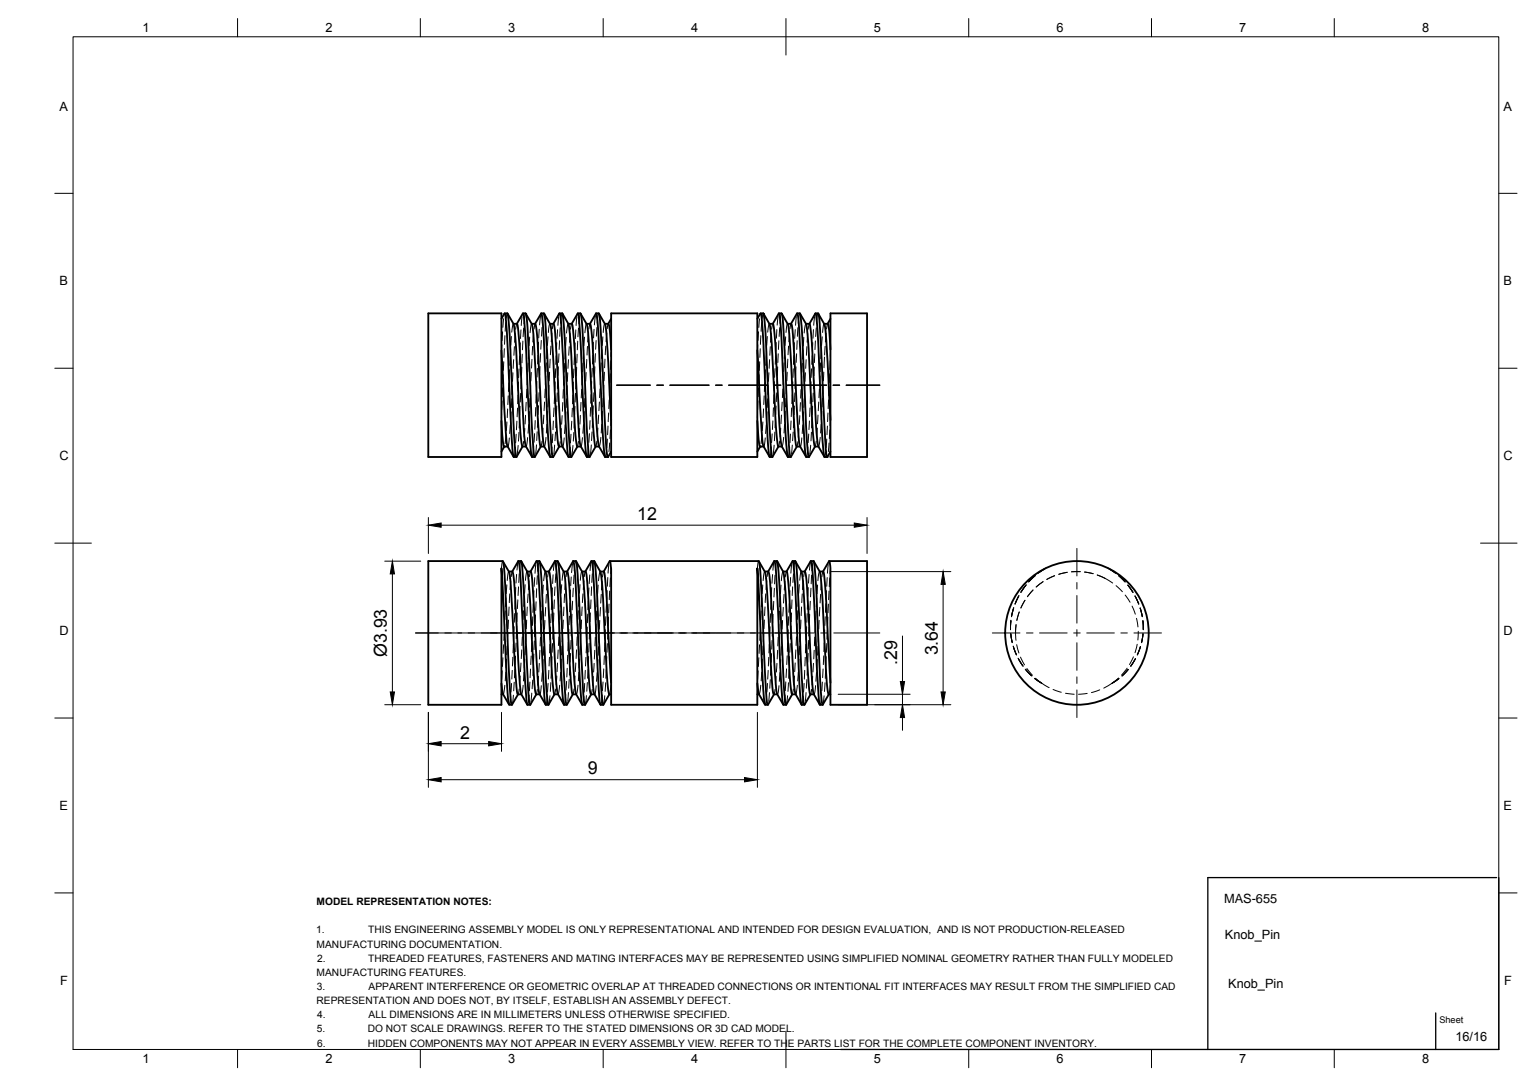
ISO-10303-21;
HEADER;
FILE_DESCRIPTION((''),'2;1');
FILE_NAME('Knob_Pin.step','2026-10-09T11:34:15-07:00',(''),(''),'','','');
FILE_SCHEMA (('AUTOMOTIVE_DESIGN { 1 0 10303 214 3 1 1 }'));
ENDSEC;
DATA;
#10=MECHANICAL_DESIGN_GEOMETRIC_PRESENTATION_REPRESENTATION('',(#648),#117170);
#606=SHAPE_REPRESENTATION_RELATIONSHIP('SRR','None',#117261,#627) ;
#627=ADVANCED_BREP_SHAPE_REPRESENTATION('',(#669),#117169) ;
#648=STYLED_ITEM('',(#117355),#669) ;
#669=MANIFOLD_SOLID_BREP('Body1',#49077) ;
#770=FACE_BOUND('',#17019,.T.) ;
#771=FACE_BOUND('',#17020,.T.) ;
#772=FACE_BOUND('',#17021,.T.) ;
#1697=B_SPLINE_CURVE_WITH_KNOTS('',3,(#109203,#109204,#109205,#109206,#109207,
#109208,#109209,#109210,#109211,#109212,#109213,#109214,#109215,#109216,
#109217,#109218,#109219,#109220,#109221,#109222,#109223,#109224,#109225,
#109226,#109227,#109228,#109229,#109230,#109231,#109232,#109233,#109234,
#109235,#109236,#109237,#109238,#109239,#109240,#109241,#109242,#109243,
#109244,#109245,#109246,#109247,#109248,#109249,#109250,#109251,#109252,
#109253,#109254,#109255,#109256,#109257,#109258,#109259,#109260,#109261,
#109262,#109263,#109264,#109265,#109266,#109267,#109268,#109269,#109270,
#109271,#109272,#109273,#109274,#109275,#109276,#109277,#109278,#109279,
#109280,#109281,#109282),.UNSPECIFIED.,.F.,.F.,(4,2,2,2,2,2,2,2,2,2,2,2,
2,2,2,2,2,2,2,2,2,2,2,2,2,2,2,2,2,2,2,2,2,2,2,2,2,2,2,4),(-0.552593410761711,
-0.5520841033493,-0.543414800045841,-0.530981645331462,-0.515682120379995,
-0.489011851192856,-0.475791475211459,-0.469800228676837,-0.464823585052418,
-0.456758200675436,-0.446117862199597,-0.412190397885134,-0.396445377902817,
-0.387356530724998,-0.378534621106888,-0.364686037892163,-0.330083411853553,
-0.312869588553632,-0.306676202327231,-0.301718040883505,-0.293987276238174,
-0.28400901338443,-0.255540175710082,-0.235962621045616,-0.226122570338451,
-0.217486499647387,-0.205608163506685,-0.191376706596845,-0.162958816002947,
-0.149015686282994,-0.143020064395438,-0.137940493423511,-0.129517498871141,
-0.118194060456811,-0.0767579974893125,-0.0659012890372971,-0.0573052858902992,
-0.0467033580009995,-0.0196389999660062,-0.00261625130652141),
 .UNSPECIFIED.) ;
#1698=B_SPLINE_CURVE_WITH_KNOTS('',3,(#109285,#109286,#109287,#109288,#109289,
#109290,#109291,#109292,#109293,#109294,#109295,#109296,#109297,#109298,
#109299,#109300,#109301,#109302,#109303,#109304,#109305,#109306,#109307,
#109308,#109309,#109310,#109311,#109312,#109313,#109314,#109315,#109316,
#109317,#109318,#109319,#109320,#109321,#109322,#109323,#109324,#109325,
#109326,#109327,#109328,#109329,#109330,#109331,#109332),.UNSPECIFIED.,
 .F.,.F.,(4,2,2,2,2,2,2,2,2,2,2,2,2,2,2,2,2,2,2,2,2,2,2,4),(-1.74388914172831,
-1.74010158624316,-1.73533493491195,-1.69713014187374,-1.68355997429145,
-1.67194962285965,-1.66271393068178,-1.65106169492588,-1.61630518110585,
-1.58993773929061,-1.58306967342475,-1.57816077380394,-1.57132637085491,
-1.54363126039316,-1.51548297073149,-1.50527675750718,-1.49695811956463,
-1.48648723066268,-1.44858943711612,-1.42603340225277,-1.41932565863014,
-1.41457975898413,-1.40826951094876,-1.40009241220142),.UNSPECIFIED.) ;
#1699=B_SPLINE_CURVE_WITH_KNOTS('',3,(#109337,#109338,#109339,#109340,#109341,
#109342,#109343,#109344,#109345,#109346,#109347,#109348,#109349,#109350,
#109351,#109352,#109353,#109354,#109355,#109356,#109357,#109358,#109359,
#109360,#109361,#109362,#109363,#109364,#109365,#109366,#109367,#109368,
#109369,#109370,#109371,#109372,#109373,#109374,#109375,#109376,#109377,
#109378,#109379,#109380,#109381,#109382,#109383,#109384,#109385,#109386,
#109387,#109388,#109389,#109390,#109391,#109392,#109393,#109394,#109395,
#109396,#109397,#109398,#109399,#109400,#109401,#109402,#109403,#109404,
#109405,#109406,#109407,#109408,#109409,#109410,#109411,#109412,#109413,
#109414,#109415,#109416,#109417,#109418,#109419,#109420,#109421,#109422,
#109423,#109424,#109425,#109426,#109427,#109428,#109429,#109430,#109431,
#109432,#109433,#109434,#109435,#109436,#109437,#109438,#109439,#109440,
#109441,#109442,#109443,#109444,#109445,#109446,#109447,#109448,#109449,
#109450,#109451,#109452,#109453,#109454,#109455,#109456,#109457,#109458,
#109459,#109460,#109461,#109462,#109463,#109464,#109465,#109466,#109467,
#109468,#109469,#109470,#109471,#109472,#109473,#109474,#109475,#109476),
 .UNSPECIFIED.,.F.,.F.,(4,2,2,2,2,2,2,2,2,2,2,2,2,2,2,2,2,2,2,2,2,2,2,2,
2,2,2,2,2,2,2,2,2,2,2,2,2,2,2,2,2,2,2,2,2,2,2,2,2,2,2,2,2,2,2,2,2,2,2,2,
2,2,2,2,2,2,2,2,2,4),(-1.60819476001236,-1.60157151108133,-1.57374993060186,
-1.54333520918712,-1.5330944628995,-1.52455732114626,-1.51368106490473,
-1.48363670371605,-1.45716775914122,-1.45034362080875,-1.44544941240374,
-1.43858684897259,-1.40293109993587,-1.38660840131381,-1.37365915712381,
-1.36493247672918,-1.35557163070149,-1.33795142758038,-1.30177252657126,
-1.29363751094972,-1.28694201653805,-1.28204551297269,-1.27504505146196,
-1.24750286398903,-1.21793991752278,-1.20732165243159,-1.1987959811487,
-1.18816616116487,-1.1535726711856,-1.1305629468268,-1.12379029329879,-1.11889461776859,
-1.11197522743769,-1.08352620940999,-1.05355243311613,-1.04333196199694,
-1.03479173415174,-1.02388438639545,-0.996280762100526,-0.97622121148834,
-0.964282134908163,-0.958700667916607,-0.953524190525165,-0.944167265791223,
-0.930858282226715,-0.891097096141751,-0.88060265191729,-0.872078959293447,
-0.861328341297288,-0.836209324457884,-0.803362711467678,-0.796962241119135,
-0.792056336516214,-0.784839695546787,-0.775791460713609,-0.753103628892537,
-0.728807187779854,-0.717955013186807,-0.709422378254332,-0.699000038493792,
-0.687312334031512,-0.663447018063261,-0.64163726390635,-0.634488912403423,
-0.629581096095425,-0.622988562285989,-0.615033268711227,-0.580749247858517,
-0.561627829423672,-0.552593410761711),.UNSPECIFIED.) ;
#1700=B_SPLINE_CURVE_WITH_KNOTS('',3,(#109477,#109478,#109479,#109480,#109481,
#109482,#109483,#109484,#109485,#109486,#109487,#109488,#109489,#109490,
#109491,#109492,#109493,#109494,#109495,#109496,#109497,#109498,#109499,
#109500,#109501,#109502,#109503,#109504,#109505,#109506,#109507,#109508,
#109509,#109510,#109511,#109512,#109513,#109514,#109515,#109516,#109517,
#109518,#109519,#109520,#109521,#109522,#109523,#109524,#109525,#109526,
#109527,#109528,#109529,#109530,#109531,#109532,#109533,#109534,#109535,
#109536,#109537,#109538,#109539,#109540,#109541,#109542,#109543,#109544,
#109545,#109546,#109547,#109548,#109549,#109550,#109551,#109552,#109553,
#109554,#109555,#109556,#109557,#109558,#109559,#109560,#109561,#109562,
#109563,#109564,#109565,#109566,#109567,#109568,#109569,#109570,#109571,
#109572,#109573,#109574,#109575,#109576,#109577,#109578,#109579,#109580,
#109581,#109582,#109583,#109584,#109585,#109586,#109587,#109588,#109589,
#109590,#109591,#109592,#109593,#109594,#109595,#109596,#109597,#109598,
#109599,#109600,#109601,#109602,#109603,#109604,#109605,#109606,#109607,
#109608,#109609,#109610,#109611,#109612,#109613,#109614,#109615,#109616,
#109617,#109618,#109619,#109620),.UNSPECIFIED.,.F.,.F.,(4,2,2,2,2,2,2,2,
2,2,2,2,2,2,2,2,2,2,2,2,2,2,2,2,2,2,2,2,2,2,2,2,2,2,2,2,2,2,2,2,2,2,2,2,
2,2,2,2,2,2,2,2,2,2,2,2,2,2,2,2,2,2,2,2,2,2,2,2,2,2,2,4),(-1.40009241220142,
-1.39027892404271,-1.35652120621099,-1.3427890502387,-1.33390838723088,
-1.3246360693791,-1.30797596827838,-1.27140299931499,-1.26322847705518,
-1.25649865986203,-1.25154939614112,-1.24437689145958,-1.22365219794817,
-1.19905991057942,-1.18720625527165,-1.17667403901707,-1.16811126913231,
-1.15728955781264,-1.12451282687639,-1.09983755963236,-1.09322146021638,
-1.08831885826578,-1.08120958853904,-1.05752347272841,-1.03479351117752,
-1.02336848189861,-1.01311471325315,-1.00462167080781,-0.993887863487606,
-0.96170664133996,-0.936256142399075,-0.929732827025822,-0.924842413978316,
-0.917692992839221,-0.896900816749588,-0.872386852319312,-0.856044560452436,
-0.846845625567806,-0.838022804779289,-0.824388691598358,-0.790916712807407,
-0.772827844029858,-0.766460546761273,-0.761546789185446,-0.754262465407307,
-0.745092618908703,-0.721724376077324,-0.698241216394806,-0.687447507649216,
-0.678919154709546,-0.668453448578193,-0.640197040220508,-0.610392150786397,
-0.603605311475741,-0.598712180190372,-0.59181667254431,-0.58333495261135,
-0.563541826914644,-0.535576624556928,-0.524668307552705,-0.51613376685688,
-0.505929580557802,-0.476712978209925,-0.447172033827767,-0.440359701789513,
-0.435467268922646,-0.428599990352192,-0.406330629551592,-0.370984619119945,
-0.36043799547759,-0.351912666138791,-0.344447890118419),.UNSPECIFIED.) ;
#1701=B_SPLINE_CURVE_WITH_KNOTS('',3,(#109626,#109627,#109628,#109629,#109630,
#109631,#109632,#109633),.UNSPECIFIED.,.F.,.F.,(4,1,1,1,1,4),(21.9911559852233,
22.8773584072887,23.8489981895043,24.8206379717199,25.7922777539356,26.2282428538859),
 .UNSPECIFIED.) ;
#1702=B_SPLINE_CURVE_WITH_KNOTS('',3,(#109634,#109635,#109636,#109637,#109638,
#109639,#109640,#109641,#109642,#109643,#109644,#109645,#109646,#109647,
#109648,#109649,#109650,#109651,#109652,#109653,#109654,#109655,#109656,
#109657,#109658,#109659,#109660,#109661,#109662,#109663,#109664,#109665,
#109666,#109667,#109668,#109669,#109670,#109671,#109672,#109673,#109674,
#109675,#109676,#109677,#109678,#109679,#109680,#109681,#109682,#109683,
#109684,#109685,#109686,#109687),.UNSPECIFIED.,.F.,.F.,(4,2,2,2,2,2,2,2,
2,2,2,2,2,2,2,2,2,2,2,2,2,2,2,2,2,2,4),(-1.95189018697911,-1.94523075986396,
-1.93976018216148,-1.9350625880257,-1.92813522823441,-1.9002619203118,-1.86981700938258,
-1.8595676021692,-1.85103118055753,-1.8401664646119,-1.81373957993934,-1.79279860037804,
-1.78408227826745,-1.77705321706049,-1.77215613141574,-1.76560901647882,
-1.72998813070304,-1.71337217751185,-1.70027829875411,-1.69153273295096,
-1.68221230721063,-1.66491104766538,-1.62833238402752,-1.62016088599395,
-1.61344422315257,-1.60854836482265,-1.60819476001236),.UNSPECIFIED.) ;
#1703=B_SPLINE_CURVE_WITH_KNOTS('',3,(#109689,#109690,#109691,#109692,#109693,
#109694,#109695,#109696,#109697,#109698,#109699,#109700,#109701,#109702,
#109703,#109704,#109705,#109706,#109707,#109708,#109709,#109710,#109711,
#109712,#109713,#109714,#109715,#109716,#109717,#109718,#109719,#109720,
#109721,#109722,#109723,#109724,#109725,#109726,#109727,#109728,#109729,
#109730,#109731,#109732,#109733,#109734),.UNSPECIFIED.,.F.,.F.,(4,2,2,2,
2,2,2,2,2,2,2,2,2,2,2,2,2,2,2,2,2,2,4),(-0.344447890118419,-0.341211553818979,
-0.316491587765998,-0.284698969180093,-0.277510677721432,-0.272606774376936,
-0.266068464621561,-0.240741588803494,-0.208560897771362,-0.197819047043028,
-0.189289309551728,-0.178943542594523,-0.150329573893438,-0.120559673202142,
-0.113770569004943,-0.108877003813415,-0.101982213749196,-0.0784204016516493,
-0.0446107495584237,-0.0340010178915369,-0.0254774882305537,-0.0173105615643668,
-0.000450519194125924),.UNSPECIFIED.) ;
#1704=B_SPLINE_CURVE_WITH_KNOTS('',3,(#109735,#109736,#109737,#109738,#109739,
#109740,#109741,#109742,#109743),.UNSPECIFIED.,.F.,.F.,(4,1,1,1,1,1,4),
(21.9911530646648,22.3032518321267,23.2748916143424,24.246531396558,25.2181711787737,
26.1898109609893,26.2282189766792),.UNSPECIFIED.) ;
#1705=B_SPLINE_CURVE_WITH_KNOTS('',3,(#109749,#109750,#109751,#109752,#109753,
#109754,#109755,#109756,#109757,#109758,#109759,#109760,#109761,#109762,
#109763,#109764,#109765,#109766,#109767,#109768,#109769,#109770,#109771,
#109772,#109773,#109774,#109775,#109776,#109777,#109778,#109779,#109780,
#109781,#109782,#109783,#109784,#109785,#109786,#109787,#109788,#109789,
#109790,#109791,#109792,#109793,#109794,#109795,#109796,#109797,#109798,
#109799,#109800,#109801,#109802,#109803,#109804,#109805,#109806,#109807,
#109808,#109809,#109810,#109811,#109812,#109813,#109814,#109815,#109816,
#109817,#109818,#109819,#109820,#109821,#109822,#109823,#109824,#109825,
#109826,#109827,#109828,#109829,#109830,#109831,#109832,#109833,#109834,
#109835,#109836,#109837,#109838,#109839,#109840,#109841,#109842,#109843,
#109844,#109845,#109846,#109847,#109848,#109849,#109850,#109851,#109852,
#109853,#109854,#109855,#109856,#109857,#109858,#109859,#109860,#109861,
#109862,#109863,#109864,#109865,#109866),.UNSPECIFIED.,.F.,.F.,(4,3,3,3,
3,3,3,3,3,3,3,3,3,3,3,3,3,3,3,3,3,3,3,3,3,3,3,3,3,3,3,3,3,3,3,3,3,3,3,4),
(28.2743338823081,28.3918577636548,28.5096435278108,28.6278521981456,28.7071971005825,
28.8171687217528,28.9269585080325,29.0366468286716,29.1462735481556,29.255878446213,
29.3655761414453,29.4753179582527,29.5852551857474,29.6788368827982,29.7887989434638,
29.8985795120685,30.0082588307296,30.1178767771779,30.2274731446426,30.337162748593,
30.4468967050156,30.5568265477835,30.6504766650138,30.7603623692327,30.8700661842359,
30.9796685717358,31.0892095506955,31.1987290554581,31.3083425744435,31.4180007690804,
31.527856329468,31.6221164472294,31.733214795593,31.8431380171637,31.9529572746322,
32.0627121966772,32.1747599560424,32.2845548564219,32.39772904528,32.5109032341381),
 .UNSPECIFIED.) ;
#1706=B_SPLINE_CURVE_WITH_KNOTS('',3,(#109867,#109868,#109869,#109870,#109871,
#109872),.UNSPECIFIED.,.F.,.F.,(4,1,1,4),(26.2282428538859,26.7639175361512,
27.7355573183669,28.2743338823081),.UNSPECIFIED.) ;
#1707=B_SPLINE_CURVE_WITH_KNOTS('',3,(#109874,#109875,#109876,#109877,#109878,
#109879),.UNSPECIFIED.,.F.,.F.,(4,1,1,4),(26.2282189766792,27.161450743205,
28.1330905254206,28.2743338823081),.UNSPECIFIED.) ;
#1708=B_SPLINE_CURVE_WITH_KNOTS('',3,(#109880,#109881,#109882,#109883,#109884,
#109885,#109886,#109887,#109888,#109889,#109890,#109891,#109892,#109893,
#109894,#109895,#109896,#109897,#109898,#109899,#109900,#109901,#109902,
#109903,#109904,#109905,#109906,#109907,#109908,#109909,#109910,#109911,
#109912,#109913,#109914,#109915,#109916,#109917,#109918,#109919,#109920,
#109921,#109922,#109923,#109924,#109925,#109926,#109927,#109928,#109929,
#109930,#109931,#109932,#109933,#109934,#109935,#109936,#109937,#109938,
#109939,#109940,#109941,#109942,#109943,#109944,#109945,#109946,#109947,
#109948,#109949,#109950,#109951,#109952,#109953,#109954,#109955,#109956,
#109957,#109958,#109959,#109960,#109961,#109962,#109963,#109964,#109965,
#109966,#109967,#109968,#109969,#109970,#109971,#109972,#109973,#109974,
#109975,#109976,#109977,#109978,#109979),.UNSPECIFIED.,.F.,.F.,(4,2,2,2,
2,2,2,2,2,2,2,2,2,2,2,2,2,2,2,2,2,2,2,2,2,2,2,2,2,2,2,2,2,2,2,2,2,2,2,2,
2,2,2,2,2,2,2,2,2,4),(0.712378143918981,0.712379954064215,0.72117831390082,
0.734657145018622,0.752068558527762,0.785373251131307,0.792345568546191,
0.79723963207803,0.803953757521709,0.812122008433253,0.848675628910262,
0.866001748507462,0.875321640069418,0.884058766219068,0.89712011860944,
0.913671889982011,0.949516073360798,0.956030042968438,0.960925950122258,
0.967985280014148,0.976755452934728,0.997970755917627,1.02406159262653,
1.03490881969519,1.0434433464097,1.05370359091221,1.08319754493553,1.11210683471402,
1.11898020632238,1.12387379656926,1.13068482421711,1.13901971639607,1.15811611731338,
1.18714628278811,1.19805288514865,1.20658974636888,1.21680178599216,1.24639735813157,
1.27537558519748,1.28224247880753,1.28713538887,1.2939502869039,1.30229203079242,
1.32142061052155,1.35040203680972,1.36130945627684,1.36984608699719,1.38005675842585,
1.4095946811458,1.42435463577266),.UNSPECIFIED.) ;
#1709=B_SPLINE_CURVE_WITH_KNOTS('',3,(#109985,#109986,#109987,#109988,#109989,
#109990,#109991,#109992,#109993,#109994,#109995,#109996,#109997,#109998,
#109999,#110000,#110001,#110002,#110003,#110004,#110005,#110006,#110007,
#110008,#110009,#110010,#110011,#110012,#110013,#110014,#110015,#110016,
#110017,#110018,#110019,#110020,#110021,#110022,#110023,#110024,#110025,
#110026,#110027,#110028,#110029,#110030,#110031,#110032,#110033,#110034,
#110035,#110036,#110037,#110038,#110039,#110040,#110041,#110042,#110043,
#110044,#110045,#110046,#110047,#110048,#110049,#110050,#110051,#110052,
#110053,#110054,#110055,#110056,#110057,#110058,#110059,#110060,#110061,
#110062,#110063,#110064,#110065,#110066,#110067,#110068,#110069,#110070,
#110071,#110072,#110073,#110074,#110075,#110076,#110077,#110078),
 .UNSPECIFIED.,.F.,.F.,(4,3,3,3,3,3,3,3,3,3,3,3,3,3,3,3,3,3,3,3,3,3,3,3,
3,3,3,3,3,3,3,4),(10.3764047342417,10.4900645190595,10.5981563505387,10.7061539904157,
10.8140997864379,10.9220360039885,11.0300742467267,11.1381720731464,11.2464519829849,
11.2856830127838,11.3954831058327,11.5060464833154,11.6155542565773,11.7249978887657,
11.8344175025737,11.9458106583537,12.0553714468275,12.1676807862607,12.2799901256938,
12.3895641603662,12.5001557951459,12.6094282845871,12.7186338508099,12.8278130186388,
12.93943407363,13.0487513389406,13.1615242887721,13.2742972386037,13.3839155036222,
13.4933854860546,13.6027340815615,13.6618521794004),.UNSPECIFIED.) ;
#1710=B_SPLINE_CURVE_WITH_KNOTS('',3,(#110081,#110082,#110083,#110084,#110085,
#110086,#110087,#110088,#110089,#110090,#110091,#110092,#110093,#110094,
#110095,#110096,#110097,#110098,#110099,#110100,#110101,#110102,#110103,
#110104,#110105,#110106,#110107,#110108,#110109,#110110,#110111,#110112,
#110113,#110114,#110115,#110116,#110117,#110118,#110119,#110120,#110121,
#110122,#110123,#110124,#110125,#110126,#110127,#110128,#110129,#110130,
#110131,#110132,#110133,#110134,#110135,#110136,#110137,#110138,#110139,
#110140),.UNSPECIFIED.,.F.,.F.,(4,2,2,2,2,2,2,2,2,2,2,2,2,2,2,2,2,2,2,2,
2,2,2,2,2,2,2,2,2,4),(-6.33424724009888,-6.3305869177302,-6.32541614156915,
-6.30776597142003,-6.28525261227357,-6.27314356015186,-6.2633690855282,
-6.25704102834557,-6.25075796634079,-6.24130885212152,-6.2018848898745,
-6.17573635588415,-6.17042441658865,-6.16711907831754,-6.16370428441967,
-6.15775527423043,-6.13753220062291,-6.11997163190395,-6.09800360015442,
-6.09050748347225,-6.08506535512531,-6.07923638089268,-6.06962378328271,
-6.02913105778434,-6.01429072948881,-6.00777656269078,-6.00256469572425,
-5.99938374041717,-5.99604989891884,-5.99053971230419),.UNSPECIFIED.) ;
#1711=B_SPLINE_CURVE_WITH_KNOTS('',3,(#110146,#110147,#110148,#110149,#110150,
#110151,#110152,#110153,#110154,#110155,#110156,#110157,#110158,#110159,
#110160,#110161,#110162,#110163,#110164,#110165,#110166,#110167,#110168,
#110169,#110170,#110171,#110172,#110173,#110174,#110175,#110176,#110177,
#110178,#110179,#110180,#110181,#110182,#110183,#110184,#110185,#110186,
#110187,#110188,#110189,#110190,#110191,#110192,#110193,#110194,#110195,
#110196,#110197,#110198,#110199,#110200,#110201,#110202,#110203,#110204,
#110205,#110206,#110207,#110208,#110209,#110210,#110211,#110212,#110213,
#110214,#110215,#110216,#110217,#110218,#110219,#110220,#110221,#110222,
#110223,#110224,#110225,#110226,#110227,#110228,#110229,#110230,#110231,
#110232,#110233,#110234,#110235,#110236,#110237,#110238,#110239,#110240,
#110241,#110242,#110243,#110244,#110245,#110246,#110247,#110248,#110249,
#110250,#110251,#110252,#110253,#110254,#110255,#110256,#110257),
 .UNSPECIFIED.,.F.,.F.,(4,2,2,2,2,2,2,2,2,2,2,2,2,2,2,2,2,2,2,2,2,2,2,2,
2,2,2,2,2,2,2,2,2,2,2,2,2,2,2,2,2,2,2,2,2,2,2,2,2,2,2,2,2,2,2,4),(-0.712477051017104,
-0.692802655493847,-0.683772920129568,-0.677945641814678,-0.672243058678314,
-0.663900351001329,-0.630604780701155,-0.603779896817934,-0.597758211996828,
-0.594319329048754,-0.59103022263903,-0.585743272187226,-0.560611083704649,
-0.525331213931128,-0.51649143220176,-0.510699465027105,-0.504968120500479,
-0.49646209662495,-0.469169926483107,-0.436335484292804,-0.430512931507663,
-0.427114820016612,-0.42379348225532,-0.418345458607985,-0.411507449451325,
-0.39559713149191,-0.357518717259878,-0.349022553353028,-0.343864348052536,
-0.338176905527992,-0.329923428023697,-0.30068061415273,-0.268790936312498,
-0.2632130787766,-0.25986516831537,-0.256495374779357,-0.250812807680856,
-0.227712274654564,-0.190747755479028,-0.182106619482357,-0.176350235475083,
-0.170583038913043,-0.161882552302035,-0.13811727285328,-0.102004110348754,
-0.0962660030206231,-0.0928851028491788,-0.0895501348445353,-0.0840301566912476,
-0.0606491320262799,-0.0405891786089123,-0.0211129520942058,-0.0137273297259265,
-0.00825233034605935,-0.00423882998995977,-0.000487560506064013),
 .UNSPECIFIED.) ;
#1712=B_SPLINE_CURVE_WITH_KNOTS('',3,(#110258,#110259,#110260,#110261,#110262,
#110263,#110264,#110265,#110266,#110267,#110268,#110269,#110270,#110271,
#110272,#110273,#110274,#110275,#110276,#110277,#110278,#110279,#110280,
#110281,#110282,#110283,#110284,#110285,#110286,#110287,#110288,#110289,
#110290,#110291,#110292,#110293,#110294,#110295,#110296,#110297,#110298,
#110299,#110300,#110301,#110302,#110303,#110304,#110305,#110306,#110307,
#110308,#110309,#110310,#110311,#110312,#110313,#110314,#110315),
 .UNSPECIFIED.,.F.,.F.,(4,3,3,3,3,3,3,3,3,3,3,3,3,3,3,3,3,3,3,4),(13.6618521794004,
13.7711169148501,13.88037702439,13.9897475868547,14.0991785591997,14.2088043877141,
14.2686043515136,14.3782655527654,14.4888462917227,14.5982089574048,14.7075055716608,
14.8167765076852,14.9283102468698,15.0377199986809,15.1503157315523,15.2629114644236,
15.3810391917761,15.4988692888196,15.6162446022961,15.7079632675443),
 .UNSPECIFIED.) ;
#1713=B_SPLINE_CURVE_WITH_KNOTS('',3,(#110316,#110317,#110318,#110319,#110320,
#110321,#110322,#110323,#110324,#110325,#110326,#110327,#110328,#110329,
#110330,#110331,#110332,#110333,#110334,#110335,#110336,#110337,#110338,
#110339,#110340,#110341,#110342,#110343,#110344,#110345,#110346,#110347,
#110348,#110349,#110350,#110351,#110352,#110353,#110354,#110355,#110356,
#110357,#110358,#110359,#110360,#110361,#110362,#110363,#110364,#110365,
#110366,#110367,#110368,#110369,#110370,#110371,#110372,#110373,#110374,
#110375,#110376,#110377,#110378,#110379,#110380,#110381,#110382,#110383,
#110384,#110385,#110386,#110387,#110388,#110389,#110390,#110391,#110392,
#110393,#110394,#110395,#110396,#110397,#110398,#110399,#110400,#110401,
#110402,#110403,#110404,#110405,#110406,#110407,#110408,#110409,#110410,
#110411,#110412,#110413,#110414,#110415,#110416,#110417,#110418,#110419,
#110420,#110421,#110422,#110423,#110424,#110425,#110426,#110427,#110428,
#110429,#110430,#110431,#110432,#110433,#110434,#110435,#110436,#110437,
#110438,#110439,#110440,#110441,#110442,#110443,#110444,#110445,#110446,
#110447,#110448,#110449,#110450,#110451,#110452,#110453,#110454,#110455,
#110456,#110457,#110458,#110459,#110460,#110461,#110462,#110463,#110464,
#110465,#110466,#110467,#110468,#110469,#110470,#110471,#110472,#110473,
#110474,#110475),.UNSPECIFIED.,.F.,.F.,(4,2,2,2,2,2,2,2,2,2,2,2,2,2,2,2,
2,2,2,2,2,2,2,2,2,2,2,2,2,2,2,2,2,2,2,2,2,2,2,2,2,2,2,2,2,2,2,2,2,2,2,2,
2,2,2,2,2,2,2,2,2,2,2,2,2,2,2,2,2,2,2,2,2,2,2,2,2,2,2,4),(-5.99053971230419,
-5.99047461915376,-5.95863408749524,-5.92969933625071,-5.92114681247369,
-5.915382578984,-5.90955220244452,-5.90062838830993,-5.87701819018997,-5.85236394846719,
-5.84376533328685,-5.8373135536108,-5.83375945007048,-5.83052134715155,
-5.82542463673811,-5.80505229717849,-5.77693764917991,-5.76556984118265,
-5.75625855327928,-5.75035861651557,-5.7447229240835,-5.73656342255167,
-5.69603857832968,-5.68123878905728,-5.67467388255143,-5.66938441896224,
-5.6660855631516,-5.66265149068689,-5.65661618350724,-5.62976488185456,
-5.59655621591346,-5.58823493236518,-5.58255620616837,-5.57744225437469,
-5.56910919109571,-5.52835464098746,-5.51380877876097,-5.50732381078696,
-5.50209177678022,-5.49882403274683,-5.49538334870154,-5.48934624246608,
-5.46251397712469,-5.42923993509709,-5.4209137181702,-5.41521229709611,
-5.41006365996861,-5.40163487145359,-5.36317618148174,-5.34096910239947,
-5.33541870518404,-5.33207440806664,-5.32869619298517,-5.32297321551596,
-5.29245413663171,-5.26226599070794,-5.2539712036158,-5.24827681786533,
-5.24243800882422,-5.23334744843942,-5.20142115753318,-5.17348278738021,
-5.16816968985747,-5.16487583020783,-5.16144680644824,-5.15546548539489,
-5.12795602433186,-5.0955345838297,-5.08709883194831,-5.0813835504828,-5.07558361949721,
-5.06668208643157,-5.03201451159366,-5.00644599200698,-5.00112565663733,
-4.99783192271362,-4.99440511132734,-4.98843793496379,-4.95371727216649,
-4.9350521817335),.UNSPECIFIED.) ;
#1714=B_SPLINE_CURVE_WITH_KNOTS('',3,(#110480,#110481,#110482,#110483,#110484,
#110485,#110486,#110487,#110488,#110489,#110490,#110491,#110492,#110493,
#110494,#110495,#110496,#110497,#110498,#110499,#110500,#110501,#110502,
#110503,#110504,#110505,#110506,#110507,#110508,#110509,#110510,#110511,
#110512,#110513,#110514,#110515,#110516,#110517,#110518,#110519,#110520,
#110521,#110522,#110523,#110524,#110525,#110526,#110527,#110528,#110529,
#110530,#110531,#110532,#110533,#110534,#110535,#110536,#110537,#110538,
#110539,#110540,#110541,#110542,#110543,#110544,#110545,#110546,#110547,
#110548,#110549,#110550,#110551,#110552,#110553,#110554,#110555,#110556,
#110557,#110558,#110559,#110560,#110561,#110562,#110563,#110564,#110565,
#110566,#110567,#110568,#110569,#110570,#110571,#110572,#110573,#110574,
#110575,#110576,#110577,#110578,#110579,#110580,#110581,#110582,#110583,
#110584,#110585,#110586,#110587,#110588,#110589,#110590,#110591,#110592,
#110593,#110594,#110595,#110596,#110597,#110598,#110599,#110600,#110601,
#110602,#110603,#110604,#110605,#110606,#110607,#110608,#110609,#110610,
#110611,#110612,#110613,#110614,#110615,#110616,#110617,#110618,#110619,
#110620,#110621,#110622,#110623,#110624,#110625,#110626,#110627,#110628,
#110629,#110630,#110631,#110632,#110633,#110634,#110635,#110636,#110637,
#110638,#110639,#110640,#110641,#110642,#110643),.UNSPECIFIED.,.F.,.F.,
(4,2,2,2,2,2,2,2,2,2,2,2,2,2,2,2,2,2,2,2,2,2,2,2,2,2,2,2,2,2,2,2,2,2,2,
2,2,2,2,2,2,2,2,2,2,2,2,2,2,2,2,2,2,2,2,2,2,2,2,2,2,2,2,2,2,2,2,2,2,2,2,
2,2,2,2,2,2,2,2,2,2,4),(-1.76818356378078,-1.76666210863979,-1.76335874747055,
-1.75993953124951,-1.75401304730633,-1.7261788047067,-1.69407326476353,
-1.68558675228945,-1.67985926096194,-1.67406390562458,-1.66520393482846,
-1.63010226962174,-1.60561277861248,-1.59990800700045,-1.59653437101539,
-1.5931919816856,-1.58763889989772,-1.55556687777865,-1.52720892284277,
-1.5186289076951,-1.5128845673421,-1.50710766903938,-1.49834858149115,-1.46232917555678,
-1.43790919774604,-1.43254040047344,-1.42923527159702,-1.42581814563762,
-1.41990211094776,-1.39200096337258,-1.37007954259637,-1.36001416862498,
-1.35150084664892,-1.34576835606398,-1.33997808174755,-1.33114681658688,
-1.29576757956943,-1.27111086695335,-1.2656091204,-1.26227714970592,-1.2588918091262,
-1.25313088766896,-1.22300159181825,-1.19232624188739,-1.1840951061917,
-1.17841204248402,-1.17325077710014,-1.16473296027604,-1.12680166285061,
-1.11081344178922,-1.10395627554512,-1.09849739707728,-1.09517412141265,
-1.09177887023573,-1.08596972878113,-1.05647958053428,-1.02710225847862,
-1.01799436632724,-1.0121526839847,-1.0064613458708,-0.998182189048535,
-0.968373423054622,-0.937279229744221,-0.931613068231424,-0.928247271935606,
-0.924897021545374,-0.919306345738125,-0.912225740972987,-0.89530601260113,
-0.859324571674764,-0.850563538847296,-0.844786048445886,-0.839041581798305,
-0.830462374491692,-0.802250305773277,-0.76995397365888,-0.764423281997596,
-0.761085322112715,-0.75770626514405,-0.751976387823087,-0.72590084049544,
-0.712477051017104),.UNSPECIFIED.) ;
#1715=B_SPLINE_CURVE_WITH_KNOTS('',3,(#110644,#110645,#110646,#110647,#110648,
#110649,#110650,#110651,#110652,#110653,#110654,#110655,#110656,#110657,
#110658,#110659,#110660,#110661,#110662,#110663,#110664,#110665,#110666,
#110667,#110668,#110669,#110670,#110671,#110672,#110673,#110674,#110675,
#110676,#110677,#110678,#110679,#110680,#110681,#110682,#110683,#110684,
#110685,#110686,#110687,#110688,#110689,#110690,#110691,#110692,#110693,
#110694,#110695,#110696,#110697,#110698,#110699,#110700,#110701,#110702,
#110703,#110704,#110705,#110706,#110707,#110708,#110709,#110710,#110711,
#110712,#110713,#110714,#110715,#110716,#110717,#110718,#110719,#110720,
#110721,#110722,#110723,#110724,#110725,#110726,#110727,#110728,#110729,
#110730,#110731,#110732,#110733,#110734,#110735,#110736,#110737,#110738,
#110739,#110740,#110741,#110742,#110743,#110744,#110745,#110746,#110747,
#110748,#110749,#110750,#110751,#110752,#110753,#110754,#110755,#110756,
#110757,#110758,#110759,#110760,#110761,#110762,#110763,#110764,#110765,
#110766,#110767,#110768,#110769,#110770,#110771,#110772,#110773,#110774,
#110775,#110776,#110777,#110778,#110779,#110780,#110781,#110782,#110783,
#110784,#110785,#110786,#110787,#110788,#110789,#110790,#110791,#110792,
#110793,#110794,#110795,#110796,#110797,#110798,#110799,#110800,#110801,
#110802,#110803,#110804,#110805,#110806,#110807,#110808,#110809),
 .UNSPECIFIED.,.F.,.F.,(4,2,2,2,2,2,2,2,2,2,2,2,2,2,2,2,2,2,2,2,2,2,2,2,
2,2,2,2,2,2,2,2,2,2,2,2,2,2,2,2,2,2,2,2,2,2,2,2,2,2,2,2,2,2,2,2,2,2,2,2,
2,2,2,2,2,2,2,2,2,2,2,2,2,2,2,2,2,2,2,2,2,2,4),(-4.9350521817335,-4.92924063431001,
-4.92044239877843,-4.91465940528696,-4.90892351641425,-4.90038456224455,
-4.86264847290703,-4.84658277607218,-4.8397074909766,-4.83423827443184,
-4.83091341750573,-4.82752198218248,-4.82172782759203,-4.79203898950566,
-4.77112106687337,-4.76130259504078,-4.75294376002215,-4.74724004938001,
-4.74141951950012,-4.73241737215319,-4.69892832381971,-4.6728214363707,
-4.66728213436687,-4.66394329293773,-4.66056834654829,-4.65485352521452,
-4.62426640486569,-4.59411722047284,-4.58582595290027,-4.58013430875787,
-4.57429882728677,-4.56521504374047,-4.53318283650538,-4.50616750618709,
-4.50042352036627,-4.49704259355698,-4.49411219504707,-4.48902115662041,
-4.46748769556528,-4.44020461262813,-4.42900107160256,-4.41979655965162,
-4.41393804178965,-4.40832682243432,-4.40017938091833,-4.35965849168015,
-4.34482640449425,-4.3382611866649,-4.33297664176318,-4.32968873335359,
-4.32625095373141,-4.32023086486532,-4.29342481673317,-4.26015236585617,
-4.25181104174667,-4.24611029313889,-4.24028564120251,-4.23126189696331,
-4.19807637418412,-4.17162792408406,-4.16613041753203,-4.16280001841052,
-4.15941534758802,-4.15365421993062,-4.12354614187762,-4.09338197576611,
-4.08491495060093,-4.0791920594429,-4.07339477872434,-4.06451836754818,
-4.02959475019793,-4.00439138334853,-3.99899340105477,-3.99568309549955,
-3.99227477190073,-3.98639863391994,-3.95113205383628,-3.92694774181241,
-3.91819047658281,-3.91241514624073,-3.90667266451009,-3.89809625365554,
-3.87952612660362),.UNSPECIFIED.) ;
#1716=B_SPLINE_CURVE_WITH_KNOTS('',3,(#110815,#110816,#110817,#110818,#110819,
#110820,#110821,#110822,#110823,#110824,#110825,#110826,#110827,#110828,
#110829,#110830,#110831,#110832,#110833,#110834,#110835,#110836,#110837,
#110838,#110839,#110840,#110841,#110842,#110843,#110844,#110845,#110846,
#110847,#110848,#110849,#110850,#110851,#110852,#110853,#110854,#110855,
#110856,#110857,#110858,#110859,#110860,#110861,#110862,#110863,#110864,
#110865,#110866,#110867,#110868,#110869,#110870,#110871,#110872,#110873,
#110874,#110875,#110876,#110877,#110878,#110879,#110880,#110881,#110882,
#110883,#110884,#110885,#110886,#110887,#110888,#110889,#110890,#110891,
#110892,#110893,#110894,#110895,#110896,#110897,#110898,#110899,#110900,
#110901,#110902,#110903,#110904,#110905,#110906,#110907,#110908,#110909,
#110910,#110911,#110912,#110913,#110914,#110915,#110916),.UNSPECIFIED.,
 .F.,.F.,(4,2,2,2,2,2,2,2,2,2,2,2,2,2,2,2,2,2,2,2,2,2,2,2,2,2,2,2,2,2,2,
2,2,2,2,2,2,2,2,2,2,2,2,2,2,2,2,2,2,2,4),(-0.712560310195096,-0.696927543742108,
-0.664393756377226,-0.658308473226922,-0.654856627884361,-0.65157642714292,
-0.646335858781874,-0.619824553094956,-0.586138170659426,-0.577149854410368,
-0.571330128691633,-0.565621274854638,-0.557243683240465,-0.52515271781851,
-0.496938482436241,-0.491060214402507,-0.487650558070128,-0.484338641962742,
-0.478937515505729,-0.453679571810099,-0.41884006969134,-0.409954338268172,
-0.404153524304069,-0.398428867282295,-0.389962470359715,-0.360362849023259,
-0.329508722091577,-0.3238157222087,-0.320444136084627,-0.317098690632935,
-0.311532565593602,-0.287426221779339,-0.251506631916206,-0.242737154611523,
-0.236957694377381,-0.231213934171252,-0.222641014264426,-0.194841718838807,
-0.16199081489796,-0.156522544681182,-0.153197069938858,-0.149803377221981,
-0.144003303274408,-0.124995580033334,-0.0846985680180007,-0.075785096394773,
-0.0699791943610914,-0.0642589396352745,-0.0558170987592085,-0.0233685145724937,
-0.000486898249177208),.UNSPECIFIED.) ;
#1717=B_SPLINE_CURVE_WITH_KNOTS('',3,(#110917,#110918,#110919,#110920,#110921,
#110922,#110923,#110924,#110925,#110926,#110927,#110928,#110929,#110930,
#110931,#110932,#110933,#110934,#110935,#110936,#110937,#110938,#110939,
#110940,#110941,#110942,#110943,#110944,#110945,#110946,#110947,#110948,
#110949,#110950,#110951,#110952,#110953,#110954,#110955,#110956,#110957,
#110958,#110959,#110960,#110961,#110962,#110963,#110964,#110965,#110966,
#110967,#110968,#110969,#110970,#110971,#110972,#110973,#110974),
 .UNSPECIFIED.,.F.,.F.,(4,2,2,2,2,2,2,2,2,2,2,2,2,2,2,2,2,2,2,2,2,2,2,2,
2,2,2,2,4),(-2.11192746243384,-2.10365836072938,-2.10032748721145,-2.09739905319525,
-2.09395618783264,-2.0879135511067,-2.0618322929545,-2.05345777211631,-2.02888579184874,
-2.0200732276697,-2.01428663417168,-2.00855143726169,-2.00002183872159,
-1.96218415944355,-1.94615428816371,-1.93928708674953,-1.93382235705294,
-1.93049802943554,-1.92710441440501,-1.92130264175917,-1.89170157783663,
-1.86141009373834,-1.85279580594553,-1.84704537799896,-1.84127518605679,
-1.83255223671774,-1.79622972800035,-1.77202226703003,-1.76818356378078),
 .UNSPECIFIED.) ;
#1718=B_SPLINE_CURVE_WITH_KNOTS('',3,(#110975,#110976,#110977,#110978,#110979,
#110980,#110981,#110982,#110983,#110984,#110985,#110986,#110987,#110988,
#110989,#110990,#110991,#110992,#110993,#110994,#110995,#110996,#110997,
#110998,#110999,#111000,#111001,#111002,#111003,#111004,#111005,#111006,
#111007,#111008,#111009,#111010,#111011,#111012,#111013,#111014,#111015,
#111016,#111017,#111018,#111019,#111020,#111021,#111022,#111023,#111024,
#111025,#111026,#111027,#111028,#111029,#111030,#111031,#111032,#111033,
#111034,#111035,#111036,#111037,#111038,#111039,#111040,#111041,#111042,
#111043,#111044,#111045,#111046,#111047,#111048,#111049,#111050,#111051,
#111052,#111053,#111054,#111055,#111056,#111057,#111058,#111059,#111060,
#111061,#111062,#111063,#111064,#111065,#111066,#111067,#111068,#111069,
#111070,#111071,#111072,#111073,#111074,#111075,#111076,#111077,#111078,
#111079,#111080,#111081,#111082,#111083,#111084,#111085,#111086,#111087,
#111088,#111089,#111090,#111091,#111092,#111093,#111094,#111095,#111096,
#111097,#111098,#111099,#111100,#111101,#111102,#111103,#111104,#111105,
#111106,#111107,#111108,#111109,#111110,#111111,#111112,#111113,#111114,
#111115,#111116,#111117,#111118,#111119,#111120,#111121,#111122,#111123,
#111124,#111125,#111126,#111127,#111128,#111129,#111130,#111131,#111132,
#111133,#111134,#111135,#111136,#111137,#111138,#111139,#111140),
 .UNSPECIFIED.,.F.,.F.,(4,2,2,2,2,2,2,2,2,2,2,2,2,2,2,2,2,2,2,2,2,2,2,2,
2,2,2,2,2,2,2,2,2,2,2,2,2,2,2,2,2,2,2,2,2,2,2,2,2,2,2,2,2,2,2,2,2,2,2,2,
2,2,2,2,2,2,2,2,2,2,2,2,2,2,2,2,2,2,2,2,2,2,4),(-3.87952612660362,-3.86062568452188,
-3.84442601515873,-3.83751797114886,-3.83202943311297,-3.82870086247565,
-3.82531413862114,-3.81954303164399,-3.78955091772268,-3.7592912808188,
-3.7508234548549,-3.7451004257672,-3.73930331754311,-3.73042781496521,-3.6954957738308,
-3.67029896598693,-3.66490124106473,-3.661590990245,-3.65818262332641,-3.65230620949632,
-3.62412515274316,-3.5920459744581,-3.58367034575224,-3.57796362120538,
-3.57214672886548,-3.56316448102137,-3.52941186474604,-3.50302060509746,
-3.49774346021087,-3.49445708491337,-3.49101745410518,-3.48498800924908,
-3.4581560142016,-3.42487758809319,-3.41655914447765,-3.41086247708157,
-3.40503275253428,-3.39598133942955,-3.37005366899035,-3.34641573350646,
-3.33797448860644,-3.33161560747389,-3.32810952227488,-3.32490391984474,
-3.319885547723,-3.30123149955326,-3.27984059566937,-3.26413966465563,-3.25247692687625,
-3.24615940815198,-3.24063956259222,-3.23357099957884,-3.21846630144393,
-3.18244798671489,-3.16773500197394,-3.16305806015763,-3.15987674157065,
-3.15621982427784,-3.14908667546599,-3.11755196697434,-3.09237116509003,
-3.08332238548082,-3.07749299246945,-3.07179562991928,-3.06347434404492,
-3.03018176236825,-3.0033288158175,-2.99730399144291,-2.99386520520512,
-2.99057789569833,-2.98529675938854,-2.95999947546801,-2.92493103033546,
-2.91607175218247,-2.91027740623184,-2.90455134575136,-2.89606802224394,
-2.88604934852181,-2.86432142289227,-2.83600264401299,-2.83013743101675,
-2.82673127717738,-2.82399026850942),.UNSPECIFIED.) ;
#1719=B_SPLINE_CURVE_WITH_KNOTS('',3,(#111145,#111146,#111147,#111148,#111149,
#111150,#111151,#111152,#111153,#111154,#111155,#111156,#111157,#111158,
#111159,#111160,#111161,#111162,#111163,#111164,#111165,#111166,#111167,
#111168,#111169,#111170,#111171,#111172,#111173,#111174,#111175,#111176,
#111177,#111178,#111179,#111180,#111181,#111182,#111183,#111184,#111185,
#111186,#111187,#111188,#111189,#111190,#111191,#111192,#111193,#111194,
#111195,#111196,#111197,#111198,#111199,#111200,#111201,#111202,#111203,
#111204,#111205,#111206,#111207,#111208,#111209,#111210,#111211,#111212,
#111213,#111214,#111215,#111216,#111217,#111218,#111219,#111220,#111221,
#111222,#111223,#111224,#111225,#111226,#111227,#111228,#111229,#111230,
#111231,#111232,#111233,#111234,#111235,#111236,#111237,#111238,#111239,
#111240,#111241,#111242,#111243,#111244,#111245,#111246,#111247,#111248,
#111249,#111250,#111251,#111252,#111253,#111254,#111255,#111256,#111257,
#111258,#111259,#111260,#111261,#111262,#111263,#111264,#111265,#111266,
#111267,#111268,#111269,#111270,#111271,#111272,#111273,#111274,#111275,
#111276,#111277,#111278,#111279,#111280,#111281,#111282,#111283,#111284,
#111285,#111286,#111287,#111288,#111289,#111290,#111291,#111292,#111293,
#111294,#111295,#111296,#111297,#111298,#111299,#111300,#111301,#111302,
#111303,#111304,#111305,#111306),.UNSPECIFIED.,.F.,.F.,(4,2,2,2,2,2,2,2,
2,2,2,2,2,2,2,2,2,2,2,2,2,2,2,2,2,2,2,2,2,2,2,2,2,2,2,2,2,2,2,2,2,2,2,2,
2,2,2,2,2,2,2,2,2,2,2,2,2,2,2,2,2,2,2,2,2,2,2,2,2,2,2,2,2,2,2,2,2,2,2,2,
4),(-1.76829897325153,-1.75460392163481,-1.74611762918806,-1.74038984818434,
-1.73459384330885,-1.72573211997339,-1.69063835242174,-1.66555260637465,
-1.66015783335173,-1.65684745379245,-1.65343685955817,-1.64755255118024,
-1.61942449203402,-1.58730905211199,-1.57892593974264,-1.57321674186153,
-1.56739935178262,-1.55842050573739,-1.52459629337172,-1.49855014186046,
-1.49312071830056,-1.48980351553656,-1.48640137667395,-1.48055862353011,
-1.44508483627295,-1.42100550335908,-1.41226161927158,-1.40648741653162,
-1.40074025349759,-1.39214525728931,-1.35479931095745,-1.33167692340998,
-1.32614191424939,-1.32280313343559,-1.31942525780903,-1.31370051849044,
-1.28319005419036,-1.25297473638803,-1.24467823110622,-1.23898392491907,
-1.2331463645208,-1.22406051627092,-1.19201073794918,-1.16500246036131,
-1.15925695802786,-1.15587482220384,-1.15253997060442,-1.14702422880595,
-1.11462133444451,-1.08535977678247,-1.07730603012133,-1.07165280267554,
-1.06575282050299,-1.0563353966255,-1.02697771227102,-0.998098672414146,
-0.992262514355829,-0.988861694626336,-0.985543012286294,-0.98010727071304,
-0.973289789452838,-0.957461674297307,-0.919211833316843,-0.9107404145102,
-0.905586573923107,-0.899895806731126,-0.891620532261262,-0.861899771527197,
-0.830682611318693,-0.825029788918696,-0.821666696298092,-0.81831367031811,
-0.812709721714768,-0.805606455171284,-0.788590340785238,-0.752797444912451,
-0.74401456566953,-0.738233003103442,-0.732492126687357,-0.723933250484363,
-0.712560310195096),.UNSPECIFIED.) ;
#1720=B_SPLINE_CURVE_WITH_KNOTS('',3,(#111307,#111308,#111309,#111310,#111311,
#111312,#111313,#111314,#111315,#111316,#111317,#111318,#111319,#111320,
#111321,#111322,#111323,#111324,#111325,#111326,#111327,#111328,#111329,
#111330,#111331,#111332,#111333,#111334,#111335,#111336,#111337,#111338,
#111339,#111340,#111341,#111342,#111343,#111344,#111345,#111346,#111347,
#111348,#111349,#111350,#111351,#111352,#111353,#111354,#111355,#111356,
#111357,#111358,#111359,#111360,#111361,#111362,#111363,#111364,#111365,
#111366,#111367,#111368,#111369,#111370,#111371,#111372,#111373,#111374,
#111375,#111376,#111377,#111378,#111379,#111380,#111381,#111382,#111383,
#111384,#111385,#111386,#111387,#111388,#111389,#111390,#111391,#111392,
#111393,#111394,#111395,#111396,#111397,#111398,#111399,#111400,#111401,
#111402,#111403,#111404,#111405,#111406,#111407,#111408,#111409,#111410,
#111411,#111412,#111413,#111414,#111415,#111416,#111417,#111418,#111419,
#111420,#111421,#111422,#111423,#111424,#111425,#111426,#111427,#111428,
#111429,#111430,#111431,#111432,#111433,#111434,#111435,#111436,#111437,
#111438,#111439,#111440,#111441,#111442,#111443,#111444,#111445,#111446,
#111447,#111448,#111449,#111450,#111451,#111452,#111453,#111454,#111455,
#111456,#111457,#111458,#111459,#111460,#111461,#111462,#111463,#111464,
#111465,#111466,#111467,#111468),.UNSPECIFIED.,.F.,.F.,(4,2,2,2,2,2,2,2,
2,2,2,2,2,2,2,2,2,2,2,2,2,2,2,2,2,2,2,2,2,2,2,2,2,2,2,2,2,2,2,2,2,2,2,2,
2,2,2,2,2,2,2,2,2,2,2,2,2,2,2,2,2,2,2,2,2,2,2,2,2,2,2,2,2,2,2,2,2,2,2,2,
4),(-2.82399026850942,-2.82341890687629,-2.81801132306273,-2.79253919112659,
-2.75799980550302,-2.74908808182721,-2.74328402892283,-2.73756618862353,
-2.72912918990773,-2.69797579532232,-2.66887982531938,-2.66305181517914,
-2.65965324196555,-2.65633440963625,-2.65089498863588,-2.64407077120943,
-2.62821305750453,-2.59003369288838,-2.58155457207929,-2.57640052065259,
-2.57071300498161,-2.56244987304937,-2.53296005495871,-2.50142691207352,
-2.4958106358921,-2.49245568167594,-2.48909648100377,-2.48345980855283,
-2.456974533545,-2.42415276243805,-2.41510756047844,-2.40927853774309,-2.40358016901041,
-2.39525485839727,-2.36196088688736,-2.33510849801988,-2.3290854951205,
-2.32564692129078,-2.32235904506188,-2.31707583991493,-2.31051361107425,
-2.29569318899404,-2.25516488421965,-2.24702024182607,-2.24140908540174,
-2.23554906495507,-2.2263388407737,-2.21512519677322,-2.18779871835891,
-2.16629308856763,-2.16120069777036,-2.15826981502894,-2.15488845048444,
-2.14914429800924,-2.14179899911136,-2.12372082221965,-2.08990279265047,
-2.08092730936326,-2.07511128899889,-2.06940285603707,-2.06101995164008,
-2.02889883164275,-2.00075263773878,-1.99486799858886,-1.99145772928818,
-1.98814835522146,-1.98275634484835,-1.95771002465056,-1.922592074612,-1.91373719119365,
-1.90794342607117,-1.90221626915163,-1.89372810144114,-1.86159458878002,
-1.83377362628468,-1.82784069540986,-1.82442048288859,-1.82111879767998,
-1.81576572041569,-1.79171101232918,-1.76831699902817),.UNSPECIFIED.) ;
#1721=B_SPLINE_CURVE_WITH_KNOTS('',3,(#111474,#111475,#111476,#111477,#111478,
#111479,#111480,#111481,#111482,#111483,#111484,#111485,#111486,#111487,
#111488,#111489,#111490,#111491,#111492,#111493,#111494,#111495,#111496,
#111497,#111498,#111499,#111500,#111501,#111502,#111503,#111504,#111505,
#111506,#111507,#111508,#111509,#111510,#111511,#111512,#111513,#111514,
#111515,#111516,#111517,#111518,#111519,#111520,#111521,#111522,#111523,
#111524,#111525,#111526,#111527,#111528,#111529,#111530,#111531,#111532,
#111533,#111534,#111535,#111536,#111537,#111538,#111539,#111540,#111541,
#111542,#111543,#111544,#111545,#111546,#111547,#111548,#111549,#111550,
#111551,#111552,#111553,#111554,#111555,#111556,#111557,#111558,#111559,
#111560,#111561,#111562,#111563,#111564,#111565,#111566,#111567,#111568,
#111569,#111570,#111571,#111572,#111573,#111574,#111575,#111576,#111577,
#111578,#111579,#111580,#111581,#111582,#111583,#111584,#111585,#111586,
#111587,#111588),.UNSPECIFIED.,.F.,.F.,(4,3,3,3,3,3,3,3,3,3,3,3,3,3,3,3,
3,3,3,3,3,3,3,3,3,3,3,3,3,3,3,3,3,3,3,3,3,3,4),(40.8407044969695,40.9778004485257,
41.1148964000819,41.2245591175802,41.3351396670066,41.4445029598726,41.5537998679094,
41.6630707648349,41.7746039518741,41.8840128460614,41.9966081795266,42.1092035129918,
42.2188516823835,42.3294340503233,42.4387834441433,42.5480667322124,42.6573243083354,
42.768870887727,42.8782673433037,42.9908889846027,43.1035106259017,43.2130813463413,
43.3236733954001,43.4329445134416,43.5421494364015,43.6513286879563,43.7629509506701,
43.8722700890464,43.985043913929,44.0978177388117,44.2076327245732,44.3172547150156,
44.4267684933025,44.536214279915,44.6456322030823,44.7551374325598,44.8646820423166,
44.9744233938719,45.0774317841423),.UNSPECIFIED.) ;
#1722=B_SPLINE_CURVE_WITH_KNOTS('',3,(#111589,#111590,#111591,#111592,#111593,
#111594,#111595,#111596,#111597,#111598,#111599,#111600,#111601,#111602,
#111603,#111604,#111605,#111606,#111607,#111608,#111609,#111610,#111611,
#111612,#111613,#111614,#111615,#111616,#111617,#111618,#111619,#111620,
#111621,#111622,#111623,#111624,#111625,#111626,#111627,#111628,#111629,
#111630,#111631,#111632,#111633,#111634,#111635,#111636,#111637,#111638,
#111639,#111640,#111641,#111642,#111643,#111644),.UNSPECIFIED.,.F.,.F.,
(4,2,2,2,2,2,2,2,2,2,2,2,2,2,2,2,2,2,2,2,2,2,2,2,2,2,2,4),(-2.11228412499268,
-2.09589069751274,-2.08616970041209,-2.08037589962005,-2.07463269380149,
-2.0688595433906,-2.06011197044276,-2.0235776218593,-2.0069774997407,-1.99997283546138,
-1.99442747362915,-1.99108766548718,-1.98771301743009,-1.98200388162584,
-1.95133971005555,-1.92190326785172,-1.91330335441766,-1.90755485784521,
-1.9017807039189,-1.8930396354663,-1.85687418159894,-1.83256461598671,-1.82719981502227,
-1.82389505434892,-1.82047618598876,-1.81455254885302,-1.78669711134918,
-1.76829897325153),.UNSPECIFIED.) ;
#1723=B_SPLINE_CURVE_WITH_KNOTS('',3,(#111645,#111646,#111647,#111648,#111649,
#111650,#111651,#111652,#111653,#111654,#111655,#111656,#111657,#111658,
#111659,#111660,#111661,#111662,#111663,#111664,#111665,#111666,#111667,
#111668,#111669,#111670,#111671,#111672,#111673,#111674,#111675,#111676,
#111677,#111678,#111679,#111680,#111681,#111682,#111683,#111684,#111685,
#111686,#111687,#111688,#111689,#111690,#111691,#111692,#111693,#111694,
#111695,#111696,#111697,#111698,#111699,#111700,#111701,#111702,#111703,
#111704,#111705,#111706,#111707,#111708,#111709,#111710,#111711,#111712,
#111713,#111714,#111715,#111716,#111717,#111718,#111719,#111720,#111721,
#111722,#111723,#111724,#111725,#111726,#111727,#111728,#111729,#111730,
#111731,#111732,#111733,#111734,#111735,#111736,#111737,#111738,#111739,
#111740,#111741,#111742,#111743,#111744,#111745,#111746,#111747,#111748,
#111749,#111750,#111751,#111752,#111753,#111754,#111755,#111756,#111757,
#111758,#111759,#111760,#111761,#111762,#111763,#111764,#111765,#111766,
#111767,#111768,#111769,#111770,#111771,#111772,#111773,#111774,#111775,
#111776,#111777,#111778,#111779,#111780,#111781,#111782,#111783,#111784,
#111785,#111786,#111787,#111788,#111789,#111790,#111791,#111792,#111793,
#111794,#111795,#111796,#111797,#111798,#111799,#111800,#111801,#111802,
#111803,#111804,#111805,#111806,#111807,#111808),.UNSPECIFIED.,.F.,.F.,
(4,2,2,2,2,2,2,2,2,2,2,2,2,2,2,2,2,2,2,2,2,2,2,2,2,2,2,2,2,2,2,2,2,2,2,
2,2,2,2,2,2,2,2,2,2,2,2,2,2,2,2,2,2,2,2,2,2,2,2,2,2,2,2,2,2,2,2,2,2,2,2,
2,2,2,2,2,2,2,2,2,2,4),(-1.76831699902817,-1.75518964805716,-1.7464939967529,
-1.74072931780407,-1.73497502618634,-1.72633662398727,-1.69475416514867,
-1.66661632486612,-1.66073017475442,-1.65731947814099,-1.65401004875575,
-1.64861855660536,-1.62359288966011,-1.58844479684806,-1.57959255588087,
-1.57379900488342,-1.56807094121945,-1.55957925089772,-1.52737702425792,
-1.49966150675423,-1.49370975209278,-1.49028556586819,-1.48698678312783,
-1.48164844322083,-1.45555171790032,-1.42160028807763,-1.41263445446714,
-1.40681995276556,-1.40110964628147,-1.39271766668299,-1.36054972024335,
-1.33248078779257,-1.32658507794482,-1.32317237433183,-1.31986434892612,
-1.3144804660512,-1.28966197107827,-1.25422061233062,-1.24539843861857,
-1.23961009702442,-1.23387658404469,-1.22535624893443,-1.19575074172621,
-1.16505376690443,-1.15934496571757,-1.15597044251782,-1.15262831875543,
-1.14707799948981,-1.12489509543687,-1.08629569001683,-1.07787376642098,
-1.07272788441997,-1.06702884083304,-1.05870563516865,-1.02540582083539,
-0.998547257588233,-0.992520046801463,-0.989080304812647,-0.985794181702154,
-0.980516494618136,-0.97396305824982,-0.959175820696547,-0.918536689606294,
-0.910405236709954,-0.904797500956223,-0.898936632101549,-0.889715679414612,
-0.878483193532081,-0.851054163825655,-0.829681793148376,-0.824590238282511,
-0.821659670394674,-0.818276870565965,-0.812530368884856,-0.805182019449805,
-0.787095435655023,-0.753274574776637,-0.744294657821547,-0.738475350004387,
-0.732763203677629,-0.724373493863662,-0.712529018801462),.UNSPECIFIED.) ;
#1724=B_SPLINE_CURVE_WITH_KNOTS('',3,(#111816,#111817,#111818,#111819,#111820,
#111821,#111822,#111823),.UNSPECIFIED.,.F.,.F.,(4,1,1,1,1,4),(-27.2059139020381,
-26.2342741198224,-25.2626343376068,-24.2909945553912,-23.3193547731755,
-22.9423101900986),.UNSPECIFIED.) ;
#1725=B_SPLINE_CURVE_WITH_KNOTS('',3,(#111825,#111826,#111827,#111828,#111829,
#111830,#111831,#111832,#111833,#111834,#111835,#111836,#111837,#111838,
#111839,#111840,#111841,#111842,#111843,#111844,#111845,#111846,#111847,
#111848,#111849,#111850,#111851,#111852,#111853,#111854,#111855,#111856,
#111857,#111858,#111859,#111860,#111861,#111862,#111863,#111864,#111865,
#111866,#111867,#111868,#111869,#111870,#111871,#111872,#111873,#111874,
#111875,#111876,#111877,#111878,#111879,#111880,#111881,#111882,#111883,
#111884,#111885,#111886,#111887,#111888,#111889,#111890,#111891,#111892,
#111893,#111894,#111895,#111896,#111897,#111898,#111899,#111900,#111901,
#111902,#111903,#111904,#111905,#111906,#111907,#111908,#111909,#111910,
#111911,#111912,#111913,#111914,#111915,#111916,#111917,#111918,#111919,
#111920,#111921,#111922,#111923,#111924,#111925,#111926,#111927,#111928,
#111929,#111930,#111931,#111932,#111933,#111934,#111935,#111936,#111937,
#111938,#111939,#111940,#111941,#111942,#111943,#111944,#111945,#111946,
#111947,#111948,#111949,#111950,#111951,#111952,#111953,#111954,#111955,
#111956,#111957,#111958,#111959,#111960,#111961,#111962,#111963,#111964,
#111965,#111966,#111967,#111968,#111969,#111970,#111971,#111972,#111973,
#111974,#111975,#111976,#111977,#111978,#111979,#111980,#111981,#111982,
#111983,#111984,#111985,#111986,#111987,#111988,#111989,#111990,#111991,
#111992,#111993,#111994,#111995,#111996,#111997,#111998,#111999,#112000,
#112001,#112002,#112003,#112004,#112005,#112006,#112007,#112008,#112009,
#112010,#112011,#112012,#112013,#112014,#112015,#112016,#112017),
 .UNSPECIFIED.,.F.,.F.,(4,3,3,3,3,3,3,3,3,3,3,3,3,3,3,3,3,3,3,3,3,3,3,3,
3,3,3,3,3,3,3,3,3,3,3,3,3,3,3,3,3,3,3,3,3,3,3,3,3,3,3,3,3,3,3,3,3,3,3,3,
3,3,3,3,4),(-22.9423049617331,-22.8359146756665,-22.7294985856963,-22.6229461677493,
-22.5163198701347,-22.4094937864604,-22.3477149909599,-22.241991690464,
-22.133752130249,-22.0282970330834,-21.9229015138189,-21.8175302025545,
-21.7071664541019,-21.6016731308017,-21.4961119262998,-21.3903887822451,
-21.3760752087442,-21.270344951488,-21.1621062608681,-21.0566434209101,
-20.95123988815,-20.8458603053796,-20.7355040856669,-20.6300019344483,-20.5244317166851,
-20.4186993582769,-20.4044354265286,-20.2987232088165,-20.1904822632535,
-20.0850383121632,-19.9796539285277,-19.8742937220325,-19.7639192026026,
-19.6584367694276,-19.5528863693,-19.4471738307262,-19.4327956443129,-19.327075538132,
-19.2188355786277,-19.1133834865874,-19.0079908919881,-18.9026224187124,
-18.7922557795586,-18.6867650370827,-18.581206320842,-18.4754855147286,
-18.4611558620973,-18.355436078419,-18.2471960786018,-18.1417442669779,
-18.0363519363068,-17.9309837099735,-17.8206168024505,-17.7151262611044,
-17.609567729898,-17.5038470846879,-17.4895160798816,-17.3853086147757,
-17.2812326981936,-17.1772506712568,-17.0733250028991,-16.9693644080451,
-16.8653929900671,-16.7612777660331,-16.6591196549165),.UNSPECIFIED.) ;
#1726=B_SPLINE_CURVE_WITH_KNOTS('',3,(#112019,#112020,#112021,#112022,#112023,
#112024,#112025,#112026,#112027,#112028,#112029,#112030,#112031,#112032,
#112033,#112034,#112035,#112036,#112037,#112038,#112039,#112040,#112041,
#112042,#112043,#112044,#112045,#112046,#112047,#112048,#112049,#112050,
#112051,#112052,#112053,#112054,#112055,#112056,#112057,#112058,#112059,
#112060,#112061,#112062,#112063,#112064,#112065,#112066,#112067,#112068,
#112069,#112070,#112071,#112072,#112073,#112074,#112075,#112076,#112077,
#112078,#112079,#112080,#112081,#112082,#112083,#112084,#112085,#112086,
#112087,#112088,#112089,#112090,#112091,#112092,#112093,#112094,#112095,
#112096,#112097,#112098,#112099,#112100,#112101,#112102,#112103,#112104,
#112105,#112106,#112107,#112108,#112109,#112110,#112111,#112112,#112113,
#112114,#112115,#112116,#112117,#112118,#112119,#112120,#112121,#112122,
#112123,#112124,#112125,#112126,#112127,#112128,#112129,#112130,#112131,
#112132,#112133,#112134,#112135,#112136,#112137,#112138,#112139,#112140,
#112141,#112142,#112143,#112144,#112145,#112146,#112147,#112148,#112149,
#112150,#112151,#112152,#112153,#112154,#112155,#112156,#112157,#112158,
#112159,#112160,#112161,#112162,#112163,#112164,#112165,#112166,#112167,
#112168,#112169,#112170,#112171,#112172,#112173,#112174,#112175,#112176,
#112177,#112178,#112179,#112180,#112181,#112182,#112183,#112184,#112185,
#112186,#112187,#112188,#112189,#112190,#112191,#112192,#112193,#112194,
#112195,#112196,#112197,#112198,#112199,#112200,#112201,#112202,#112203,
#112204,#112205,#112206,#112207,#112208,#112209,#112210,#112211),
 .UNSPECIFIED.,.F.,.F.,(4,3,3,3,3,3,3,3,3,3,3,3,3,3,3,3,3,3,3,3,3,3,3,3,
3,3,3,3,3,3,3,3,3,3,3,3,3,3,3,3,3,3,3,3,3,3,3,3,3,3,3,3,3,3,3,3,3,3,3,3,
3,3,3,3,4),(-16.6591196545535,-16.517876297666,-16.4121571817512,-16.3039170984636,
-16.1984659993176,-16.0930743956811,-15.98770690971,-15.8773393111451,-15.7718495350374,
-15.6662917769805,-15.5605719107464,-15.5462365154503,-15.4405175111735,
-15.3322774139311,-15.2268264264337,-15.1214349341175,-15.0160675589399,
-14.9056998525136,-14.8002101845372,-14.6946525335813,-14.5889327722318,
-14.5745967332347,-14.4688778255767,-14.360637716257,-14.2551868315348,
-14.1497954439831,-14.044428175381,-13.9340603692905,-13.8285708111944,
-13.7230132711611,-13.6172936214372,-13.602956951019,-13.4972380492425,
-13.3889979391876,-13.2835470569139,-13.1781556705346,-13.0727884018306,
-12.9624205935738,-12.856931032194,-12.7513734877815,-12.6456538321663,
-12.6313171688034,-12.5255981556858,-12.4173580595486,-12.3119070683704,
-12.2065155742917,-12.1011481992669,-11.9907804960971,-11.8852908330562,
-11.7797331886823,-11.6740134361877,-11.6596773865878,-11.5539582688639,
-11.4457181858024,-11.3402670859034,-11.2348754819066,-11.1295079959672,
-11.0191403980684,-10.9136506229712,-10.8080928662617,-10.7023730018402,
-10.6880376043721,-10.5637109854946,-10.4405584833869,-10.3759343476556),
 .UNSPECIFIED.) ;
#1727=B_SPLINE_CURVE_WITH_KNOTS('',3,(#112213,#112214,#112215,#112216,#112217,
#112218,#112219,#112220,#112221,#112222,#112223,#112224,#112225,#112226,
#112227,#112228,#112229,#112230,#112231,#112232,#112233,#112234,#112235,
#112236,#112237,#112238,#112239,#112240,#112241,#112242,#112243,#112244,
#112245,#112246,#112247,#112248,#112249,#112250,#112251,#112252,#112253,
#112254,#112255,#112256,#112257,#112258,#112259,#112260,#112261,#112262,
#112263,#112264,#112265,#112266,#112267,#112268,#112269,#112270,#112271,
#112272,#112273,#112274,#112275,#112276,#112277,#112278,#112279,#112280,
#112281,#112282,#112283,#112284,#112285,#112286,#112287,#112288,#112289,
#112290,#112291,#112292,#112293,#112294,#112295,#112296,#112297,#112298,
#112299,#112300,#112301,#112302,#112303,#112304,#112305,#112306,#112307,
#112308,#112309,#112310,#112311,#112312,#112313,#112314,#112315,#112316,
#112317,#112318,#112319,#112320,#112321,#112322,#112323,#112324,#112325,
#112326,#112327,#112328,#112329,#112330,#112331,#112332,#112333,#112334,
#112335,#112336,#112337,#112338,#112339,#112340,#112341,#112342,#112343,
#112344,#112345,#112346,#112347,#112348,#112349,#112350,#112351,#112352,
#112353,#112354,#112355,#112356,#112357,#112358,#112359,#112360,#112361,
#112362,#112363,#112364,#112365,#112366,#112367,#112368,#112369,#112370,
#112371,#112372,#112373,#112374,#112375,#112376,#112377,#112378,#112379,
#112380,#112381,#112382,#112383,#112384,#112385,#112386,#112387,#112388,
#112389,#112390,#112391,#112392,#112393,#112394,#112395,#112396,#112397,
#112398,#112399,#112400,#112401,#112402,#112403,#112404,#112405,#112406,
#112407,#112408),.UNSPECIFIED.,.F.,.F.,(4,3,3,3,3,3,3,3,3,3,3,3,3,3,3,3,
3,3,3,3,3,3,3,3,3,3,3,3,3,3,3,3,3,3,3,3,3,3,3,3,3,3,3,3,3,3,3,3,3,3,3,3,
3,3,3,3,3,3,3,3,3,3,3,3,3,4),(-10.375934347374,-10.270818228235,-10.1657261742581,
-10.0606224775472,-9.95540604281518,-9.8501222535424,-9.74466686480985,
-9.71639782215646,-9.61067792744562,-9.50243794150752,-9.39698608366202,
-9.2915937308619,-9.18622550645682,-9.07585863982782,-8.97036816048045,
-8.86480971195451,-8.75908917797183,-8.74475803994082,-8.63903798481663,
-8.5307980189302,-8.42534594814427,-8.31995336372064,-8.2145848895582,-8.10421823159994,
-7.99872746061479,-7.89316870635468,-7.78744784909512,-7.77311825772517,
-7.66740644868325,-7.55916545203653,-7.45372167107659,-7.34833736890122,
-7.24297715532693,-7.13260248537258,-7.02711982401829,-6.92156911959377,
-6.81585617164976,-6.80147847550953,-6.69574689772163,-6.58750837216816,
-6.48204498251401,-6.37664118662987,-6.27126162688296,-6.16090589348569,
-6.05540447971091,-5.94983524539449,-5.84410420992605,-5.82983869329388,
-5.72411630668951,-5.6158766322381,-5.51042191551005,-5.40502657837274,
-5.29965525121858,-5.18929116618349,-5.0837973325642,-4.97823544750672,
-4.87251138793772,-4.85819891107823,-4.75396818259709,-4.64987162623521,
-4.54587159887065,-4.44193058968034,-4.33797426762636,-4.23400853536007,
-4.12994521022668,-4.09274904045468),.UNSPECIFIED.) ;
#1728=B_SPLINE_CURVE_WITH_KNOTS('',3,(#112410,#112411,#112412,#112413,#112414,
#112415,#112416,#112417,#112418,#112419,#112420,#112421,#112422,#112423,
#112424,#112425,#112426,#112427,#112428,#112429,#112430,#112431,#112432,
#112433,#112434,#112435,#112436,#112437,#112438,#112439,#112440,#112441,
#112442,#112443,#112444,#112445,#112446,#112447,#112448,#112449,#112450,
#112451,#112452,#112453,#112454,#112455,#112456,#112457,#112458,#112459,
#112460,#112461,#112462,#112463,#112464,#112465,#112466,#112467,#112468,
#112469,#112470),.UNSPECIFIED.,.F.,.F.,(4,3,3,3,3,3,3,3,3,3,3,3,3,3,3,3,
3,3,3,3,4),(-4.09274904019429,-3.94994251714104,-3.88655912886259,-3.78069844242293,
-3.67247605545093,-3.5668839769559,-3.46135201338902,-3.35584502036394,
-3.24561360193469,-3.13998805631316,-3.03429594813686,-2.92844465404552,
-2.91491934664694,-2.80970101248105,-2.70571134479635,-2.60181252142057,
-2.49796692460674,-2.39176836178501,-2.28786550058172,-2.18051908695078,
-2.07317267331984),.UNSPECIFIED.) ;
#1729=B_SPLINE_CURVE_WITH_KNOTS('',3,(#112472,#112473,#112474,#112475),
 .UNSPECIFIED.,.F.,.F.,(4,4),(-0.0367203712850908,0.),.UNSPECIFIED.) ;
#1730=B_SPLINE_CURVE_WITH_KNOTS('',3,(#112479,#112480,#112481,#112482,#112483),
 .UNSPECIFIED.,.F.,.F.,(4,1,4),(0.,0.971639782215629,1.12201628671538),
 .UNSPECIFIED.) ;
#1731=B_SPLINE_CURVE_WITH_KNOTS('',3,(#112485,#112486,#112487,#112488,#112489,
#112490,#112491,#112492,#112493,#112494,#112495,#112496,#112497,#112498,
#112499,#112500,#112501,#112502,#112503,#112504,#112505,#112506,#112507,
#112508,#112509,#112510,#112511,#112512,#112513,#112514,#112515,#112516,
#112517,#112518,#112519,#112520,#112521,#112522,#112523,#112524,#112525,
#112526,#112527,#112528,#112529,#112530,#112531,#112532,#112533,#112534,
#112535,#112536,#112537,#112538,#112539,#112540,#112541,#112542,#112543,
#112544,#112545,#112546,#112547,#112548,#112549,#112550,#112551,#112552,
#112553,#112554,#112555,#112556,#112557,#112558,#112559,#112560,#112561,
#112562,#112563,#112564,#112565,#112566,#112567,#112568,#112569,#112570,
#112571,#112572,#112573,#112574,#112575,#112576,#112577,#112578,#112579,
#112580,#112581,#112582,#112583,#112584,#112585,#112586,#112587,#112588,
#112589,#112590,#112591,#112592,#112593,#112594,#112595,#112596,#112597,
#112598,#112599,#112600,#112601,#112602,#112603,#112604,#112605,#112606,
#112607,#112608,#112609,#112610,#112611,#112612,#112613,#112614,#112615,
#112616,#112617,#112618,#112619,#112620,#112621,#112622,#112623,#112624,
#112625,#112626,#112627,#112628,#112629,#112630,#112631,#112632,#112633,
#112634,#112635,#112636,#112637,#112638,#112639,#112640,#112641,#112642,
#112643,#112644,#112645,#112646,#112647,#112648,#112649,#112650,#112651,
#112652,#112653,#112654,#112655,#112656,#112657,#112658,#112659,#112660,
#112661,#112662,#112663,#112664,#112665,#112666,#112667,#112668,#112669,
#112670,#112671,#112672,#112673,#112674,#112675,#112676,#112677),
 .UNSPECIFIED.,.F.,.F.,(4,3,3,3,3,3,3,3,3,3,3,3,3,3,3,3,3,3,3,3,3,3,3,3,
3,3,3,3,3,3,3,3,3,3,3,3,3,3,3,3,3,3,3,3,3,3,3,3,3,3,3,3,3,3,3,3,3,3,3,3,
3,3,3,3,4),(1.12201628671538,1.22573351984078,1.32934711813555,1.4328950730314,
1.53641527935953,1.64001495378494,1.74365071550474,1.84746877012718,1.94327956443127,
2.0489757773739,2.15721872353302,2.2626385001509,2.36799578538946,2.47332604534675,
2.58372437067179,2.68917019510039,2.79468174011294,2.90035256690749,2.91491934664691,
3.02076955040777,3.12899324771462,3.23458096412644,3.34011084293479,3.44561802516486,
3.55585330108929,3.66148470545172,3.76718462728308,3.8730464282202,3.88655912886256,
3.9922114528047,4.10045988508888,4.20584197472517,4.31116394383356,4.41646128846482,
4.52689569411816,4.6323148743042,4.73780194400129,4.84345148339452,4.8581989110782,
4.96392221077202,5.07216177108725,5.17761686744958,5.28301238591223,5.38838369637743,
5.49874744560654,5.60424076812202,5.70980197184468,5.81552511513283,5.82983869329384,
5.93556895048034,6.04380764110898,6.14927048100083,6.254674013696,6.36005359640275,
6.47040981617943,6.575911967338,6.68148218504262,6.78721454339403,6.80147847550949,
6.90810451976517,7.01457261073179,7.12090179489442,7.22714857804156,7.3333604972507,
7.40520159389494),.UNSPECIFIED.) ;
#1732=B_SPLINE_CURVE_WITH_KNOTS('',3,(#112679,#112680,#112681,#112682,#112683,
#112684,#112685,#112686,#112687,#112688,#112689,#112690,#112691,#112692,
#112693,#112694,#112695,#112696,#112697,#112698,#112699,#112700,#112701,
#112702,#112703,#112704,#112705,#112706,#112707,#112708,#112709,#112710,
#112711,#112712,#112713,#112714,#112715,#112716,#112717,#112718,#112719,
#112720,#112721,#112722,#112723,#112724,#112725,#112726,#112727,#112728,
#112729,#112730,#112731,#112732,#112733,#112734,#112735,#112736,#112737,
#112738,#112739,#112740,#112741,#112742,#112743,#112744,#112745,#112746,
#112747,#112748,#112749,#112750,#112751,#112752,#112753,#112754,#112755,
#112756,#112757,#112758,#112759,#112760,#112761,#112762,#112763,#112764,
#112765,#112766,#112767,#112768,#112769,#112770,#112771,#112772,#112773,
#112774,#112775,#112776,#112777,#112778,#112779,#112780,#112781,#112782,
#112783,#112784,#112785,#112786,#112787,#112788,#112789,#112790,#112791,
#112792,#112793,#112794,#112795,#112796,#112797,#112798,#112799,#112800,
#112801,#112802,#112803,#112804,#112805,#112806,#112807,#112808,#112809,
#112810,#112811,#112812,#112813,#112814,#112815,#112816,#112817,#112818,
#112819,#112820,#112821,#112822,#112823,#112824,#112825,#112826,#112827,
#112828,#112829,#112830,#112831,#112832,#112833,#112834,#112835,#112836,
#112837,#112838,#112839,#112840,#112841,#112842,#112843,#112844,#112845,
#112846,#112847,#112848,#112849,#112850,#112851,#112852,#112853,#112854,
#112855,#112856,#112857,#112858,#112859,#112860,#112861,#112862,#112863,
#112864,#112865,#112866,#112867,#112868,#112869,#112870,#112871,#112872,
#112873,#112874),.UNSPECIFIED.,.F.,.F.,(4,3,3,3,3,3,3,3,3,3,3,3,3,3,3,3,
3,3,3,3,3,3,3,3,3,3,3,3,3,3,3,3,3,3,3,3,3,3,3,3,3,3,3,3,3,3,3,3,3,3,3,3,
3,3,3,3,3,3,3,3,3,3,3,3,3,4),(7.4052015942302,7.52274829518333,7.64076688448783,
7.75933378391934,7.77311825772513,7.87883836383028,7.98707832334409,8.0925304153057,
8.19792300982544,8.3032914830209,8.41365812225087,8.51914886464601,8.6247075808057,
8.73042838683844,8.74475803994077,8.85047782361075,8.95871782342896,9.06416963504312,
9.16956196570429,9.27493019202703,9.38529709955938,9.49078764089399,9.59634617208882,
9.7020668172867,9.71639782215641,9.82211609691572,9.93035628534776,10.0358065127374,
10.1411972357971,10.2465638338936,10.3569322765132,10.4624211569032,10.5679780173793,
10.6736969896783,10.6880376043721,10.7937567202753,10.9019968035643,11.0074479026982,
11.1128395063224,11.2182069922812,11.3285745908578,11.4340643669531,11.5396221249977,
11.6453419912194,11.6596773865877,11.7653963908656,11.8736364881078,11.9790874756063,
12.0844789679236,12.1898463431023,12.3002140495275,12.405703717505,12.511261368462,
12.6169811298125,12.6313171688033,12.7370360764623,12.8452761857819,12.9507270705053,
13.0561184580582,13.1614857266615,13.2718535327509,13.3773430908484,13.4829006308829,
13.5886202806081,13.602956951019,13.6883869010745),.UNSPECIFIED.) ;
#1733=B_SPLINE_CURVE_WITH_KNOTS('',3,(#112876,#112877,#112878,#112879,#112880,
#112881,#112882,#112883,#112884,#112885,#112886,#112887,#112888,#112889,
#112890,#112891,#112892,#112893,#112894,#112895,#112896,#112897,#112898,
#112899,#112900,#112901,#112902,#112903,#112904,#112905,#112906,#112907,
#112908,#112909,#112910,#112911,#112912,#112913,#112914,#112915,#112916,
#112917,#112918,#112919,#112920,#112921,#112922,#112923,#112924,#112925,
#112926,#112927,#112928,#112929,#112930,#112931,#112932,#112933,#112934,
#112935,#112936,#112937,#112938,#112939,#112940,#112941,#112942,#112943,
#112944,#112945,#112946,#112947,#112948,#112949,#112950,#112951,#112952,
#112953,#112954,#112955,#112956,#112957,#112958,#112959,#112960,#112961,
#112962,#112963,#112964,#112965,#112966,#112967,#112968,#112969,#112970,
#112971,#112972,#112973,#112974,#112975,#112976,#112977,#112978,#112979,
#112980,#112981,#112982,#112983,#112984,#112985,#112986,#112987,#112988,
#112989,#112990,#112991,#112992,#112993,#112994,#112995,#112996,#112997,
#112998,#112999,#113000,#113001,#113002,#113003,#113004,#113005,#113006,
#113007,#113008,#113009,#113010,#113011,#113012,#113013,#113014,#113015,
#113016,#113017,#113018,#113019,#113020,#113021,#113022,#113023,#113024,
#113025,#113026,#113027,#113028,#113029,#113030,#113031,#113032,#113033,
#113034,#113035,#113036,#113037,#113038,#113039,#113040,#113041,#113042,
#113043,#113044,#113045,#113046,#113047,#113048,#113049,#113050,#113051,
#113052,#113053,#113054,#113055,#113056,#113057,#113058,#113059,#113060,
#113061,#113062,#113063,#113064,#113065,#113066,#113067,#113068),
 .UNSPECIFIED.,.F.,.F.,(4,3,3,3,3,3,3,3,3,3,3,3,3,3,3,3,3,3,3,3,3,3,3,3,
3,3,3,3,3,3,3,3,3,3,3,3,3,3,3,3,3,3,3,3,3,3,3,3,3,3,3,3,3,3,3,3,3,3,3,3,
3,3,3,3,4),(13.6883869014638,13.7928966431387,13.8972545313542,14.0015295444517,
14.10575882162,14.2099794381379,14.3142930238784,14.4186584630941,14.5231928841024,
14.5745967332346,14.6803157463521,14.7885558424894,14.8940068336676,14.9993983277466,
15.1047657027714,15.2151334059411,15.3206230689822,15.4261807133564,15.5319004658512,
15.5462365154503,15.6519556331625,15.7601957162254,15.8656468161126,15.9710384200976,
16.0764059060253,16.1867735039355,16.292263279021,16.397821035719,16.5035409001291,
16.5178762976659,16.62359452377,16.7318347182839,16.8372849254186,16.9426756387808,
17.0480422377219,17.1584106982618,17.2638996058194,17.3694565025261,17.475175523565,
17.4895160798816,17.5952359745804,17.70347596052,17.8089278183545,17.9143201711438,
18.0196883955385,18.1300552621782,18.2355457415161,18.341104190033,18.4468247240073,
18.4611558620972,18.5668759171409,18.6751158830374,18.7805679537426,18.8859605380855,
18.9913290121675,19.1016956702039,19.2071864411105,19.3127451952932,19.4184660524764,
19.4327956443128,19.5414242479478,19.6498166849957,19.7580694756742,19.8661879885317,
19.9715722082541),.UNSPECIFIED.) ;
#1734=B_SPLINE_CURVE_WITH_KNOTS('',3,(#113070,#113071,#113072,#113073,#113074,
#113075,#113076,#113077,#113078,#113079,#113080,#113081,#113082,#113083,
#113084,#113085,#113086,#113087,#113088,#113089,#113090,#113091,#113092,
#113093,#113094,#113095,#113096,#113097,#113098,#113099,#113100,#113101,
#113102,#113103,#113104,#113105,#113106,#113107,#113108,#113109,#113110,
#113111,#113112,#113113,#113114,#113115,#113116,#113117,#113118,#113119,
#113120,#113121,#113122,#113123,#113124,#113125,#113126,#113127,#113128,
#113129,#113130,#113131,#113132,#113133,#113134,#113135,#113136,#113137,
#113138,#113139,#113140,#113141,#113142,#113143,#113144,#113145,#113146,
#113147,#113148,#113149,#113150,#113151,#113152,#113153,#113154,#113155,
#113156,#113157,#113158,#113159,#113160,#113161,#113162,#113163,#113164,
#113165,#113166,#113167,#113168,#113169,#113170,#113171,#113172,#113173,
#113174,#113175,#113176,#113177,#113178,#113179,#113180,#113181,#113182,
#113183,#113184,#113185,#113186,#113187,#113188,#113189,#113190,#113191,
#113192,#113193,#113194,#113195,#113196,#113197,#113198,#113199,#113200,
#113201,#113202,#113203,#113204,#113205,#113206,#113207,#113208,#113209,
#113210,#113211,#113212,#113213,#113214,#113215,#113216,#113217,#113218,
#113219,#113220,#113221,#113222,#113223,#113224,#113225,#113226),
 .UNSPECIFIED.,.F.,.F.,(4,3,3,3,3,3,3,3,3,3,3,3,3,3,3,3,3,3,3,3,3,3,3,3,
3,3,3,3,3,3,3,3,3,3,3,3,3,3,3,3,3,3,3,3,3,3,3,3,3,3,3,3,4),(19.9715722086605,
20.0845648631634,20.1977996632066,20.3114400836798,20.4044354265285,20.5101670042602,
20.6184055298206,20.7238689194144,20.8292727152366,20.9346522749201,21.0450080083761,
21.1505094220841,21.2560786563325,21.3618096917317,21.3760752087441,21.4817975945836,
21.5900372691306,21.6954919850707,21.8008873214135,21.9062586477675,22.0166227335656,
22.122116566379,22.2276784506292,22.3334025093939,22.3477149909598,22.4533639643363,
22.5616128154412,22.6669935098671,22.7723148103133,22.8776122117521,22.9880478521079,
23.0934689019899,23.1989584650854,23.3046113595733,23.3193547731754,23.4252154579137,
23.5334378450984,23.6390299220907,23.7445618842346,23.8500688759196,23.9603002957875,
24.0659258402978,24.1716179474442,24.2774692406294,24.2909945553911,24.396212889557,
24.5002025561162,24.6041013784337,24.7079469742604,24.8141455378748,24.9180483982882,
25.0253948135031,25.1327412287181),.UNSPECIFIED.) ;
#1735=B_SPLINE_CURVE_WITH_KNOTS('',3,(#113227,#113228,#113229,#113230),
 .UNSPECIFIED.,.F.,.F.,(4,4),(-0.0367209699986071,0.),.UNSPECIFIED.) ;
#1736=B_SPLINE_CURVE_WITH_KNOTS('',3,(#113235,#113236,#113237,#113238,#113239,
#113240,#113241,#113242),.UNSPECIFIED.,.F.,.F.,(4,1,1,1,1,4),(-39.7722845163973,
-38.7779774034875,-37.7836702905775,-36.7893631776676,-35.7950560647577,
-35.5086795309852),.UNSPECIFIED.) ;
#1737=B_SPLINE_CURVE_WITH_KNOTS('',3,(#113244,#113245,#113246,#113247,#113248,
#113249,#113250,#113251,#113252,#113253,#113254,#113255,#113256,#113257,
#113258,#113259,#113260,#113261,#113262,#113263,#113264,#113265,#113266,
#113267,#113268,#113269,#113270,#113271,#113272,#113273,#113274,#113275,
#113276,#113277,#113278,#113279,#113280,#113281,#113282,#113283,#113284,
#113285,#113286,#113287,#113288,#113289,#113290,#113291,#113292,#113293,
#113294,#113295,#113296,#113297,#113298,#113299,#113300,#113301,#113302,
#113303,#113304,#113305,#113306,#113307,#113308,#113309,#113310,#113311,
#113312,#113313,#113314,#113315,#113316,#113317,#113318,#113319,#113320,
#113321,#113322,#113323,#113324,#113325,#113326,#113327,#113328,#113329,
#113330,#113331,#113332,#113333,#113334,#113335,#113336,#113337,#113338,
#113339,#113340,#113341,#113342,#113343,#113344,#113345,#113346,#113347,
#113348,#113349,#113350,#113351,#113352,#113353,#113354,#113355,#113356,
#113357,#113358,#113359,#113360,#113361,#113362,#113363,#113364,#113365,
#113366,#113367,#113368,#113369,#113370,#113371,#113372,#113373,#113374,
#113375,#113376,#113377,#113378,#113379,#113380,#113381,#113382,#113383,
#113384,#113385,#113386,#113387,#113388,#113389,#113390,#113391,#113392,
#113393,#113394,#113395,#113396,#113397,#113398,#113399,#113400,#113401,
#113402,#113403,#113404,#113405,#113406,#113407,#113408,#113409,#113410,
#113411,#113412,#113413,#113414,#113415,#113416,#113417,#113418,#113419,
#113420,#113421,#113422,#113423,#113424,#113425,#113426,#113427,#113428,
#113429,#113430,#113431,#113432,#113433),.UNSPECIFIED.,.F.,.F.,(4,3,3,3,
3,3,3,3,3,3,3,3,3,3,3,3,3,3,3,3,3,3,3,3,3,3,3,3,3,3,3,3,3,3,3,3,3,3,3,3,
3,3,3,3,3,3,3,3,3,3,3,3,3,3,3,3,3,3,3,3,3,3,3,4),(-35.5086755760922,-35.4044022275757,
-35.3001748457792,-35.1959564275686,-35.0916365673699,-34.9872656491195,
-34.8827030128636,-34.8007489518477,-34.6953269562437,-34.590062699299,
-34.4849213620955,-34.3798454078011,-34.2747989300688,-34.1697460662361,
-34.0645822019727,-33.9593555008014,-33.8539493708266,-33.8064418389378,
-33.7010087123129,-33.5957328956943,-33.4905794204482,-33.3854909757382,
-33.280431674028,-33.1753656711069,-33.0701882799077,-32.9649478104766,
-32.859527683096,-32.8121347260278,-32.7067227907937,-32.6014685704431,
-32.4963371822769,-32.3912711160732,-32.2862344494186,-32.1811913035088,
-32.0760369477011,-31.9708196485666,-31.8654226574899,-31.8178276131179,
-31.7124073632301,-31.6071447184869,-31.5020047860233,-31.3969301063105,
-31.2918847704261,-31.1868329129934,-31.0816698418366,-30.9764438127394,
-30.8710381603998,-30.823520500208,-30.7180998986488,-30.6128368710002,
-30.5076965111687,-30.4026213766816,-30.2975755592732,-30.1925231941935,
-30.0873595792423,-29.9821329848799,-29.8767267400281,-29.8292133872981,
-29.7224635603256,-29.6158838669993,-29.5094623746583,-29.4031341758113,
-29.2968586465874,-29.2254902689127),.UNSPECIFIED.) ;
#1738=B_SPLINE_CURVE_WITH_KNOTS('',3,(#113435,#113436,#113437,#113438,#113439,
#113440,#113441,#113442,#113443,#113444,#113445,#113446,#113447,#113448,
#113449,#113450,#113451,#113452,#113453,#113454,#113455,#113456,#113457,
#113458,#113459,#113460,#113461,#113462,#113463,#113464,#113465,#113466,
#113467,#113468,#113469,#113470,#113471,#113472,#113473,#113474,#113475,
#113476,#113477,#113478,#113479,#113480,#113481,#113482,#113483,#113484,
#113485,#113486,#113487,#113488,#113489,#113490,#113491,#113492,#113493,
#113494,#113495,#113496,#113497,#113498,#113499,#113500,#113501,#113502,
#113503,#113504,#113505,#113506,#113507,#113508,#113509,#113510,#113511,
#113512,#113513,#113514,#113515,#113516,#113517,#113518,#113519,#113520,
#113521,#113522,#113523,#113524,#113525,#113526,#113527,#113528,#113529,
#113530,#113531,#113532,#113533,#113534,#113535,#113536,#113537,#113538,
#113539,#113540,#113541,#113542,#113543,#113544,#113545,#113546,#113547,
#113548,#113549,#113550,#113551,#113552,#113553,#113554,#113555,#113556,
#113557,#113558,#113559,#113560,#113561,#113562,#113563,#113564,#113565,
#113566,#113567,#113568,#113569,#113570,#113571,#113572,#113573,#113574,
#113575,#113576,#113577,#113578,#113579,#113580,#113581,#113582,#113583,
#113584,#113585,#113586,#113587,#113588,#113589,#113590,#113591,#113592,
#113593,#113594,#113595,#113596,#113597,#113598,#113599,#113600,#113601,
#113602,#113603,#113604,#113605,#113606,#113607,#113608,#113609,#113610,
#113611,#113612,#113613,#113614,#113615,#113616,#113617,#113618,#113619,
#113620,#113621,#113622,#113623,#113624),.UNSPECIFIED.,.F.,.F.,(4,3,3,3,
3,3,3,3,3,3,3,3,3,3,3,3,3,3,3,3,3,3,3,3,3,3,3,3,3,3,3,3,3,3,3,3,3,3,3,3,
3,3,3,3,3,3,3,3,3,3,3,3,3,3,3,3,3,3,3,3,3,3,3,4),(-29.2254902685167,-29.1088417077146,
-28.9917385973977,-28.8740574296362,-28.8349062743881,-28.7294867233392,
-28.6242247724242,-28.5190855227818,-28.4140115186036,-28.3089668498783,
-28.2039156501323,-28.0987532177186,-27.9935278174278,-27.8881227719779,
-27.8405991614782,-27.7351796522675,-27.6299177413909,-27.5247785289052,
-27.419704560066,-27.3146599248016,-27.2096087565756,-27.1044463525154,
-26.9992209788055,-26.8938159569209,-26.8462920485682,-26.7408727177183,
-26.6356109889847,-26.5304719633295,-26.4253981841197,-26.3203537409896,
-26.2153027671114,-26.1101405594126,-26.0049153834966,-25.8995105595505,
-25.8519849356583,-25.746565505444,-25.6413036758188,-25.5361645475202,
-25.4310906646418,-25.3260461169799,-25.2209950378678,-25.1158327245988,
-25.0106074427696,-24.9052025134882,-24.8576778227484,-24.7522584043583,
-24.6469965865146,-24.5418574698731,-24.436783598567,-24.331739062374,-24.2266879946087,
-24.1215256924225,-24.0163004215407,-23.9108955028829,-23.8633707098384,
-23.7590253019421,-23.6548572600467,-23.5507881656705,-23.4467805861788,
-23.34279717317,-23.238732933035,-23.1346302543012,-23.0303500238302,-22.9423049621638),
 .UNSPECIFIED.) ;
#1739=B_SPLINE_CURVE_WITH_KNOTS('',3,(#113626,#113627,#113628,#113629,#113630,
#113631,#113632,#113633,#113634,#113635,#113636,#113637,#113638,#113639,
#113640,#113641,#113642,#113643,#113644,#113645,#113646,#113647,#113648,
#113649,#113650,#113651,#113652,#113653,#113654,#113655,#113656,#113657,
#113658,#113659,#113660,#113661,#113662,#113663,#113664,#113665,#113666,
#113667,#113668,#113669,#113670,#113671,#113672,#113673,#113674,#113675,
#113676,#113677,#113678,#113679,#113680,#113681,#113682,#113683,#113684,
#113685,#113686,#113687,#113688,#113689,#113690,#113691,#113692,#113693,
#113694,#113695,#113696,#113697,#113698,#113699,#113700,#113701,#113702,
#113703,#113704,#113705,#113706,#113707,#113708,#113709,#113710,#113711,
#113712,#113713,#113714,#113715,#113716,#113717,#113718,#113719,#113720,
#113721,#113722,#113723,#113724,#113725,#113726,#113727,#113728,#113729,
#113730,#113731,#113732,#113733,#113734,#113735,#113736,#113737,#113738,
#113739,#113740,#113741,#113742,#113743,#113744,#113745,#113746,#113747,
#113748,#113749,#113750,#113751,#113752,#113753,#113754,#113755,#113756,
#113757,#113758,#113759,#113760,#113761,#113762,#113763,#113764,#113765,
#113766,#113767,#113768,#113769,#113770,#113771,#113772,#113773,#113774,
#113775,#113776,#113777,#113778,#113779,#113780,#113781,#113782,#113783,
#113784,#113785,#113786,#113787,#113788,#113789,#113790,#113791,#113792,
#113793,#113794,#113795,#113796,#113797,#113798,#113799,#113800,#113801,
#113802,#113803,#113804,#113805,#113806,#113807,#113808,#113809,#113810,
#113811,#113812,#113813,#113814,#113815),.UNSPECIFIED.,.F.,.F.,(4,3,3,3,
3,3,3,3,3,3,3,3,3,3,3,3,3,3,3,3,3,3,3,3,3,3,3,3,3,3,3,3,3,3,3,3,3,3,3,3,
3,3,3,3,3,3,3,3,3,3,3,3,3,3,3,3,3,3,3,3,3,3,3,4),(-22.9423049617331,-22.8690635969285,
-22.7636441836932,-22.6583823711868,-22.5532432601264,-22.4481693945498,
-22.3431248642258,-22.2380738024606,-22.1329115064317,-22.0276862418063,
-21.9222813294921,-21.8747564840186,-21.7693370725943,-21.6640752619096,
-21.5589361526772,-21.4538622889313,-21.3488177604379,-21.2437667005001,
-21.1386044062813,-21.0333791434584,-20.9279742329166,-20.8804493711086,
-20.7750299606903,-20.6697681510407,-20.5646290428816,-20.4595551802322,
-20.3545106528565,-20.2494595940563,-20.1442973009971,-20.0390720393482,
-19.93366712999,-19.8861422581987,-19.7807228478555,-19.6754610382638,-19.5703219301372,
-19.4652480675043,-19.3602035401295,-19.2551524813143,-19.1499901882165,
-19.0447649265154,-18.9393600170848,-18.8918351452888,-18.7864157337639,
-18.6811539230014,-18.5760148137255,-18.4709409499573,-18.3658964214628,
-18.2608453615451,-18.1556830673781,-18.0504578046253,-17.9450528941805,
-17.8975280323788,-17.7921086190912,-17.6868468065444,-17.5817076954615,
-17.4766338298734,-17.371589299549,-17.2665382377944,-17.1613759417928,
-17.056150677204,-16.9507457649406,-16.9032209194689,-16.7660415444305,
-16.6591196548236),.UNSPECIFIED.) ;
#1740=B_SPLINE_CURVE_WITH_KNOTS('',3,(#113817,#113818,#113819,#113820,#113821,
#113822,#113823,#113824,#113825,#113826,#113827,#113828,#113829,#113830,
#113831,#113832,#113833,#113834,#113835,#113836,#113837,#113838,#113839,
#113840,#113841,#113842,#113843,#113844,#113845,#113846,#113847,#113848,
#113849,#113850,#113851,#113852,#113853,#113854,#113855,#113856,#113857,
#113858,#113859,#113860,#113861,#113862,#113863,#113864,#113865,#113866,
#113867,#113868,#113869,#113870,#113871,#113872,#113873,#113874,#113875,
#113876,#113877,#113878,#113879,#113880,#113881,#113882,#113883,#113884,
#113885,#113886,#113887,#113888,#113889,#113890,#113891,#113892,#113893,
#113894,#113895,#113896,#113897,#113898,#113899,#113900,#113901,#113902,
#113903,#113904,#113905,#113906,#113907,#113908,#113909,#113910,#113911,
#113912,#113913,#113914,#113915,#113916,#113917,#113918,#113919,#113920,
#113921,#113922,#113923,#113924,#113925,#113926,#113927,#113928,#113929,
#113930,#113931,#113932,#113933,#113934,#113935,#113936,#113937,#113938,
#113939,#113940,#113941,#113942,#113943,#113944,#113945,#113946,#113947,
#113948,#113949,#113950,#113951,#113952,#113953,#113954,#113955,#113956,
#113957,#113958,#113959,#113960,#113961,#113962,#113963,#113964,#113965,
#113966,#113967,#113968,#113969,#113970,#113971,#113972,#113973,#113974,
#113975,#113976,#113977,#113978,#113979,#113980,#113981,#113982,#113983,
#113984,#113985,#113986,#113987,#113988,#113989,#113990,#113991,#113992,
#113993,#113994,#113995,#113996,#113997,#113998,#113999,#114000,#114001,
#114002,#114003,#114004,#114005,#114006,#114007,#114008,#114009),
 .UNSPECIFIED.,.F.,.F.,(4,3,3,3,3,3,3,3,3,3,3,3,3,3,3,3,3,3,3,3,3,3,3,3,
3,3,3,3,3,3,3,3,3,3,3,3,3,3,3,3,3,3,3,3,3,3,3,3,3,3,3,3,3,3,3,3,3,3,3,3,
3,3,3,3,4),(-16.6591196545535,-16.5552036813066,-16.4513560625145,-16.3475392568374,
-16.2437157711178,-16.1397837879908,-16.0357856707898,-15.9316178772595,
-15.908913806559,-15.8034943869351,-15.698232568139,-15.5930934509645,-15.4880195793859,
-15.3829750431806,-15.2779239756628,-15.1727616741133,-15.0675364040917,
-14.9621314866271,-14.914606693649,-14.8091872634756,-14.7039254338822,
-14.5987863056011,-14.4937124227317,-14.3886678750699,-14.2836167959496,
-14.178454482659,-14.0732292008009,-13.9678242714792,-13.9202995807391,
-13.8148802555112,-13.7096185311161,-13.6044795078905,-13.4994057299235,
-13.3943612868513,-13.2893103118467,-13.1841481012487,-13.0789229214155,
-12.9735180920354,-12.9259924678292,-12.8205729452315,-12.715311024023,
-12.6101718057521,-12.5050978339537,-12.4000531985516,-12.2950020330076,
-12.1898396358509,-12.0846142714686,-11.9792092625234,-11.9316853549192,
-11.8262658092296,-11.7210038624508,-11.6158646151245,-11.5107906121308,
-11.4057459434607,-11.3006947426411,-11.1955323074635,-11.0903069034382,
-10.9849018528082,-10.9373782420093,-10.8292878650851,-10.7159494856573,
-10.6082494155454,-10.5006633351676,-10.3931764397244,-10.375934347374),
 .UNSPECIFIED.) ;
#1741=B_SPLINE_CURVE_WITH_KNOTS('',3,(#114011,#114012,#114013,#114014,#114015,
#114016,#114017,#114018,#114019,#114020,#114021,#114022,#114023,#114024,
#114025,#114026,#114027,#114028,#114029,#114030,#114031,#114032,#114033,
#114034,#114035,#114036,#114037,#114038,#114039,#114040,#114041,#114042,
#114043,#114044,#114045,#114046,#114047,#114048,#114049,#114050,#114051,
#114052,#114053,#114054,#114055,#114056,#114057,#114058,#114059,#114060,
#114061,#114062,#114063,#114064,#114065,#114066,#114067,#114068,#114069,
#114070,#114071,#114072,#114073,#114074,#114075,#114076,#114077,#114078,
#114079,#114080,#114081,#114082,#114083,#114084,#114085,#114086,#114087,
#114088,#114089,#114090,#114091,#114092,#114093,#114094,#114095,#114096,
#114097,#114098,#114099,#114100,#114101,#114102,#114103,#114104,#114105,
#114106,#114107,#114108,#114109,#114110,#114111,#114112,#114113,#114114,
#114115,#114116,#114117,#114118,#114119,#114120,#114121,#114122,#114123,
#114124,#114125,#114126,#114127,#114128,#114129,#114130,#114131,#114132,
#114133,#114134,#114135,#114136,#114137,#114138,#114139,#114140,#114141,
#114142,#114143,#114144,#114145,#114146,#114147,#114148,#114149,#114150,
#114151,#114152,#114153,#114154,#114155,#114156,#114157,#114158,#114159,
#114160,#114161,#114162,#114163,#114164,#114165,#114166,#114167,#114168,
#114169,#114170,#114171,#114172,#114173,#114174,#114175,#114176,#114177,
#114178,#114179,#114180,#114181,#114182,#114183,#114184,#114185,#114186,
#114187,#114188,#114189,#114190,#114191,#114192,#114193,#114194,#114195,
#114196,#114197,#114198,#114199,#114200),.UNSPECIFIED.,.F.,.F.,(4,3,3,3,
3,3,3,3,3,3,3,3,3,3,3,3,3,3,3,3,3,3,3,3,3,3,3,3,3,3,3,3,3,3,3,3,3,3,3,3,
3,3,3,3,3,3,3,3,3,3,3,3,3,3,3,3,3,3,3,3,3,3,3,4),(-10.3759343470868,-10.2622932374969,
-10.1483592599546,-10.0339564107411,-9.94307112909935,-9.83765038685958,
-9.73238725063561,-9.62724683000794,-9.52217166442452,-9.41712584557071,
-9.31207350868044,-9.20690996627838,-9.10168346994019,-8.99627736106777,
-8.94876401618942,-8.84334386834391,-8.7380813023553,-8.63294141399026,
-8.52786675683356,-8.42282142199786,-8.31776954411901,-8.21260642033977,
-8.107380320142,-8.00197456917108,-7.95445690327949,-7.84904538178143,-7.74379148075398,
-7.63866027140058,-7.53359429667177,-7.42855763429612,-7.32351440552014,
-7.21835983638616,-7.1131422490107,-7.00774485805702,-6.96014979036955,
-6.85471520591697,-6.74943826420544,-6.64428415902488,-6.53919539218959,
-6.43413607566243,-6.329070365056,-6.22389372586801,-6.11865427247152,-6.01323555438736,
-5.96584267745961,-5.86042207933793,-5.75515890094995,-5.65001816767372,
-5.54494252227572,-5.43989605888921,-5.3348429150212,-5.2296783300615,-5.1244506551307,
-5.01904317436125,-4.97153556454968,-4.86758857729089,-4.76381948081389,
-4.66014914956136,-4.55653972806567,-4.45295345014138,-4.34929458304977,
-4.24559519972438,-4.14174369917986,-4.09274904066394),.UNSPECIFIED.) ;
#1742=B_SPLINE_CURVE_WITH_KNOTS('',3,(#114202,#114203,#114204,#114205,#114206,
#114207,#114208,#114209,#114210,#114211,#114212,#114213,#114214,#114215,
#114216,#114217,#114218,#114219,#114220,#114221,#114222,#114223,#114224,
#114225,#114226,#114227,#114228,#114229,#114230,#114231,#114232,#114233,
#114234,#114235,#114236,#114237,#114238,#114239,#114240,#114241,#114242,
#114243,#114244,#114245,#114246,#114247,#114248,#114249,#114250,#114251,
#114252,#114253,#114254,#114255,#114256,#114257,#114258,#114259,#114260,
#114261,#114262),.UNSPECIFIED.,.F.,.F.,(4,3,3,3,3,3,3,3,3,3,3,3,3,3,3,3,
3,3,3,3,4),(-4.09274904019429,-3.97722845163974,-3.87164849924216,-3.76622632436345,
-3.66092789460631,-3.55569545944398,-3.45049334973295,-3.34528594082316,
-3.23997021120549,-3.13459296743756,-3.02903986465691,-2.98292133872981,
-2.87879939642559,-2.77485099638648,-2.67099903247579,-2.56720584380832,
-2.46343385283584,-2.35957849417104,-2.25568164883975,-2.15160928322696,
-2.07317267331984),.UNSPECIFIED.) ;
#1743=B_SPLINE_CURVE_WITH_KNOTS('',3,(#114264,#114265,#114266,#114267),
 .UNSPECIFIED.,.F.,.F.,(4,4),(-0.0487081061340111,0.),.UNSPECIFIED.) ;
#1744=B_SPLINE_CURVE_WITH_KNOTS('',3,(#114271,#114272,#114273,#114274,#114275),
 .UNSPECIFIED.,.F.,.F.,(4,1,4),(0.,0.994307112909918,1.12201628671538),
 .UNSPECIFIED.) ;
#1745=B_SPLINE_CURVE_WITH_KNOTS('',3,(#114277,#114278,#114279,#114280,#114281,
#114282,#114283,#114284,#114285,#114286,#114287,#114288,#114289,#114290,
#114291,#114292,#114293,#114294,#114295,#114296,#114297,#114298,#114299,
#114300,#114301,#114302,#114303,#114304,#114305,#114306,#114307,#114308,
#114309,#114310,#114311,#114312,#114313,#114314,#114315,#114316,#114317,
#114318,#114319,#114320,#114321,#114322,#114323,#114324,#114325,#114326,
#114327,#114328,#114329,#114330,#114331,#114332,#114333,#114334,#114335,
#114336,#114337,#114338,#114339,#114340,#114341,#114342,#114343,#114344,
#114345,#114346,#114347,#114348,#114349,#114350,#114351,#114352,#114353,
#114354,#114355,#114356,#114357,#114358,#114359,#114360,#114361,#114362,
#114363,#114364,#114365,#114366,#114367,#114368,#114369,#114370,#114371,
#114372,#114373,#114374,#114375,#114376,#114377,#114378,#114379,#114380,
#114381,#114382,#114383,#114384,#114385,#114386,#114387,#114388,#114389,
#114390,#114391,#114392,#114393,#114394,#114395,#114396,#114397,#114398,
#114399,#114400,#114401,#114402,#114403,#114404,#114405,#114406,#114407,
#114408,#114409,#114410,#114411,#114412,#114413,#114414,#114415,#114416,
#114417,#114418,#114419,#114420,#114421,#114422,#114423,#114424,#114425,
#114426,#114427,#114428,#114429,#114430,#114431,#114432,#114433,#114434,
#114435,#114436,#114437,#114438,#114439,#114440,#114441,#114442,#114443,
#114444,#114445,#114446,#114447,#114448,#114449,#114450,#114451,#114452,
#114453,#114454,#114455,#114456,#114457,#114458,#114459,#114460,#114461,
#114462,#114463,#114464,#114465,#114466),.UNSPECIFIED.,.F.,.F.,(4,3,3,3,
3,3,3,3,3,3,3,3,3,3,3,3,3,3,3,3,3,3,3,3,3,3,3,3,3,3,3,3,3,3,3,3,3,3,3,3,
3,3,3,3,3,3,3,3,3,3,3,3,3,3,3,3,3,3,3,3,3,3,3,4),(1.12201628671538,1.23034102910344,
1.33358330420648,1.43674793062772,1.53987315811359,1.64299717167808,1.74622395060981,
1.84951097348011,1.95297061142083,1.98861422581985,2.09399892739112,2.19922262279794,
2.30431881533442,2.40934681168488,2.51434260972737,2.61934216073603,2.72444914077599,
2.82961683585291,2.93496134502189,2.98292133872979,3.08848800174328,3.19389992341939,
3.29919261601425,3.40442212311023,3.50962410932036,3.6148341977006,3.72015679699726,
3.82554331992505,3.93110928046911,3.97722845163972,4.08257777213716,4.18776850937299,
4.29283544498566,4.39783649479165,4.50280768124411,4.60778498265087,4.71287339380203,
4.81802459579896,4.92335594389848,4.97153556454966,5.07695755890264,5.18222181458872,
5.28736315052821,5.39243910355605,5.49748558002122,5.60253844258718,5.70770230559402,
5.81292900551239,5.91833513425313,5.96584267745959,6.07127580375949,6.176551620046,
6.28170509495031,6.38679353931261,6.49185284066994,6.59691884323355,6.70209623407033,
6.80733670313579,6.9127568301494,6.96014979036953,7.07372300911412,7.18702116753589,
7.2998880871726,7.40520159341374),.UNSPECIFIED.) ;
#1746=B_SPLINE_CURVE_WITH_KNOTS('',3,(#114468,#114469,#114470,#114471,#114472,
#114473,#114474,#114475,#114476,#114477,#114478,#114479,#114480,#114481,
#114482,#114483,#114484,#114485,#114486,#114487,#114488,#114489,#114490,
#114491,#114492,#114493,#114494,#114495,#114496,#114497,#114498,#114499,
#114500,#114501,#114502,#114503,#114504,#114505,#114506,#114507,#114508,
#114509,#114510,#114511,#114512,#114513,#114514,#114515,#114516,#114517,
#114518,#114519,#114520,#114521,#114522,#114523,#114524,#114525,#114526,
#114527,#114528,#114529,#114530,#114531,#114532,#114533,#114534,#114535,
#114536,#114537,#114538,#114539,#114540,#114541,#114542,#114543,#114544,
#114545,#114546,#114547,#114548,#114549,#114550,#114551,#114552,#114553,
#114554,#114555,#114556,#114557,#114558,#114559,#114560,#114561,#114562,
#114563,#114564,#114565,#114566,#114567,#114568,#114569,#114570,#114571,
#114572,#114573,#114574,#114575,#114576,#114577,#114578,#114579,#114580,
#114581,#114582,#114583,#114584,#114585,#114586,#114587,#114588,#114589,
#114590,#114591,#114592,#114593,#114594,#114595,#114596,#114597,#114598,
#114599,#114600,#114601,#114602,#114603,#114604,#114605,#114606,#114607,
#114608,#114609,#114610,#114611,#114612,#114613,#114614,#114615,#114616,
#114617,#114618,#114619,#114620,#114621,#114622,#114623,#114624,#114625,
#114626,#114627,#114628,#114629,#114630,#114631,#114632,#114633,#114634,
#114635,#114636,#114637,#114638,#114639,#114640,#114641,#114642,#114643,
#114644,#114645,#114646,#114647,#114648,#114649,#114650,#114651,#114652,
#114653,#114654,#114655,#114656,#114657),.UNSPECIFIED.,.F.,.F.,(4,3,3,3,
3,3,3,3,3,3,3,3,3,3,3,3,3,3,3,3,3,3,3,3,3,3,3,3,3,3,3,3,3,3,3,3,3,3,3,3,
3,3,3,3,3,3,3,3,3,3,3,3,3,3,3,3,3,3,3,3,3,3,3,4),(7.40520159389494,7.51310671647122,
7.62344426317328,7.73165200870718,7.84305445599332,7.95445690327946,8.05987715300651,
8.16513979758751,8.27027972988675,8.37535440943424,8.4803997451524,8.58545160241827,
8.69061467340867,8.79584070233938,8.90124635451427,8.94876401618939,9.05418461770193,
9.15944764530252,9.26458800508425,9.36966313952041,9.47470895687734,9.57976132190398,
9.68492493680147,9.79015153110949,9.89555777590651,9.94307112909933,10.0484897557137,
10.1537507688988,10.2588890658611,10.3639621086595,10.4690058088096,10.574056034282,
10.6792174905251,10.7844419121692,10.8898459853794,10.9373782420093,11.0427977930361,
11.1480597439288,11.2531989935486,11.3582729977041,11.4633176664064,11.5683688661293,
11.6735312985203,11.7787566987884,11.8841617442156,11.9316853549192,12.0371048641248,
12.1423667749956,12.2475059874759,12.3525799563095,12.4576245915682,12.5626757597885,
12.6678381638428,12.7730635375468,12.8784685594254,12.9259924678291,13.0300394883708,
13.1339455877987,13.2377486448433,13.3414863916629,13.4452303857489,13.5489787431586,
13.652816925385,13.6883869007106),.UNSPECIFIED.) ;
#1747=B_SPLINE_CURVE_WITH_KNOTS('',3,(#114659,#114660,#114661,#114662,#114663,
#114664,#114665,#114666,#114667,#114668,#114669,#114670,#114671,#114672,
#114673,#114674,#114675,#114676,#114677,#114678,#114679,#114680,#114681,
#114682,#114683,#114684,#114685,#114686,#114687,#114688,#114689,#114690,
#114691,#114692,#114693,#114694,#114695,#114696,#114697,#114698,#114699,
#114700,#114701,#114702,#114703,#114704,#114705,#114706,#114707,#114708,
#114709,#114710,#114711,#114712,#114713,#114714,#114715,#114716,#114717,
#114718,#114719,#114720,#114721,#114722,#114723,#114724,#114725,#114726,
#114727,#114728,#114729,#114730,#114731,#114732,#114733,#114734,#114735,
#114736,#114737,#114738,#114739,#114740,#114741,#114742,#114743,#114744,
#114745,#114746,#114747,#114748,#114749,#114750,#114751,#114752,#114753,
#114754,#114755,#114756,#114757,#114758,#114759,#114760,#114761,#114762,
#114763,#114764,#114765,#114766,#114767,#114768,#114769,#114770,#114771,
#114772,#114773,#114774,#114775,#114776,#114777,#114778,#114779,#114780,
#114781,#114782,#114783,#114784,#114785,#114786,#114787,#114788,#114789,
#114790,#114791,#114792,#114793,#114794,#114795,#114796,#114797,#114798,
#114799,#114800,#114801,#114802,#114803,#114804,#114805,#114806,#114807,
#114808,#114809,#114810,#114811,#114812,#114813,#114814,#114815,#114816,
#114817,#114818,#114819,#114820,#114821,#114822,#114823,#114824,#114825,
#114826,#114827,#114828,#114829,#114830,#114831,#114832,#114833,#114834,
#114835,#114836,#114837,#114838,#114839,#114840,#114841,#114842,#114843,
#114844,#114845,#114846,#114847,#114848),.UNSPECIFIED.,.F.,.F.,(4,3,3,3,
3,3,3,3,3,3,3,3,3,3,3,3,3,3,3,3,3,3,3,3,3,3,3,3,3,3,3,3,3,3,3,3,3,3,3,3,
3,3,3,3,3,3,3,3,3,3,3,3,3,3,3,3,3,3,3,3,3,3,3,4),(13.6883869010745,13.8285226780631,
13.9202995807391,14.0257190109509,14.1309808405734,14.2361199688695,14.3411938517453,
14.4462383994047,14.5512894785142,14.6564517917807,14.7616770736072,14.8670820028861,
14.914606693649,15.0200261120377,15.1252879298801,15.2304270465202,15.3355009178248,
15.4405454540164,15.5455965217802,15.6507588239649,15.7559840948451,15.8613890135014,
15.9089138065589,16.0143332095239,16.1195950115914,16.2247341120157,16.3298079668403,
16.4348524863131,16.5399035371446,16.6450658221904,16.7502910757889,16.8556959771237,
16.9032209194689,17.0086403327036,17.1139021452095,17.2190412562692,17.3241151218452,
17.4291596521685,17.5342107139331,17.6393730099613,17.7445982745861,17.8500031868997,
17.8975280323788,18.0029474438031,18.1082092544879,18.2133483637203,18.3184222274662,
18.4234667559597,18.5285178158973,18.6336801101162,18.738905372939,18.8443102834809,
18.8918351452887,18.9972545557072,19.1025163653571,19.2076554735164,19.3127293361661,
19.417773863542,19.5228249223424,19.6279872154019,19.7332124770511,19.8386173864095,
19.8861422581987,19.9715722082541),.UNSPECIFIED.) ;
#1748=B_SPLINE_CURVE_WITH_KNOTS('',3,(#114850,#114851,#114852,#114853,#114854,
#114855,#114856,#114857,#114858,#114859,#114860,#114861,#114862,#114863,
#114864,#114865,#114866,#114867,#114868,#114869,#114870,#114871,#114872,
#114873,#114874,#114875,#114876,#114877,#114878,#114879,#114880,#114881,
#114882,#114883,#114884,#114885,#114886,#114887,#114888,#114889,#114890,
#114891,#114892,#114893,#114894,#114895,#114896,#114897,#114898,#114899,
#114900,#114901,#114902,#114903,#114904,#114905,#114906,#114907,#114908,
#114909,#114910,#114911,#114912,#114913,#114914,#114915,#114916,#114917,
#114918,#114919,#114920,#114921,#114922,#114923,#114924,#114925,#114926,
#114927,#114928,#114929,#114930,#114931,#114932,#114933,#114934,#114935,
#114936,#114937,#114938,#114939,#114940,#114941,#114942,#114943,#114944,
#114945,#114946,#114947,#114948,#114949,#114950,#114951,#114952,#114953,
#114954,#114955,#114956,#114957,#114958,#114959,#114960,#114961,#114962,
#114963,#114964,#114965,#114966,#114967,#114968,#114969,#114970,#114971,
#114972,#114973,#114974,#114975,#114976,#114977,#114978,#114979,#114980,
#114981,#114982,#114983,#114984,#114985,#114986,#114987,#114988,#114989,
#114990,#114991,#114992,#114993,#114994,#114995,#114996,#114997,#114998,
#114999,#115000,#115001,#115002,#115003,#115004,#115005,#115006,#115007,
#115008,#115009,#115010,#115011,#115012,#115013,#115014,#115015,#115016,
#115017,#115018,#115019,#115020,#115021,#115022,#115023,#115024,#115025,
#115026,#115027,#115028,#115029,#115030,#115031,#115032,#115033,#115034,
#115035,#115036,#115037,#115038,#115039),.UNSPECIFIED.,.F.,.F.,(4,3,3,3,
3,3,3,3,3,3,3,3,3,3,3,3,3,3,3,3,3,3,3,3,3,3,3,3,3,3,3,3,3,3,3,3,3,3,3,3,
3,3,3,3,3,3,3,3,3,3,3,3,3,3,3,3,3,3,3,3,3,3,3,4),(19.9715722087079,20.0757526573405,
20.1797732687495,20.2837058335539,20.3875878870888,20.4914568929667,20.5954209680976,
20.699433391534,20.8036305474994,20.8804493711086,20.9858687826337,21.0911305933964,
21.1962697026724,21.3013435664408,21.4063880949356,21.5114391548532,21.6166014490203,
21.7218267117734,21.8272316222182,21.8747564840186,21.9801758973058,22.0854377098522,
22.1905768209346,22.2956506865221,22.4006952168461,22.5057462786001,22.6109085746013,
22.7161338391897,22.8215387514525,22.8690635969285,22.9744829992754,23.0797448008656,
23.1848839010226,23.2899577557102,23.3950022751763,23.5000533261311,23.6052156114951,
23.7104408655235,23.8158457674549,23.8633707098384,23.9687901294618,24.0740519482573,
24.1791910654315,24.2842649370099,24.3893094732149,24.4943605407323,24.5995228422816,
24.7047481123027,24.8101530297671,24.8576778227484,24.9630972529186,25.0683590825089,
25.1734982107868,25.2785720936532,25.3836166413118,25.4886677204293,25.5938300337168,
25.6990553155718,25.8044602448903,25.8519849356583,25.9685846308431,26.0848174253634,
26.2004492469501,26.2547575150606),.UNSPECIFIED.) ;
#1749=B_SPLINE_CURVE_WITH_KNOTS('',3,(#115041,#115042,#115043,#115044,#115045,
#115046,#115047,#115048,#115049,#115050,#115051,#115052,#115053,#115054,
#115055,#115056,#115057,#115058,#115059,#115060,#115061,#115062,#115063,
#115064,#115065,#115066,#115067,#115068,#115069,#115070,#115071,#115072,
#115073,#115074,#115075,#115076,#115077,#115078,#115079,#115080,#115081,
#115082,#115083,#115084,#115085,#115086,#115087,#115088,#115089,#115090,
#115091,#115092,#115093,#115094,#115095,#115096,#115097,#115098,#115099,
#115100,#115101,#115102,#115103,#115104,#115105,#115106,#115107,#115108,
#115109,#115110,#115111,#115112,#115113,#115114,#115115,#115116,#115117,
#115118,#115119,#115120,#115121,#115122,#115123,#115124,#115125,#115126,
#115127,#115128,#115129,#115130,#115131,#115132,#115133,#115134,#115135,
#115136,#115137,#115138,#115139,#115140,#115141,#115142,#115143,#115144,
#115145,#115146,#115147,#115148,#115149,#115150,#115151,#115152,#115153,
#115154,#115155,#115156,#115157,#115158,#115159,#115160,#115161,#115162,
#115163,#115164,#115165,#115166,#115167,#115168,#115169,#115170,#115171,
#115172,#115173,#115174,#115175,#115176,#115177,#115178,#115179,#115180,
#115181,#115182,#115183,#115184,#115185,#115186,#115187,#115188,#115189,
#115190,#115191,#115192,#115193,#115194,#115195,#115196,#115197,#115198,
#115199,#115200,#115201,#115202,#115203,#115204,#115205,#115206,#115207,
#115208,#115209,#115210,#115211,#115212,#115213,#115214,#115215,#115216,
#115217,#115218,#115219,#115220,#115221,#115222,#115223,#115224,#115225,
#115226,#115227,#115228,#115229,#115230),.UNSPECIFIED.,.F.,.F.,(4,3,3,3,
3,3,3,3,3,3,3,3,3,3,3,3,3,3,3,3,3,3,3,3,3,3,3,3,3,3,3,3,3,3,3,3,3,3,3,3,
3,3,3,3,3,3,3,3,3,3,3,3,3,3,3,3,3,3,3,3,3,3,3,4),(26.2547575154336,26.3613465931618,
26.4679789682056,26.5747709772014,26.6816506924515,26.7887463962673,26.8462920485682,
26.9517115711595,27.0569734923618,27.1621127106266,27.2671866824188,27.3722313178148,
27.4772824833525,27.5824448805035,27.68767024488,27.7930752538197,27.8405991614782,
27.9460187071456,28.0512806539019,28.1564199012058,28.2614939041769,28.3665385728247,
28.4715897736222,28.5767522087774,28.6819776127802,28.7873826633883,28.8349062743881,
28.9403248515837,29.0455858266276,29.1507241022328,29.2557971341069,29.3608408337486,
29.4658910691218,29.5710525508493,29.6762770069266,29.7816811279033,29.829213387298,
29.9346341294826,30.039897265652,30.1450376862259,30.2501128517563,30.3551586705575,
30.4602110073962,30.5653745497481,30.6706010460371,30.7760071548619,30.823520500208,
30.9289406478903,31.0342032137143,31.1393431019143,31.2444177589056,31.3494630935756,
31.4545149712888,31.5596780949041,31.6649041949384,31.7703099457485,31.8178276131179,
31.9222753937316,32.0265781783092,32.1307733970436,32.2349210195028,32.3390353788241,
32.4432146412587,32.5379428226133),.UNSPECIFIED.) ;
#1750=B_SPLINE_CURVE_WITH_KNOTS('',3,(#115232,#115233,#115234,#115235,#115236,
#115237,#115238,#115239,#115240,#115241,#115242,#115243,#115244,#115245,
#115246,#115247,#115248,#115249,#115250,#115251,#115252,#115253,#115254,
#115255,#115256,#115257,#115258,#115259,#115260,#115261,#115262,#115263,
#115264,#115265,#115266,#115267,#115268,#115269,#115270,#115271,#115272,
#115273,#115274,#115275,#115276,#115277,#115278,#115279,#115280,#115281,
#115282,#115283,#115284,#115285,#115286,#115287,#115288,#115289,#115290,
#115291,#115292,#115293,#115294,#115295,#115296,#115297,#115298,#115299,
#115300,#115301,#115302,#115303,#115304,#115305,#115306,#115307,#115308,
#115309,#115310,#115311,#115312,#115313,#115314,#115315,#115316,#115317,
#115318,#115319,#115320,#115321,#115322,#115323,#115324,#115325,#115326,
#115327,#115328,#115329,#115330,#115331,#115332,#115333,#115334,#115335,
#115336,#115337,#115338,#115339,#115340,#115341,#115342,#115343,#115344,
#115345,#115346,#115347,#115348,#115349,#115350,#115351,#115352,#115353,
#115354,#115355,#115356,#115357,#115358,#115359,#115360,#115361,#115362,
#115363,#115364,#115365,#115366,#115367,#115368,#115369,#115370,#115371,
#115372,#115373,#115374,#115375,#115376,#115377,#115378,#115379,#115380,
#115381,#115382,#115383,#115384,#115385,#115386,#115387,#115388),
 .UNSPECIFIED.,.F.,.F.,(4,3,3,3,3,3,3,3,3,3,3,3,3,3,3,3,3,3,3,3,3,3,3,3,
3,3,3,3,3,3,3,3,3,3,3,3,3,3,3,3,3,3,3,3,3,3,3,3,3,3,3,3,4),(32.5379428229721,
32.6678523512312,32.8000400073029,32.8121347260278,32.9175693101144,33.0228462514619,
33.1280003562829,33.2330891227617,33.3381484389358,33.4432141491931,33.5483907880401,
33.6536302410997,33.7590489588567,33.8064418389378,33.9118624358314,34.0171256129785,
34.1222663450006,34.227341989137,34.3323884512563,34.4374415938531,34.5426061775443,
34.6478338512062,34.7532413307192,34.8007489518477,34.9060950858955,35.0112833633988,
35.1163489210678,35.2213492651478,35.3263204169927,35.4312983545223,35.5363884064698,
35.6415418258675,35.7468762517544,35.7950560647576,35.9006360132837,36.0060581843695,
36.1113566104704,36.2165890420641,36.3217911483003,36.4269985538351,36.5323142802526,
36.6376915209163,36.7432446207726,36.7893631776676,36.8934851122297,36.9974335047275,
37.101285461222,37.2050786426096,37.3088506264494,37.412705978262,37.5166028168842,
37.6206751761,37.6991118430775),.UNSPECIFIED.) ;
#1751=B_SPLINE_CURVE_WITH_KNOTS('',3,(#115389,#115390,#115391,#115392),
 .UNSPECIFIED.,.F.,.F.,(4,4),(-0.0487088993428013,0.),.UNSPECIFIED.) ;
#1752=B_SPLINE_CURVE_WITH_KNOTS('',3,(#115397,#115398,#115399,#115400,#115401,
#115402,#115403,#115404,#115405,#115406,#115407,#115408,#115409,#115410,
#115411,#115412,#115413,#115414,#115415,#115416,#115417,#115418,#115419,
#115420,#115421,#115422,#115423,#115424,#115425,#115426,#115427,#115428,
#115429,#115430,#115431,#115432,#115433,#115434,#115435,#115436,#115437,
#115438,#115439,#115440,#115441,#115442,#115443,#115444,#115445,#115446,
#115447,#115448,#115449,#115450,#115451,#115452,#115453,#115454,#115455,
#115456,#115457,#115458,#115459,#115460,#115461,#115462,#115463,#115464,
#115465,#115466,#115467,#115468,#115469,#115470,#115471,#115472,#115473,
#115474,#115475,#115476,#115477,#115478,#115479,#115480,#115481,#115482,
#115483,#115484,#115485,#115486,#115487,#115488,#115489,#115490,#115491,
#115492,#115493,#115494,#115495,#115496,#115497,#115498,#115499,#115500,
#115501,#115502,#115503,#115504),.UNSPECIFIED.,.F.,.F.,(4,2,2,2,2,2,2,2,
2,2,2,2,2,2,2,2,2,2,2,2,2,2,2,2,2,2,2,2,2,2,2,2,2,2,2,2,2,2,2,2,2,2,2,2,
2,2,2,2,2,2,2,2,2,4),(-0.712529018801462,-0.692215766132187,-0.664135864238742,
-0.658240027550338,-0.65482564774828,-0.651510806762373,-0.646109027517185,
-0.620883198311623,-0.586121850216688,-0.5772399037717,-0.571437147349492,
-0.565706665075696,-0.557223325800328,-0.547208645040879,-0.525513742714016,
-0.497097727813206,-0.491238951503433,-0.487834075555186,-0.484537915090653,
-0.479163400168952,-0.454304399302376,-0.418678985728483,-0.409866567247856,
-0.404097580583173,-0.398395458960152,-0.389949910340539,-0.360561181362236,
-0.329412523059719,-0.323757230869978,-0.320400114298294,-0.317033346831293,
-0.311416967020911,-0.282511821131457,-0.252233820777348,-0.243100580417461,
-0.237232557741588,-0.231505891629165,-0.22315293004513,-0.189759578067865,
-0.163006081390897,-0.156972073278048,-0.15351761524682,-0.150169378793417,
-0.144734566387307,-0.137933698959475,-0.122196090774211,-0.0850532115423573,
-0.0765779487325186,-0.0714002462994081,-0.0656613420703193,-0.0572626031513613,
-0.0474086202233217,-0.0264640630640861,-0.00352947697862977),
 .UNSPECIFIED.) ;
#1753=B_SPLINE_CURVE_WITH_KNOTS('',3,(#115508,#115509,#115510,#115511,#115512,
#115513,#115514,#115515,#115516,#115517,#115518,#115519,#115520,#115521,
#115522,#115523,#115524,#115525,#115526,#115527,#115528,#115529,#115530,
#115531,#115532,#115533,#115534,#115535),.UNSPECIFIED.,.F.,.F.,(4,3,3,3,
3,3,3,3,3,4),(47.1238898043947,47.2352837902631,47.3464400309164,47.4574585890731,
47.5683762665546,47.6792297317267,47.7900945032509,47.900961870412,48.0119293664921,
48.0750461904514),.UNSPECIFIED.) ;
#1754=B_SPLINE_CURVE_WITH_KNOTS('',3,(#115536,#115537,#115538,#115539,#115540,
#115541,#115542,#115543,#115544,#115545,#115546,#115547,#115548,#115549,
#115550,#115551,#115552,#115553,#115554,#115555,#115556,#115557,#115558,
#115559,#115560,#115561,#115562,#115563,#115564,#115565,#115566,#115567,
#115568,#115569,#115570,#115571,#115572,#115573,#115574,#115575,#115576,
#115577,#115578,#115579,#115580,#115581,#115582,#115583,#115584,#115585,
#115586,#115587,#115588,#115589,#115590,#115591,#115592,#115593,#115594,
#115595,#115596),.UNSPECIFIED.,.F.,.F.,(4,3,3,3,3,3,3,3,3,3,3,3,3,3,3,3,
3,3,3,3,4),(45.0774317841423,45.0921248517216,45.2017087476041,45.3122991497326,
45.4215907363396,45.5308188028355,45.6400238367858,45.7516258687472,45.8609770374908,
45.9737045010611,46.0864319646315,46.1954426168905,46.3061046744719,46.4148166958695,
46.5234644023138,46.6320892195687,46.7442516840619,46.8530297571829,46.9668844173622,
47.0807390775415,47.1238898038469),.UNSPECIFIED.) ;
#1755=B_SPLINE_CURVE_WITH_KNOTS('',3,(#115599,#115600,#115601,#115602,#115603,
#115604,#115605,#115606,#115607,#115608,#115609,#115610,#115611,#115612,
#115613,#115614,#115615,#115616,#115617,#115618,#115619,#115620,#115621,
#115622,#115623,#115624,#115625,#115626,#115627,#115628,#115629,#115630,
#115631,#115632,#115633,#115634,#115635,#115636,#115637,#115638,#115639,
#115640,#115641,#115642,#115643,#115644,#115645,#115646,#115647,#115648,
#115649,#115650,#115651,#115652,#115653,#115654,#115655,#115656,#115657,
#115658,#115659,#115660,#115661,#115662,#115663,#115664,#115665,#115666,
#115667,#115668,#115669,#115670,#115671,#115672,#115673,#115674,#115675,
#115676,#115677,#115678,#115679,#115680,#115681,#115682,#115683,#115684,
#115685,#115686,#115687,#115688,#115689,#115690,#115691,#115692,#115693,
#115694),.UNSPECIFIED.,.F.,.F.,(4,2,2,2,2,2,2,2,2,2,2,2,2,2,2,2,2,2,2,2,
2,2,2,2,2,2,2,2,2,2,2,2,2,2,2,2,2,2,2,2,2,2,2,2,2,2,2,4),(0.0026151563363548,
0.0179899578167905,0.0472044811745065,0.0576295306852423,0.0662273340337798,
0.0770918755822315,0.104350311824498,0.124050281215216,0.132515561685311,
0.139413475602386,0.144360237891016,0.151347291161069,0.179374142514947,
0.209542405261021,0.219879444032952,0.228451041843246,0.239320643288716,
0.269825786465474,0.296023856051,0.302771836078026,0.307671052620665,0.314629037379767,
0.342607736599612,0.37249921285926,0.382872374942502,0.391361215872602,
0.402138206335904,0.425642624421977,0.456294846706203,0.46460630768549,
0.469613781743472,0.475497265298997,0.487976737859294,0.515898642790773,
0.531093292477762,0.54347082513099,0.552130780531028,0.561688755483493,
0.580959665388665,0.615071972976662,0.623009519934321,0.629591131217097,
0.634497357221016,0.641651525729804,0.661384245233401,0.686587476454549,
0.703154313183141,0.712378143918981),.UNSPECIFIED.) ;
#1756=B_SPLINE_CURVE_WITH_KNOTS('',3,(#115698,#115699,#115700,#115701,#115702,
#115703,#115704,#115705,#115706,#115707,#115708,#115709,#115710,#115711,
#115712,#115713,#115714,#115715,#115716,#115717,#115718,#115719,#115720,
#115721,#115722,#115723,#115724,#115725),.UNSPECIFIED.,.F.,.F.,(4,3,3,3,
3,3,3,3,3,4),(34.557519189987,34.6694584461235,34.7811724399487,34.8927552132247,
35.0042418725079,35.1156673936037,35.2271037225296,35.338542288418,35.4500742527154,
35.508675576092),.UNSPECIFIED.) ;
#1757=B_SPLINE_CURVE_WITH_KNOTS('',3,(#115726,#115727,#115728,#115729,#115730,
#115731,#115732,#115733,#115734,#115735,#115736,#115737,#115738,#115739,
#115740,#115741,#115742,#115743,#115744,#115745,#115746,#115747,#115748,
#115749,#115750,#115751,#115752,#115753,#115754,#115755,#115756,#115757,
#115758,#115759,#115760,#115761,#115762,#115763,#115764,#115765,#115766,
#115767,#115768,#115769,#115770,#115771,#115772,#115773,#115774,#115775,
#115776,#115777,#115778,#115779,#115780,#115781,#115782,#115783,#115784,
#115785,#115786),.UNSPECIFIED.,.F.,.F.,(4,3,3,3,3,3,3,3,3,3,3,3,3,3,3,3,
3,3,3,3,4),(32.5109032341381,32.5937562294451,32.7036640037873,32.8133945161912,
32.9230264084955,33.0325996547794,33.1421541476789,33.2518066805613,33.3615061631074,
33.4714063488116,33.5653960116607,33.6748026965323,33.7840268426677,33.8931495282482,
34.0022116569275,34.1112540474795,34.2203971020844,34.3295877652005,34.4389867358328,
34.5370357938764,34.5575191894878),.UNSPECIFIED.) ;
#1758=B_SPLINE_CURVE_WITH_KNOTS('',3,(#115788,#115789,#115790,#115791,#115792,
#115793,#115794,#115795,#115796,#115797,#115798,#115799,#115800,#115801,
#115802,#115803,#115804,#115805,#115806,#115807,#115808,#115809,#115810,
#115811,#115812,#115813,#115814,#115815,#115816,#115817,#115818,#115819,
#115820,#115821,#115822,#115823,#115824,#115825,#115826,#115827,#115828,
#115829,#115830,#115831,#115832,#115833,#115834,#115835,#115836,#115837,
#115838,#115839,#115840,#115841,#115842,#115843,#115844,#115845,#115846,
#115847,#115848,#115849,#115850,#115851,#115852,#115853,#115854,#115855,
#115856,#115857,#115858,#115859,#115860,#115861,#115862,#115863,#115864,
#115865,#115866,#115867,#115868,#115869,#115870,#115871,#115872),
 .UNSPECIFIED.,.F.,.F.,(4,3,3,3,3,3,3,3,3,3,3,3,3,3,3,3,3,3,3,3,3,3,3,3,
3,3,3,3,4),(-0.375230238529917,-0.357518914002748,-0.353499339011933,-0.330618426268482,
-0.324807980319591,-0.303153187739658,-0.286565543905241,-0.280293721854319,
-0.274975125238719,-0.253681437664564,-0.232737497017393,-0.217166132029125,
-0.208374669734109,-0.204725951335004,-0.184285942423822,-0.170452037064323,
-0.149145532431283,-0.139823936654328,-0.135833708785121,-0.132392631626963,
-0.112078350447567,-0.0917069570560497,-0.071654175354626,-0.0676263159013853,
-0.0641204348977771,-0.0443305734284611,-0.0248574443104007,-0.00603170532718953,
0.),.UNSPECIFIED.) ;
#1759=B_SPLINE_CURVE_WITH_KNOTS('',3,(#115874,#115875,#115876,#115877),
 .UNSPECIFIED.,.F.,.F.,(4,4),(0.,0.0129878021108932),.UNSPECIFIED.) ;
#1760=B_SPLINE_CURVE_WITH_KNOTS('',3,(#115878,#115879,#115880,#115881,#115882,
#115883,#115884,#115885,#115886,#115887,#115888,#115889,#115890,#115891,
#115892,#115893,#115894,#115895,#115896,#115897,#115898,#115899,#115900,
#115901,#115902,#115903,#115904,#115905,#115906,#115907,#115908,#115909,
#115910,#115911,#115912,#115913,#115914,#115915,#115916,#115917,#115918,
#115919,#115920,#115921,#115922,#115923,#115924,#115925,#115926,#115927,
#115928,#115929,#115930,#115931,#115932,#115933,#115934,#115935,#115936,
#115937,#115938,#115939,#115940,#115941,#115942,#115943,#115944,#115945,
#115946,#115947,#115948,#115949,#115950,#115951,#115952,#115953,#115954,
#115955,#115956,#115957,#115958,#115959,#115960,#115961,#115962,#115963,
#115964,#115965),.UNSPECIFIED.,.F.,.F.,(4,3,3,3,3,3,3,3,3,3,3,3,3,3,3,3,
3,3,3,3,3,3,3,3,3,3,3,3,3,4),(-0.380169894663495,-0.360311041953257,-0.358093714841347,
-0.344714901897815,-0.336915301102773,-0.332696968908371,-0.312888567026539,
-0.296964077029212,-0.291611757449479,-0.287054572082553,-0.266750979851411,
-0.246125107358001,-0.23096699228048,-0.222333842397338,-0.217980610353271,
-0.196924266505527,-0.185492647047918,-0.164983292057223,-0.154671836303647,
-0.149608821797306,-0.146454059323621,-0.125463742568063,-0.104059845569569,
-0.082556275683466,-0.0772769044299627,-0.0730030946602837,-0.0510590776608034,
-0.0291391974875742,-0.0077601331035521,0.),.UNSPECIFIED.) ;
#1761=B_SPLINE_CURVE_WITH_KNOTS('',3,(#116091,#116092,#116093,#116094,#116095,
#116096,#116097,#116098,#116099,#116100,#116101,#116102,#116103,#116104,
#116105,#116106,#116107,#116108,#116109,#116110,#116111,#116112,#116113,
#116114,#116115,#116116,#116117,#116118,#116119,#116120,#116121,#116122,
#116123,#116124,#116125,#116126,#116127,#116128,#116129,#116130,#116131,
#116132,#116133,#116134,#116135,#116136,#116137,#116138,#116139,#116140,
#116141,#116142,#116143,#116144,#116145,#116146,#116147,#116148,#116149,
#116150,#116151,#116152,#116153,#116154,#116155,#116156,#116157,#116158,
#116159,#116160,#116161,#116162,#116163,#116164,#116165,#116166,#116167,
#116168,#116169,#116170,#116171,#116172,#116173,#116174,#116175,#116176,
#116177,#116178),.UNSPECIFIED.,.F.,.F.,(4,3,3,3,3,3,3,3,3,3,3,3,3,3,3,3,
3,3,3,3,3,3,3,3,3,3,3,3,3,4),(-0.380169894663605,-0.360311041858371,-0.358093714841452,
-0.344714902065716,-0.336915300765293,-0.33269696876484,-0.312888566814864,
-0.296964076844001,-0.291611755955825,-0.287054571535372,-0.266750979273317,
-0.2461251068382,-0.230966991890641,-0.222333842148618,-0.217980610319933,
-0.196924266519412,-0.185492647047962,-0.164983291825849,-0.154671836086734,
-0.149608821363363,-0.146454058645083,-0.125531321942587,-0.104043798334106,
-0.0825562747256238,-0.0772769030728362,-0.0730030943857931,-0.0510590773577688,
-0.0291391975209706,-0.00776013404481242,0.),.UNSPECIFIED.) ;
#1762=B_SPLINE_CURVE_WITH_KNOTS('',3,(#116179,#116180,#116181,#116182),
 .UNSPECIFIED.,.F.,.F.,(4,4),(-0.0129879181954274,0.),.UNSPECIFIED.) ;
#1763=B_SPLINE_CURVE_WITH_KNOTS('',3,(#116184,#116185,#116186,#116187,#116188,
#116189,#116190,#116191,#116192,#116193,#116194,#116195,#116196,#116197,
#116198,#116199,#116200,#116201,#116202,#116203,#116204,#116205,#116206,
#116207,#116208,#116209,#116210,#116211,#116212,#116213,#116214,#116215,
#116216,#116217,#116218,#116219,#116220,#116221,#116222,#116223,#116224,
#116225,#116226,#116227,#116228,#116229,#116230,#116231,#116232,#116233,
#116234,#116235,#116236,#116237,#116238,#116239,#116240,#116241,#116242,
#116243,#116244,#116245,#116246,#116247,#116248,#116249,#116250,#116251,
#116252,#116253,#116254,#116255,#116256,#116257,#116258,#116259,#116260,
#116261,#116262,#116263,#116264,#116265,#116266,#116267,#116268),
 .UNSPECIFIED.,.F.,.F.,(4,3,3,3,3,3,3,3,3,3,3,3,3,3,3,3,3,3,3,3,3,3,3,3,
3,3,3,3,4),(-0.375230298695406,-0.357518914044833,-0.353499339011814,-0.330618426268376,
-0.324807980341732,-0.303153187730854,-0.286565543897536,-0.280293721896857,
-0.27497512524351,-0.253681437665961,-0.232737497308779,-0.217166132247661,
-0.208374670197327,-0.204725951707223,-0.184285943084061,-0.170452037064309,
-0.14914553243127,-0.139823936654316,-0.135833708541921,-0.132392631416531,
-0.112078350352873,-0.0917069566471694,-0.0716541742035818,-0.067626310494424,
-0.0641204340447217,-0.0443305720467959,-0.0250908100884248,-0.00603170206196263,
-5.00355929031884E-15),.UNSPECIFIED.) ;
#1764=B_SPLINE_CURVE_WITH_KNOTS('',3,(#116394,#116395,#116396,#116397,#116398,
#116399,#116400,#116401,#116402,#116403,#116404,#116405,#116406,#116407,
#116408,#116409,#116410,#116411,#116412,#116413,#116414,#116415,#116416,
#116417,#116418,#116419,#116420,#116421,#116422,#116423,#116424,#116425,
#116426,#116427,#116428,#116429,#116430,#116431,#116432,#116433,#116434,
#116435,#116436,#116437,#116438,#116439,#116440,#116441,#116442,#116443,
#116444,#116445,#116446,#116447,#116448,#116449,#116450,#116451,#116452,
#116453,#116454,#116455,#116456,#116457,#116458,#116459,#116460,#116461,
#116462,#116463,#116464,#116465,#116466,#116467,#116468,#116469,#116470,
#116471,#116472,#116473,#116474,#116475,#116476,#116477,#116478,#116479,
#116480,#116481),.UNSPECIFIED.,.F.,.F.,(4,3,3,3,3,3,3,3,3,3,3,3,3,3,3,3,
3,3,3,3,3,3,3,3,3,3,3,3,3,4),(-0.374020018364427,-0.362349077150302,-0.34056398080081,
-0.33345324485073,-0.328206439767411,-0.323553301020776,-0.301861361668488,
-0.285952048119608,-0.279252129425629,-0.275334282185498,-0.254027310368013,
-0.233103842154587,-0.218474594935304,-0.206338981465346,-0.202820931586694,
-0.182410565592875,-0.174586853277452,-0.153875936134864,-0.143831381828718,
-0.13799507666095,-0.134412923455841,-0.114104327564578,-0.0937141935060995,
-0.0736245310869828,-0.0688062389308537,-0.0640039679130607,-0.0442183910804699,
-0.0247594363974842,-0.00595275431251839,0.),.UNSPECIFIED.) ;
#1765=B_SPLINE_CURVE_WITH_KNOTS('',3,(#116483,#116484,#116485,#116486),
 .UNSPECIFIED.,.F.,.F.,(4,4),(0.,0.0180654173549806),.UNSPECIFIED.) ;
#1766=B_SPLINE_CURVE_WITH_KNOTS('',3,(#116487,#116488,#116489,#116490,#116491,
#116492,#116493,#116494,#116495,#116496,#116497,#116498,#116499,#116500,
#116501,#116502,#116503,#116504,#116505,#116506,#116507,#116508,#116509,
#116510,#116511,#116512,#116513,#116514,#116515,#116516,#116517,#116518,
#116519,#116520,#116521,#116522,#116523,#116524,#116525,#116526,#116527,
#116528,#116529,#116530,#116531,#116532,#116533,#116534,#116535,#116536,
#116537,#116538,#116539,#116540,#116541,#116542,#116543,#116544,#116545,
#116546,#116547,#116548,#116549,#116550,#116551,#116552,#116553,#116554,
#116555,#116556,#116557,#116558,#116559,#116560,#116561,#116562,#116563,
#116564,#116565,#116566,#116567,#116568,#116569,#116570,#116571,#116572,
#116573,#116574,#116575,#116576,#116577),.UNSPECIFIED.,.F.,.F.,(4,3,3,3,
3,3,3,3,3,3,3,3,3,3,3,3,3,3,3,3,3,3,3,3,3,3,3,3,3,3,4),(-0.380169894663632,
-0.365829779172372,-0.346639954767462,-0.338855951704939,-0.33481170502711,
-0.31500122031449,-0.299335348941147,-0.290828675949366,-0.287130866641693,
-0.266780066890063,-0.246135635921242,-0.232029437966579,-0.224974018565242,
-0.220447300081947,-0.217112258820216,-0.196051485500263,-0.189674249327746,
-0.169242036501509,-0.158592891500461,-0.152820666006991,-0.149331434698219,
-0.145470149822495,-0.124229913596774,-0.102989677371053,-0.0814839825252319,
-0.0765643464165228,-0.0730763435899889,-0.0511173678544621,-0.0291950315550003,
-0.00783050913432987,0.),.UNSPECIFIED.) ;
#1767=B_SPLINE_CURVE_WITH_KNOTS('',3,(#116750,#116751,#116752,#116753,#116754,
#116755,#116756,#116757,#116758,#116759,#116760,#116761,#116762,#116763,
#116764,#116765,#116766,#116767,#116768,#116769,#116770,#116771,#116772,
#116773,#116774,#116775,#116776,#116777,#116778,#116779,#116780,#116781,
#116782,#116783,#116784,#116785,#116786,#116787,#116788,#116789,#116790,
#116791,#116792,#116793,#116794,#116795,#116796,#116797,#116798,#116799,
#116800,#116801,#116802,#116803,#116804,#116805,#116806,#116807,#116808,
#116809,#116810,#116811,#116812,#116813,#116814,#116815,#116816,#116817,
#116818,#116819,#116820,#116821,#116822,#116823,#116824,#116825,#116826,
#116827,#116828,#116829,#116830,#116831,#116832,#116833,#116834,#116835,
#116836,#116837,#116838,#116839,#116840),.UNSPECIFIED.,.F.,.F.,(4,3,3,3,
3,3,3,3,3,3,3,3,3,3,3,3,3,3,3,3,3,3,3,3,3,3,3,3,3,3,4),(-0.380169894663596,
-0.365829779172345,-0.346639954384228,-0.338855950466618,-0.334811703196154,
-0.315001218246295,-0.299335347131477,-0.290828672854654,-0.287130864274129,
-0.266780064403244,-0.246147831802541,-0.232029436183843,-0.224974014860838,
-0.220447286668042,-0.217112256507811,-0.196051483279599,-0.189674249327752,
-0.169242036096976,-0.158592891228521,-0.152820665783821,-0.149331432694279,
-0.145470149474333,-0.124229912877894,-0.102989676281454,-0.0814839817255933,
-0.0765643433675259,-0.0730763417070937,-0.0511173658980769,-0.0291950301878927,
-0.00783050936092446,0.),.UNSPECIFIED.) ;
#1768=B_SPLINE_CURVE_WITH_KNOTS('',3,(#116842,#116843,#116844,#116845,#116846,
#116847,#116848,#116849,#116850,#116851,#116852,#116853,#116854,#116855,
#116856,#116857,#116858,#116859,#116860,#116861,#116862,#116863,#116864,
#116865,#116866,#116867,#116868,#116869,#116870,#116871,#116872,#116873,
#116874,#116875,#116876,#116877,#116878,#116879,#116880,#116881,#116882,
#116883,#116884,#116885,#116886,#116887,#116888,#116889,#116890,#116891,
#116892,#116893,#116894,#116895,#116896,#116897,#116898,#116899,#116900,
#116901,#116902,#116903,#116904,#116905,#116906,#116907,#116908,#116909,
#116910,#116911,#116912,#116913,#116914,#116915,#116916,#116917,#116918,
#116919,#116920,#116921,#116922,#116923,#116924,#116925,#116926,#116927,
#116928,#116929),.UNSPECIFIED.,.F.,.F.,(4,3,3,3,3,3,3,3,3,3,3,3,3,3,3,3,
3,3,3,3,3,3,3,3,3,3,3,3,3,4),(-0.374020098293467,-0.362349077150222,-0.340563980758886,
-0.333453244980001,-0.328206442865421,-0.323553301758691,-0.30186136236912,
-0.285952048732665,-0.279252131280905,-0.275334282105171,-0.254027310290031,
-0.233103842618665,-0.218474595283369,-0.206338981920192,-0.202820931774396,
-0.182410566355118,-0.174586853277482,-0.153875936555904,-0.14383138253821,
-0.137995078806115,-0.134412924715841,-0.114130938170206,-0.0938043258732684,
-0.0736245309349631,-0.0688062385263128,-0.0640039679354593,-0.0442183901736035,
-0.0247594340386698,-0.00595275010025783,-2.53963310401108E-15),
 .UNSPECIFIED.) ;
#2115=B_SPLINE_SURFACE_WITH_KNOTS('',3,3,((#115966,#115967,#115968,#115969,
#115970,#115971,#115972,#115973,#115974,#115975,#115976,#115977,#115978,
#115979,#115980,#115981,#115982,#115983,#115984,#115985,#115986,#115987,
#115988,#115989,#115990,#115991,#115992,#115993,#115994,#115995,#115996),
(#115997,#115998,#115999,#116000,#116001,#116002,#116003,#116004,#116005,
#116006,#116007,#116008,#116009,#116010,#116011,#116012,#116013,#116014,
#116015,#116016,#116017,#116018,#116019,#116020,#116021,#116022,#116023,
#116024,#116025,#116026,#116027),(#116028,#116029,#116030,#116031,#116032,
#116033,#116034,#116035,#116036,#116037,#116038,#116039,#116040,#116041,
#116042,#116043,#116044,#116045,#116046,#116047,#116048,#116049,#116050,
#116051,#116052,#116053,#116054,#116055,#116056,#116057,#116058),(#116059,
#116060,#116061,#116062,#116063,#116064,#116065,#116066,#116067,#116068,
#116069,#116070,#116071,#116072,#116073,#116074,#116075,#116076,#116077,
#116078,#116079,#116080,#116081,#116082,#116083,#116084,#116085,#116086,
#116087,#116088,#116089)),.UNSPECIFIED.,.F.,.F.,.F.,(4,4),(4,1,1,1,1,1,
1,1,1,1,1,1,1,1,1,1,1,1,1,1,1,1,1,1,1,1,1,1,4),(-0.000330953812216286,0.0332825271993837),
(8.30276167405401,9.27440145626965,10.2460412384853,11.2176810207009,12.1893208029166,
13.1609605851322,14.1326003673479,15.1042401495635,16.0758799317792,17.0475197139948,
18.0191594962104,18.9907992784261,19.9624390606417,20.9340788428574,21.905718625073,
22.8773584072887,23.8489981895043,24.8206379717199,25.7922777539356,26.7639175361512,
27.7355573183669,28.7071971005825,29.6788368827982,30.6504766650138,31.6221164472294,
32.5937562294451,33.5653960116607,34.5370357938764,35.5090065299042),
 .UNSPECIFIED.) ;
#2116=B_SPLINE_SURFACE_WITH_KNOTS('',3,3,((#116269,#116270,#116271,#116272,
#116273,#116274,#116275,#116276,#116277,#116278,#116279,#116280,#116281,
#116282,#116283,#116284,#116285,#116286,#116287,#116288,#116289,#116290,
#116291,#116292,#116293,#116294,#116295,#116296,#116297,#116298,#116299),
(#116300,#116301,#116302,#116303,#116304,#116305,#116306,#116307,#116308,
#116309,#116310,#116311,#116312,#116313,#116314,#116315,#116316,#116317,
#116318,#116319,#116320,#116321,#116322,#116323,#116324,#116325,#116326,
#116327,#116328,#116329,#116330),(#116331,#116332,#116333,#116334,#116335,
#116336,#116337,#116338,#116339,#116340,#116341,#116342,#116343,#116344,
#116345,#116346,#116347,#116348,#116349,#116350,#116351,#116352,#116353,
#116354,#116355,#116356,#116357,#116358,#116359,#116360,#116361),(#116362,
#116363,#116364,#116365,#116366,#116367,#116368,#116369,#116370,#116371,
#116372,#116373,#116374,#116375,#116376,#116377,#116378,#116379,#116380,
#116381,#116382,#116383,#116384,#116385,#116386,#116387,#116388,#116389,
#116390,#116391,#116392)),.UNSPECIFIED.,.F.,.F.,.F.,(4,4),(4,1,1,1,1,1,
1,1,1,1,1,1,1,1,1,1,1,1,1,1,1,1,1,1,1,1,1,1,4),(-0.000267929854482752,0.0333311607245051),
(11.6148786349143,12.5868540099703,13.5584937921859,14.5301335744016,15.5017733566172,
16.4734131388329,17.4450529210485,18.4166927032641,19.3883324854798,20.3599722676954,
21.3316120499111,22.3032518321267,23.2748916143424,24.246531396558,25.2181711787737,
26.1898109609893,27.161450743205,28.1330905254206,29.1047303076363,30.0763700898519,
31.0480098720675,32.0196496542832,32.9912894364988,33.9629292187145,34.9345690009301,
35.9062087831458,36.8778485653614,37.8494883475771,38.8211281297927),
 .UNSPECIFIED.) ;
#2117=B_SPLINE_SURFACE_WITH_KNOTS('',3,3,((#116578,#116579,#116580,#116581,
#116582,#116583,#116584,#116585,#116586,#116587,#116588,#116589,#116590,
#116591,#116592,#116593,#116594,#116595,#116596,#116597,#116598,#116599,
#116600,#116601,#116602,#116603,#116604,#116605,#116606,#116607,#116608,
#116609,#116610,#116611,#116612,#116613,#116614,#116615,#116616,#116617,
#116618,#116619,#116620),(#116621,#116622,#116623,#116624,#116625,#116626,
#116627,#116628,#116629,#116630,#116631,#116632,#116633,#116634,#116635,
#116636,#116637,#116638,#116639,#116640,#116641,#116642,#116643,#116644,
#116645,#116646,#116647,#116648,#116649,#116650,#116651,#116652,#116653,
#116654,#116655,#116656,#116657,#116658,#116659,#116660,#116661,#116662,
#116663),(#116664,#116665,#116666,#116667,#116668,#116669,#116670,#116671,
#116672,#116673,#116674,#116675,#116676,#116677,#116678,#116679,#116680,
#116681,#116682,#116683,#116684,#116685,#116686,#116687,#116688,#116689,
#116690,#116691,#116692,#116693,#116694,#116695,#116696,#116697,#116698,
#116699,#116700,#116701,#116702,#116703,#116704,#116705,#116706),(#116707,
#116708,#116709,#116710,#116711,#116712,#116713,#116714,#116715,#116716,
#116717,#116718,#116719,#116720,#116721,#116722,#116723,#116724,#116725,
#116726,#116727,#116728,#116729,#116730,#116731,#116732,#116733,#116734,
#116735,#116736,#116737,#116738,#116739,#116740,#116741,#116742,#116743,
#116744,#116745,#116746,#116747,#116748,#116749)),.UNSPECIFIED.,.F.,.F.,
 .F.,(4,4),(4,1,1,1,1,1,1,1,1,1,1,1,1,1,1,1,1,1,1,1,1,1,1,1,1,1,1,1,1,1,
1,1,1,1,1,1,1,1,1,1,4),(-0.00035408581260011,0.0333043091341808),(8.30276167405401,
9.29706878696395,10.2913758998739,11.2856830127838,12.2799901256938,13.2742972386037,
14.2686043515136,15.2629114644236,16.2572185773335,17.2515256902434,18.2458328031534,
19.2401399160633,20.2344470289732,21.2287541418832,22.2230612547931,23.217368367703,
24.211675480613,25.2059825935229,26.2002897064328,27.1945968193428,28.1889039322527,
29.1832110451626,30.1775181580726,31.1718252709825,32.1661323838924,33.1604394968024,
34.1547466097123,35.1490537226222,36.1433608355322,37.1376679484421,38.1319750613521,
39.126282174262,40.1205892871719,41.1148964000819,42.1092035129918,43.1035106259017,
44.0978177388117,45.0921248517216,46.0864319646315,47.0807390775415,48.075400276264),
 .UNSPECIFIED.) ;
#2118=B_SPLINE_SURFACE_WITH_KNOTS('',3,3,((#116930,#116931,#116932,#116933,
#116934,#116935,#116936,#116937,#116938,#116939,#116940,#116941,#116942,
#116943,#116944,#116945,#116946,#116947,#116948,#116949,#116950,#116951,
#116952,#116953,#116954,#116955,#116956,#116957,#116958,#116959,#116960,
#116961,#116962,#116963,#116964,#116965,#116966,#116967,#116968,#116969,
#116970,#116971,#116972),(#116973,#116974,#116975,#116976,#116977,#116978,
#116979,#116980,#116981,#116982,#116983,#116984,#116985,#116986,#116987,
#116988,#116989,#116990,#116991,#116992,#116993,#116994,#116995,#116996,
#116997,#116998,#116999,#117000,#117001,#117002,#117003,#117004,#117005,
#117006,#117007,#117008,#117009,#117010,#117011,#117012,#117013,#117014,
#117015),(#117016,#117017,#117018,#117019,#117020,#117021,#117022,#117023,
#117024,#117025,#117026,#117027,#117028,#117029,#117030,#117031,#117032,
#117033,#117034,#117035,#117036,#117037,#117038,#117039,#117040,#117041,
#117042,#117043,#117044,#117045,#117046,#117047,#117048,#117049,#117050,
#117051,#117052,#117053,#117054,#117055,#117056,#117057,#117058),(#117059,
#117060,#117061,#117062,#117063,#117064,#117065,#117066,#117067,#117068,
#117069,#117070,#117071,#117072,#117073,#117074,#117075,#117076,#117077,
#117078,#117079,#117080,#117081,#117082,#117083,#117084,#117085,#117086,
#117087,#117088,#117089,#117090,#117091,#117092,#117093,#117094,#117095,
#117096,#117097,#117098,#117099,#117100,#117101)),.UNSPECIFIED.,.F.,.F.,
 .F.,(4,4),(4,1,1,1,1,1,1,1,1,1,1,1,1,1,1,1,1,1,1,1,1,1,1,1,1,1,1,1,1,1,
1,1,1,1,1,1,1,1,1,1,4),(-0.00029211499150135,0.0333604038950206),(11.6148493917438,
12.6095213406646,13.6038284535745,14.5981355664844,15.5924426793944,16.5867497923043,
17.5810569052142,18.5753640181242,19.5696711310341,20.563978243944,21.558285356854,
22.5525924697639,23.5468995826738,24.5412066955838,25.5355138084937,26.5298209214036,
27.5241280343136,28.5184351472235,29.5127422601335,30.5070493730434,31.5013564859533,
32.4956635988633,33.4899707117732,34.4842778246831,35.4785849375931,36.472892050503,
37.4671991634129,38.4615062763229,39.4558133892328,40.4501205021427,41.4444276150527,
42.4387347279626,43.4330418408725,44.4273489537825,45.4216560666924,46.4159631796023,
47.4102702925123,48.4045774054222,49.3988845183321,50.3931916312421,51.387498744152),
 .UNSPECIFIED.) ;
#3026=PLANE('',#55070) ;
#3027=PLANE('',#55071) ;
#3028=PLANE('',#55072) ;
#3029=PLANE('',#55073) ;
#3030=PLANE('',#55074) ;
#3031=PLANE('',#55075) ;
#6236=LINE('',#109201,#9450) ;
#6237=LINE('',#109336,#9451) ;
#6238=LINE('',#109624,#9452) ;
#6239=LINE('',#109747,#9453) ;
#6240=LINE('',#109983,#9454) ;
#6241=LINE('',#110144,#9455) ;
#6242=LINE('',#110479,#9456) ;
#6243=LINE('',#110813,#9457) ;
#6244=LINE('',#111144,#9458) ;
#6245=LINE('',#111472,#9459) ;
#9450=VECTOR('',#69777,1.67774999999999) ;
#9451=VECTOR('',#69782,1.67774999999999) ;
#9452=VECTOR('',#69785,1.67774999999999) ;
#9453=VECTOR('',#69788,1.67774999999999) ;
#9454=VECTOR('',#69791,1.67774999999999) ;
#9455=VECTOR('',#69796,1.67774999999999) ;
#9456=VECTOR('',#69799,1.67774999999999) ;
#9457=VECTOR('',#69802,1.67774999999999) ;
#9458=VECTOR('',#69805,1.67774999999999) ;
#9459=VECTOR('',#69808,1.67774999999999) ;
#10734=CYLINDRICAL_SURFACE('',#55047,1.67774999999999) ;
#10735=CYLINDRICAL_SURFACE('',#55049,1.67774999999999) ;
#10736=CYLINDRICAL_SURFACE('',#55050,1.67774999999999) ;
#10737=CYLINDRICAL_SURFACE('',#55051,1.67774999999999) ;
#10738=CYLINDRICAL_SURFACE('',#55052,1.67774999999999) ;
#10739=CYLINDRICAL_SURFACE('',#55054,1.67774999999999) ;
#10740=CYLINDRICAL_SURFACE('',#55055,1.67774999999999) ;
#10741=CYLINDRICAL_SURFACE('',#55056,1.67774999999999) ;
#10742=CYLINDRICAL_SURFACE('',#55057,1.67774999999999) ;
#10743=CYLINDRICAL_SURFACE('',#55058,1.67774999999999) ;
#10744=CYLINDRICAL_SURFACE('',#55059,1.9635) ;
#10745=CYLINDRICAL_SURFACE('',#55066,1.67774999999999) ;
#10746=CYLINDRICAL_SURFACE('',#55068,1.67774999999999) ;
#13816=FACE_OUTER_BOUND('',#17008,.T.) ;
#13817=FACE_OUTER_BOUND('',#17009,.T.) ;
#13818=FACE_OUTER_BOUND('',#17010,.T.) ;
#13819=FACE_OUTER_BOUND('',#17011,.T.) ;
#13820=FACE_OUTER_BOUND('',#17012,.T.) ;
#13821=FACE_OUTER_BOUND('',#17013,.T.) ;
#13822=FACE_OUTER_BOUND('',#17014,.T.) ;
#13823=FACE_OUTER_BOUND('',#17015,.T.) ;
#13824=FACE_OUTER_BOUND('',#17016,.T.) ;
#13825=FACE_OUTER_BOUND('',#17017,.T.) ;
#13826=FACE_OUTER_BOUND('',#17018,.T.) ;
#13827=FACE_OUTER_BOUND('',#17022,.T.) ;
#13828=FACE_OUTER_BOUND('',#17023,.T.) ;
#13829=FACE_OUTER_BOUND('',#17024,.T.) ;
#13830=FACE_OUTER_BOUND('',#17025,.T.) ;
#13831=FACE_OUTER_BOUND('',#17026,.T.) ;
#13832=FACE_OUTER_BOUND('',#17027,.T.) ;
#13833=FACE_OUTER_BOUND('',#17028,.T.) ;
#13834=FACE_OUTER_BOUND('',#17029,.T.) ;
#13835=FACE_OUTER_BOUND('',#17030,.T.) ;
#13836=FACE_OUTER_BOUND('',#17031,.T.) ;
#13837=FACE_OUTER_BOUND('',#17032,.T.) ;
#13838=FACE_OUTER_BOUND('',#17033,.T.) ;
#17008=EDGE_LOOP('',(#45248,#45249,#45250,#45251)) ;
#17009=EDGE_LOOP('',(#45252,#45253,#45254,#45255)) ;
#17010=EDGE_LOOP('',(#45256,#45257,#45258,#45259,#45260,#45261)) ;
#17011=EDGE_LOOP('',(#45262,#45263,#45264,#45265,#45266,#45267)) ;
#17012=EDGE_LOOP('',(#45268,#45269,#45270,#45271)) ;
#17013=EDGE_LOOP('',(#45272,#45273,#45274,#45275,#45276)) ;
#17014=EDGE_LOOP('',(#45277,#45278,#45279,#45280)) ;
#17015=EDGE_LOOP('',(#45281,#45282,#45283,#45284,#45285)) ;
#17016=EDGE_LOOP('',(#45286,#45287,#45288,#45289)) ;
#17017=EDGE_LOOP('',(#45290,#45291,#45292,#45293,#45294)) ;
#17018=EDGE_LOOP('',(#45295)) ;
#17019=EDGE_LOOP('',(#45296,#45297,#45298,#45299,#45300,#45301,#45302,#45303,
#45304,#45305,#45306,#45307,#45308,#45309)) ;
#17020=EDGE_LOOP('',(#45310,#45311,#45312,#45313,#45314,#45315,#45316,#45317,
#45318,#45319,#45320,#45321,#45322,#45323,#45324,#45325,#45326,#45327)) ;
#17021=EDGE_LOOP('',(#45328)) ;
#17022=EDGE_LOOP('',(#45329,#45330,#45331,#45332,#45333)) ;
#17023=EDGE_LOOP('',(#45334,#45335,#45336,#45337,#45338)) ;
#17024=EDGE_LOOP('',(#45339,#45340,#45341,#45342,#45343)) ;
#17025=EDGE_LOOP('',(#45344,#45345,#45346,#45347,#45348,#45349,#45350,#45351,
#45352,#45353,#45354,#45355,#45356,#45357,#45358,#45359,#45360)) ;
#17026=EDGE_LOOP('',(#45361,#45362,#45363,#45364,#45365)) ;
#17027=EDGE_LOOP('',(#45366,#45367,#45368,#45369,#45370,#45371,#45372,#45373,
#45374,#45375,#45376,#45377,#45378,#45379,#45380,#45381)) ;
#17028=EDGE_LOOP('',(#45382,#45383,#45384,#45385,#45386)) ;
#17029=EDGE_LOOP('',(#45387,#45388,#45389,#45390,#45391,#45392,#45393,#45394,
#45395,#45396,#45397,#45398,#45399,#45400,#45401,#45402,#45403,#45404,#45405,
#45406,#45407)) ;
#17030=EDGE_LOOP('',(#45408,#45409,#45410,#45411)) ;
#17031=EDGE_LOOP('',(#45412,#45413,#45414,#45415,#45416,#45417,#45418,#45419,
#45420,#45421,#45422,#45423,#45424,#45425,#45426,#45427,#45428,#45429)) ;
#17032=EDGE_LOOP('',(#45430)) ;
#17033=EDGE_LOOP('',(#45431)) ;
#19551=CIRCLE('',#55048,1.67774999999999) ;
#19552=CIRCLE('',#55053,1.67774999999999) ;
#19553=CIRCLE('',#55060,1.9635) ;
#19554=CIRCLE('',#55061,1.9635) ;
#19555=CIRCLE('',#55062,1.9635) ;
#19556=CIRCLE('',#55063,1.9635) ;
#19557=CIRCLE('',#55064,1.9635) ;
#19558=CIRCLE('',#55065,1.9635) ;
#19559=CIRCLE('',#55067,1.67774999999999) ;
#19560=CIRCLE('',#55069,1.67774999999999) ;
#23701=VERTEX_POINT('',#109199) ;
#23702=VERTEX_POINT('',#109200) ;
#23703=VERTEX_POINT('',#109202) ;
#23704=VERTEX_POINT('',#109283) ;
#23705=VERTEX_POINT('',#109334) ;
#23706=VERTEX_POINT('',#109335) ;
#23707=VERTEX_POINT('',#109622) ;
#23708=VERTEX_POINT('',#109623) ;
#23709=VERTEX_POINT('',#109625) ;
#23710=VERTEX_POINT('',#109688) ;
#23711=VERTEX_POINT('',#109745) ;
#23712=VERTEX_POINT('',#109746) ;
#23713=VERTEX_POINT('',#109748) ;
#23714=VERTEX_POINT('',#109873) ;
#23715=VERTEX_POINT('',#109981) ;
#23716=VERTEX_POINT('',#109982) ;
#23717=VERTEX_POINT('',#109984) ;
#23718=VERTEX_POINT('',#110079) ;
#23719=VERTEX_POINT('',#110142) ;
#23720=VERTEX_POINT('',#110143) ;
#23721=VERTEX_POINT('',#110145) ;
#23722=VERTEX_POINT('',#110477) ;
#23723=VERTEX_POINT('',#110478) ;
#23724=VERTEX_POINT('',#110811) ;
#23725=VERTEX_POINT('',#110812) ;
#23726=VERTEX_POINT('',#110814) ;
#23727=VERTEX_POINT('',#111142) ;
#23728=VERTEX_POINT('',#111143) ;
#23729=VERTEX_POINT('',#111470) ;
#23730=VERTEX_POINT('',#111471) ;
#23731=VERTEX_POINT('',#111473) ;
#23732=VERTEX_POINT('',#111810) ;
#23733=VERTEX_POINT('',#111812) ;
#23734=VERTEX_POINT('',#111813) ;
#23735=VERTEX_POINT('',#111815) ;
#23736=VERTEX_POINT('',#111824) ;
#23737=VERTEX_POINT('',#112018) ;
#23738=VERTEX_POINT('',#112212) ;
#23739=VERTEX_POINT('',#112409) ;
#23740=VERTEX_POINT('',#112471) ;
#23741=VERTEX_POINT('',#112476) ;
#23742=VERTEX_POINT('',#112478) ;
#23743=VERTEX_POINT('',#112484) ;
#23744=VERTEX_POINT('',#112678) ;
#23745=VERTEX_POINT('',#112875) ;
#23746=VERTEX_POINT('',#113069) ;
#23747=VERTEX_POINT('',#113231) ;
#23748=VERTEX_POINT('',#113232) ;
#23749=VERTEX_POINT('',#113234) ;
#23750=VERTEX_POINT('',#113243) ;
#23751=VERTEX_POINT('',#113434) ;
#23752=VERTEX_POINT('',#113625) ;
#23753=VERTEX_POINT('',#113816) ;
#23754=VERTEX_POINT('',#114010) ;
#23755=VERTEX_POINT('',#114201) ;
#23756=VERTEX_POINT('',#114263) ;
#23757=VERTEX_POINT('',#114268) ;
#23758=VERTEX_POINT('',#114270) ;
#23759=VERTEX_POINT('',#114276) ;
#23760=VERTEX_POINT('',#114467) ;
#23761=VERTEX_POINT('',#114658) ;
#23762=VERTEX_POINT('',#114849) ;
#23763=VERTEX_POINT('',#115040) ;
#23764=VERTEX_POINT('',#115231) ;
#23765=VERTEX_POINT('',#115393) ;
#23766=VERTEX_POINT('',#115396) ;
#23767=VERTEX_POINT('',#115505) ;
#23768=VERTEX_POINT('',#115507) ;
#23769=VERTEX_POINT('',#115598) ;
#23770=VERTEX_POINT('',#115695) ;
#23771=VERTEX_POINT('',#115697) ;
#23772=VERTEX_POINT('',#115873) ;
#23773=VERTEX_POINT('',#116090) ;
#23774=VERTEX_POINT('',#116482) ;
#30902=EDGE_CURVE('',#23701,#23702,#6236,.T.) ;
#30903=EDGE_CURVE('',#23703,#23701,#1697,.F.) ;
#30904=EDGE_CURVE('',#23704,#23703,#19551,.T.) ;
#30905=EDGE_CURVE('',#23704,#23702,#1698,.T.) ;
#30906=EDGE_CURVE('',#23705,#23706,#6237,.T.) ;
#30907=EDGE_CURVE('',#23701,#23705,#1699,.F.) ;
#30908=EDGE_CURVE('',#23702,#23706,#1700,.T.) ;
#30909=EDGE_CURVE('',#23707,#23708,#6238,.T.) ;
#30910=EDGE_CURVE('',#23709,#23707,#1701,.T.) ;
#30911=EDGE_CURVE('',#23705,#23709,#1702,.F.) ;
#30912=EDGE_CURVE('',#23706,#23710,#1703,.T.) ;
#30913=EDGE_CURVE('',#23710,#23708,#1704,.T.) ;
#30914=EDGE_CURVE('',#23711,#23712,#6239,.T.) ;
#30915=EDGE_CURVE('',#23713,#23711,#1705,.T.) ;
#30916=EDGE_CURVE('',#23707,#23713,#1706,.T.) ;
#30917=EDGE_CURVE('',#23708,#23714,#1707,.T.) ;
#30918=EDGE_CURVE('',#23714,#23712,#1708,.F.) ;
#30919=EDGE_CURVE('',#23715,#23716,#6240,.T.) ;
#30920=EDGE_CURVE('',#23717,#23715,#1709,.T.) ;
#30921=EDGE_CURVE('',#23718,#23717,#19552,.T.) ;
#30922=EDGE_CURVE('',#23718,#23716,#1710,.T.) ;
#30923=EDGE_CURVE('',#23719,#23720,#6241,.T.) ;
#30924=EDGE_CURVE('',#23721,#23719,#1711,.F.) ;
#30925=EDGE_CURVE('',#23715,#23721,#1712,.T.) ;
#30926=EDGE_CURVE('',#23716,#23720,#1713,.T.) ;
#30927=EDGE_CURVE('',#23722,#23723,#6242,.T.) ;
#30928=EDGE_CURVE('',#23719,#23722,#1714,.F.) ;
#30929=EDGE_CURVE('',#23720,#23723,#1715,.T.) ;
#30930=EDGE_CURVE('',#23724,#23725,#6243,.T.) ;
#30931=EDGE_CURVE('',#23726,#23724,#1716,.F.) ;
#30932=EDGE_CURVE('',#23722,#23726,#1717,.F.) ;
#30933=EDGE_CURVE('',#23723,#23725,#1718,.T.) ;
#30934=EDGE_CURVE('',#23727,#23728,#6244,.T.) ;
#30935=EDGE_CURVE('',#23724,#23727,#1719,.F.) ;
#30936=EDGE_CURVE('',#23725,#23728,#1720,.T.) ;
#30937=EDGE_CURVE('',#23729,#23730,#6245,.T.) ;
#30938=EDGE_CURVE('',#23731,#23729,#1721,.T.) ;
#30939=EDGE_CURVE('',#23727,#23731,#1722,.F.) ;
#30940=EDGE_CURVE('',#23728,#23730,#1723,.T.) ;
#30941=EDGE_CURVE('',#23732,#23732,#19553,.T.) ;
#30942=EDGE_CURVE('',#23733,#23734,#19554,.T.) ;
#30943=EDGE_CURVE('',#23734,#23735,#1724,.T.) ;
#30944=EDGE_CURVE('',#23735,#23736,#1725,.T.) ;
#30945=EDGE_CURVE('',#23736,#23737,#1726,.T.) ;
#30946=EDGE_CURVE('',#23737,#23738,#1727,.T.) ;
#30947=EDGE_CURVE('',#23738,#23739,#1728,.T.) ;
#30948=EDGE_CURVE('',#23739,#23740,#1729,.T.) ;
#30949=EDGE_CURVE('',#23740,#23741,#19555,.T.) ;
#30950=EDGE_CURVE('',#23741,#23742,#1730,.T.) ;
#30951=EDGE_CURVE('',#23742,#23743,#1731,.T.) ;
#30952=EDGE_CURVE('',#23743,#23744,#1732,.T.) ;
#30953=EDGE_CURVE('',#23744,#23745,#1733,.T.) ;
#30954=EDGE_CURVE('',#23745,#23746,#1734,.T.) ;
#30955=EDGE_CURVE('',#23746,#23733,#1735,.T.) ;
#30956=EDGE_CURVE('',#23747,#23748,#19556,.T.) ;
#30957=EDGE_CURVE('',#23748,#23749,#1736,.T.) ;
#30958=EDGE_CURVE('',#23749,#23750,#1737,.T.) ;
#30959=EDGE_CURVE('',#23750,#23751,#1738,.T.) ;
#30960=EDGE_CURVE('',#23751,#23752,#1739,.T.) ;
#30961=EDGE_CURVE('',#23752,#23753,#1740,.T.) ;
#30962=EDGE_CURVE('',#23753,#23754,#1741,.T.) ;
#30963=EDGE_CURVE('',#23754,#23755,#1742,.T.) ;
#30964=EDGE_CURVE('',#23755,#23756,#1743,.T.) ;
#30965=EDGE_CURVE('',#23756,#23757,#19557,.T.) ;
#30966=EDGE_CURVE('',#23757,#23758,#1744,.T.) ;
#30967=EDGE_CURVE('',#23758,#23759,#1745,.T.) ;
#30968=EDGE_CURVE('',#23759,#23760,#1746,.T.) ;
#30969=EDGE_CURVE('',#23760,#23761,#1747,.T.) ;
#30970=EDGE_CURVE('',#23761,#23762,#1748,.T.) ;
#30971=EDGE_CURVE('',#23762,#23763,#1749,.T.) ;
#30972=EDGE_CURVE('',#23763,#23764,#1750,.T.) ;
#30973=EDGE_CURVE('',#23764,#23747,#1751,.T.) ;
#30974=EDGE_CURVE('',#23765,#23765,#19558,.F.) ;
#30975=EDGE_CURVE('',#23730,#23766,#1752,.T.) ;
#30976=EDGE_CURVE('',#23767,#23766,#19559,.T.) ;
#30977=EDGE_CURVE('',#23768,#23767,#1753,.T.) ;
#30978=EDGE_CURVE('',#23729,#23768,#1754,.T.) ;
#30979=EDGE_CURVE('',#23712,#23769,#1755,.F.) ;
#30980=EDGE_CURVE('',#23770,#23769,#19560,.T.) ;
#30981=EDGE_CURVE('',#23771,#23770,#1756,.T.) ;
#30982=EDGE_CURVE('',#23711,#23771,#1757,.T.) ;
#30983=EDGE_CURVE('',#23733,#23770,#1758,.T.) ;
#30984=EDGE_CURVE('',#23769,#23772,#1759,.T.) ;
#30985=EDGE_CURVE('',#23772,#23734,#1760,.T.) ;
#30986=EDGE_CURVE('',#23773,#23741,#1761,.T.) ;
#30987=EDGE_CURVE('',#23773,#23703,#1762,.T.) ;
#30988=EDGE_CURVE('',#23740,#23704,#1763,.T.) ;
#30989=EDGE_CURVE('',#23747,#23767,#1764,.T.) ;
#30990=EDGE_CURVE('',#23766,#23774,#1765,.T.) ;
#30991=EDGE_CURVE('',#23774,#23748,#1766,.T.) ;
#30992=EDGE_CURVE('',#23717,#23757,#1767,.T.) ;
#30993=EDGE_CURVE('',#23756,#23718,#1768,.T.) ;
#45248=ORIENTED_EDGE('',*,*,#30902,.F.) ;
#45249=ORIENTED_EDGE('',*,*,#30903,.F.) ;
#45250=ORIENTED_EDGE('',*,*,#30904,.F.) ;
#45251=ORIENTED_EDGE('',*,*,#30905,.T.) ;
#45252=ORIENTED_EDGE('',*,*,#30906,.F.) ;
#45253=ORIENTED_EDGE('',*,*,#30907,.F.) ;
#45254=ORIENTED_EDGE('',*,*,#30902,.T.) ;
#45255=ORIENTED_EDGE('',*,*,#30908,.T.) ;
#45256=ORIENTED_EDGE('',*,*,#30909,.F.) ;
#45257=ORIENTED_EDGE('',*,*,#30910,.F.) ;
#45258=ORIENTED_EDGE('',*,*,#30911,.F.) ;
#45259=ORIENTED_EDGE('',*,*,#30906,.T.) ;
#45260=ORIENTED_EDGE('',*,*,#30912,.T.) ;
#45261=ORIENTED_EDGE('',*,*,#30913,.T.) ;
#45262=ORIENTED_EDGE('',*,*,#30914,.F.) ;
#45263=ORIENTED_EDGE('',*,*,#30915,.F.) ;
#45264=ORIENTED_EDGE('',*,*,#30916,.F.) ;
#45265=ORIENTED_EDGE('',*,*,#30909,.T.) ;
#45266=ORIENTED_EDGE('',*,*,#30917,.T.) ;
#45267=ORIENTED_EDGE('',*,*,#30918,.T.) ;
#45268=ORIENTED_EDGE('',*,*,#30919,.F.) ;
#45269=ORIENTED_EDGE('',*,*,#30920,.F.) ;
#45270=ORIENTED_EDGE('',*,*,#30921,.F.) ;
#45271=ORIENTED_EDGE('',*,*,#30922,.T.) ;
#45272=ORIENTED_EDGE('',*,*,#30923,.F.) ;
#45273=ORIENTED_EDGE('',*,*,#30924,.F.) ;
#45274=ORIENTED_EDGE('',*,*,#30925,.F.) ;
#45275=ORIENTED_EDGE('',*,*,#30919,.T.) ;
#45276=ORIENTED_EDGE('',*,*,#30926,.T.) ;
#45277=ORIENTED_EDGE('',*,*,#30927,.F.) ;
#45278=ORIENTED_EDGE('',*,*,#30928,.F.) ;
#45279=ORIENTED_EDGE('',*,*,#30923,.T.) ;
#45280=ORIENTED_EDGE('',*,*,#30929,.T.) ;
#45281=ORIENTED_EDGE('',*,*,#30930,.F.) ;
#45282=ORIENTED_EDGE('',*,*,#30931,.F.) ;
#45283=ORIENTED_EDGE('',*,*,#30932,.F.) ;
#45284=ORIENTED_EDGE('',*,*,#30927,.T.) ;
#45285=ORIENTED_EDGE('',*,*,#30933,.T.) ;
#45286=ORIENTED_EDGE('',*,*,#30934,.F.) ;
#45287=ORIENTED_EDGE('',*,*,#30935,.F.) ;
#45288=ORIENTED_EDGE('',*,*,#30930,.T.) ;
#45289=ORIENTED_EDGE('',*,*,#30936,.T.) ;
#45290=ORIENTED_EDGE('',*,*,#30937,.F.) ;
#45291=ORIENTED_EDGE('',*,*,#30938,.F.) ;
#45292=ORIENTED_EDGE('',*,*,#30939,.F.) ;
#45293=ORIENTED_EDGE('',*,*,#30934,.T.) ;
#45294=ORIENTED_EDGE('',*,*,#30940,.T.) ;
#45295=ORIENTED_EDGE('',*,*,#30941,.F.) ;
#45296=ORIENTED_EDGE('',*,*,#30942,.T.) ;
#45297=ORIENTED_EDGE('',*,*,#30943,.T.) ;
#45298=ORIENTED_EDGE('',*,*,#30944,.T.) ;
#45299=ORIENTED_EDGE('',*,*,#30945,.T.) ;
#45300=ORIENTED_EDGE('',*,*,#30946,.T.) ;
#45301=ORIENTED_EDGE('',*,*,#30947,.T.) ;
#45302=ORIENTED_EDGE('',*,*,#30948,.T.) ;
#45303=ORIENTED_EDGE('',*,*,#30949,.T.) ;
#45304=ORIENTED_EDGE('',*,*,#30950,.T.) ;
#45305=ORIENTED_EDGE('',*,*,#30951,.T.) ;
#45306=ORIENTED_EDGE('',*,*,#30952,.T.) ;
#45307=ORIENTED_EDGE('',*,*,#30953,.T.) ;
#45308=ORIENTED_EDGE('',*,*,#30954,.T.) ;
#45309=ORIENTED_EDGE('',*,*,#30955,.T.) ;
#45310=ORIENTED_EDGE('',*,*,#30956,.T.) ;
#45311=ORIENTED_EDGE('',*,*,#30957,.T.) ;
#45312=ORIENTED_EDGE('',*,*,#30958,.T.) ;
#45313=ORIENTED_EDGE('',*,*,#30959,.T.) ;
#45314=ORIENTED_EDGE('',*,*,#30960,.T.) ;
#45315=ORIENTED_EDGE('',*,*,#30961,.T.) ;
#45316=ORIENTED_EDGE('',*,*,#30962,.T.) ;
#45317=ORIENTED_EDGE('',*,*,#30963,.T.) ;
#45318=ORIENTED_EDGE('',*,*,#30964,.T.) ;
#45319=ORIENTED_EDGE('',*,*,#30965,.T.) ;
#45320=ORIENTED_EDGE('',*,*,#30966,.T.) ;
#45321=ORIENTED_EDGE('',*,*,#30967,.T.) ;
#45322=ORIENTED_EDGE('',*,*,#30968,.T.) ;
#45323=ORIENTED_EDGE('',*,*,#30969,.T.) ;
#45324=ORIENTED_EDGE('',*,*,#30970,.T.) ;
#45325=ORIENTED_EDGE('',*,*,#30971,.T.) ;
#45326=ORIENTED_EDGE('',*,*,#30972,.T.) ;
#45327=ORIENTED_EDGE('',*,*,#30973,.T.) ;
#45328=ORIENTED_EDGE('',*,*,#30974,.F.) ;
#45329=ORIENTED_EDGE('',*,*,#30937,.T.) ;
#45330=ORIENTED_EDGE('',*,*,#30975,.T.) ;
#45331=ORIENTED_EDGE('',*,*,#30976,.F.) ;
#45332=ORIENTED_EDGE('',*,*,#30977,.F.) ;
#45333=ORIENTED_EDGE('',*,*,#30978,.F.) ;
#45334=ORIENTED_EDGE('',*,*,#30914,.T.) ;
#45335=ORIENTED_EDGE('',*,*,#30979,.T.) ;
#45336=ORIENTED_EDGE('',*,*,#30980,.F.) ;
#45337=ORIENTED_EDGE('',*,*,#30981,.F.) ;
#45338=ORIENTED_EDGE('',*,*,#30982,.F.) ;
#45339=ORIENTED_EDGE('',*,*,#30942,.F.) ;
#45340=ORIENTED_EDGE('',*,*,#30983,.T.) ;
#45341=ORIENTED_EDGE('',*,*,#30980,.T.) ;
#45342=ORIENTED_EDGE('',*,*,#30984,.T.) ;
#45343=ORIENTED_EDGE('',*,*,#30985,.T.) ;
#45344=ORIENTED_EDGE('',*,*,#30983,.F.) ;
#45345=ORIENTED_EDGE('',*,*,#30955,.F.) ;
#45346=ORIENTED_EDGE('',*,*,#30954,.F.) ;
#45347=ORIENTED_EDGE('',*,*,#30953,.F.) ;
#45348=ORIENTED_EDGE('',*,*,#30952,.F.) ;
#45349=ORIENTED_EDGE('',*,*,#30951,.F.) ;
#45350=ORIENTED_EDGE('',*,*,#30950,.F.) ;
#45351=ORIENTED_EDGE('',*,*,#30986,.F.) ;
#45352=ORIENTED_EDGE('',*,*,#30987,.T.) ;
#45353=ORIENTED_EDGE('',*,*,#30903,.T.) ;
#45354=ORIENTED_EDGE('',*,*,#30907,.T.) ;
#45355=ORIENTED_EDGE('',*,*,#30911,.T.) ;
#45356=ORIENTED_EDGE('',*,*,#30910,.T.) ;
#45357=ORIENTED_EDGE('',*,*,#30916,.T.) ;
#45358=ORIENTED_EDGE('',*,*,#30915,.T.) ;
#45359=ORIENTED_EDGE('',*,*,#30982,.T.) ;
#45360=ORIENTED_EDGE('',*,*,#30981,.T.) ;
#45361=ORIENTED_EDGE('',*,*,#30949,.F.) ;
#45362=ORIENTED_EDGE('',*,*,#30988,.T.) ;
#45363=ORIENTED_EDGE('',*,*,#30904,.T.) ;
#45364=ORIENTED_EDGE('',*,*,#30987,.F.) ;
#45365=ORIENTED_EDGE('',*,*,#30986,.T.) ;
#45366=ORIENTED_EDGE('',*,*,#30985,.F.) ;
#45367=ORIENTED_EDGE('',*,*,#30984,.F.) ;
#45368=ORIENTED_EDGE('',*,*,#30979,.F.) ;
#45369=ORIENTED_EDGE('',*,*,#30918,.F.) ;
#45370=ORIENTED_EDGE('',*,*,#30917,.F.) ;
#45371=ORIENTED_EDGE('',*,*,#30913,.F.) ;
#45372=ORIENTED_EDGE('',*,*,#30912,.F.) ;
#45373=ORIENTED_EDGE('',*,*,#30908,.F.) ;
#45374=ORIENTED_EDGE('',*,*,#30905,.F.) ;
#45375=ORIENTED_EDGE('',*,*,#30988,.F.) ;
#45376=ORIENTED_EDGE('',*,*,#30948,.F.) ;
#45377=ORIENTED_EDGE('',*,*,#30947,.F.) ;
#45378=ORIENTED_EDGE('',*,*,#30946,.F.) ;
#45379=ORIENTED_EDGE('',*,*,#30945,.F.) ;
#45380=ORIENTED_EDGE('',*,*,#30944,.F.) ;
#45381=ORIENTED_EDGE('',*,*,#30943,.F.) ;
#45382=ORIENTED_EDGE('',*,*,#30956,.F.) ;
#45383=ORIENTED_EDGE('',*,*,#30989,.T.) ;
#45384=ORIENTED_EDGE('',*,*,#30976,.T.) ;
#45385=ORIENTED_EDGE('',*,*,#30990,.T.) ;
#45386=ORIENTED_EDGE('',*,*,#30991,.T.) ;
#45387=ORIENTED_EDGE('',*,*,#30989,.F.) ;
#45388=ORIENTED_EDGE('',*,*,#30973,.F.) ;
#45389=ORIENTED_EDGE('',*,*,#30972,.F.) ;
#45390=ORIENTED_EDGE('',*,*,#30971,.F.) ;
#45391=ORIENTED_EDGE('',*,*,#30970,.F.) ;
#45392=ORIENTED_EDGE('',*,*,#30969,.F.) ;
#45393=ORIENTED_EDGE('',*,*,#30968,.F.) ;
#45394=ORIENTED_EDGE('',*,*,#30967,.F.) ;
#45395=ORIENTED_EDGE('',*,*,#30966,.F.) ;
#45396=ORIENTED_EDGE('',*,*,#30992,.F.) ;
#45397=ORIENTED_EDGE('',*,*,#30920,.T.) ;
#45398=ORIENTED_EDGE('',*,*,#30925,.T.) ;
#45399=ORIENTED_EDGE('',*,*,#30924,.T.) ;
#45400=ORIENTED_EDGE('',*,*,#30928,.T.) ;
#45401=ORIENTED_EDGE('',*,*,#30932,.T.) ;
#45402=ORIENTED_EDGE('',*,*,#30931,.T.) ;
#45403=ORIENTED_EDGE('',*,*,#30935,.T.) ;
#45404=ORIENTED_EDGE('',*,*,#30939,.T.) ;
#45405=ORIENTED_EDGE('',*,*,#30938,.T.) ;
#45406=ORIENTED_EDGE('',*,*,#30978,.T.) ;
#45407=ORIENTED_EDGE('',*,*,#30977,.T.) ;
#45408=ORIENTED_EDGE('',*,*,#30965,.F.) ;
#45409=ORIENTED_EDGE('',*,*,#30993,.T.) ;
#45410=ORIENTED_EDGE('',*,*,#30921,.T.) ;
#45411=ORIENTED_EDGE('',*,*,#30992,.T.) ;
#45412=ORIENTED_EDGE('',*,*,#30991,.F.) ;
#45413=ORIENTED_EDGE('',*,*,#30990,.F.) ;
#45414=ORIENTED_EDGE('',*,*,#30975,.F.) ;
#45415=ORIENTED_EDGE('',*,*,#30940,.F.) ;
#45416=ORIENTED_EDGE('',*,*,#30936,.F.) ;
#45417=ORIENTED_EDGE('',*,*,#30933,.F.) ;
#45418=ORIENTED_EDGE('',*,*,#30929,.F.) ;
#45419=ORIENTED_EDGE('',*,*,#30926,.F.) ;
#45420=ORIENTED_EDGE('',*,*,#30922,.F.) ;
#45421=ORIENTED_EDGE('',*,*,#30993,.F.) ;
#45422=ORIENTED_EDGE('',*,*,#30964,.F.) ;
#45423=ORIENTED_EDGE('',*,*,#30963,.F.) ;
#45424=ORIENTED_EDGE('',*,*,#30962,.F.) ;
#45425=ORIENTED_EDGE('',*,*,#30961,.F.) ;
#45426=ORIENTED_EDGE('',*,*,#30960,.F.) ;
#45427=ORIENTED_EDGE('',*,*,#30959,.F.) ;
#45428=ORIENTED_EDGE('',*,*,#30958,.F.) ;
#45429=ORIENTED_EDGE('',*,*,#30957,.F.) ;
#45430=ORIENTED_EDGE('',*,*,#30941,.T.) ;
#45431=ORIENTED_EDGE('',*,*,#30974,.T.) ;
#49034=ADVANCED_FACE('',(#13816),#10734,.T.) ;
#49035=ADVANCED_FACE('',(#13817),#10735,.T.) ;
#49036=ADVANCED_FACE('',(#13818),#10736,.T.) ;
#49037=ADVANCED_FACE('',(#13819),#10737,.T.) ;
#49038=ADVANCED_FACE('',(#13820),#10738,.T.) ;
#49039=ADVANCED_FACE('',(#13821),#10739,.T.) ;
#49040=ADVANCED_FACE('',(#13822),#10740,.T.) ;
#49041=ADVANCED_FACE('',(#13823),#10741,.T.) ;
#49042=ADVANCED_FACE('',(#13824),#10742,.T.) ;
#49043=ADVANCED_FACE('',(#13825),#10743,.T.) ;
#49044=ADVANCED_FACE('',(#13826,#770,#771,#772),#10744,.T.) ;
#49045=ADVANCED_FACE('',(#13827),#10745,.T.) ;
#49046=ADVANCED_FACE('',(#13828),#10746,.T.) ;
#49047=ADVANCED_FACE('',(#13829),#3026,.T.) ;
#49048=ADVANCED_FACE('',(#13830),#2115,.F.) ;
#49049=ADVANCED_FACE('',(#13831),#3027,.F.) ;
#49050=ADVANCED_FACE('',(#13832),#2116,.F.) ;
#49051=ADVANCED_FACE('',(#13833),#3028,.T.) ;
#49052=ADVANCED_FACE('',(#13834),#2117,.F.) ;
#49053=ADVANCED_FACE('',(#13835),#3029,.F.) ;
#49054=ADVANCED_FACE('',(#13836),#2118,.F.) ;
#49055=ADVANCED_FACE('',(#13837),#3030,.F.) ;
#49056=ADVANCED_FACE('',(#13838),#3031,.T.) ;
#49077=CLOSED_SHELL('',(#49034,#49035,#49036,#49037,#49038,#49039,#49040,
#49041,#49042,#49043,#49044,#49045,#49046,#49047,#49048,#49049,#49050,#49051,
#49052,#49053,#49054,#49055,#49056)) ;
#55046=AXIS2_PLACEMENT_3D('',#109197,#69773,#69774) ;
#55047=AXIS2_PLACEMENT_3D('',#109198,#69775,#69776) ;
#55048=AXIS2_PLACEMENT_3D('',#109284,#69778,#69779) ;
#55049=AXIS2_PLACEMENT_3D('',#109333,#69780,#69781) ;
#55050=AXIS2_PLACEMENT_3D('',#109621,#69783,#69784) ;
#55051=AXIS2_PLACEMENT_3D('',#109744,#69786,#69787) ;
#55052=AXIS2_PLACEMENT_3D('',#109980,#69789,#69790) ;
#55053=AXIS2_PLACEMENT_3D('',#110080,#69792,#69793) ;
#55054=AXIS2_PLACEMENT_3D('',#110141,#69794,#69795) ;
#55055=AXIS2_PLACEMENT_3D('',#110476,#69797,#69798) ;
#55056=AXIS2_PLACEMENT_3D('',#110810,#69800,#69801) ;
#55057=AXIS2_PLACEMENT_3D('',#111141,#69803,#69804) ;
#55058=AXIS2_PLACEMENT_3D('',#111469,#69806,#69807) ;
#55059=AXIS2_PLACEMENT_3D('',#111809,#69809,#69810) ;
#55060=AXIS2_PLACEMENT_3D('',#111811,#69811,#69812) ;
#55061=AXIS2_PLACEMENT_3D('',#111814,#69813,#69814) ;
#55062=AXIS2_PLACEMENT_3D('',#112477,#69815,#69816) ;
#55063=AXIS2_PLACEMENT_3D('',#113233,#69817,#69818) ;
#55064=AXIS2_PLACEMENT_3D('',#114269,#69819,#69820) ;
#55065=AXIS2_PLACEMENT_3D('',#115394,#69821,#69822) ;
#55066=AXIS2_PLACEMENT_3D('',#115395,#69823,#69824) ;
#55067=AXIS2_PLACEMENT_3D('',#115506,#69825,#69826) ;
#55068=AXIS2_PLACEMENT_3D('',#115597,#69827,#69828) ;
#55069=AXIS2_PLACEMENT_3D('',#115696,#69829,#69830) ;
#55070=AXIS2_PLACEMENT_3D('',#115787,#69831,#69832) ;
#55071=AXIS2_PLACEMENT_3D('',#116183,#69833,#69834) ;
#55072=AXIS2_PLACEMENT_3D('',#116393,#69835,#69836) ;
#55073=AXIS2_PLACEMENT_3D('',#116841,#69837,#69838) ;
#55074=AXIS2_PLACEMENT_3D('',#117102,#69839,#69840) ;
#55075=AXIS2_PLACEMENT_3D('',#117103,#69841,#69842) ;
#69773=DIRECTION('axis',(0.,0.,1.)) ;
#69774=DIRECTION('refdir',(1.,0.,0.)) ;
#69775=DIRECTION('center_axis',(-1.,0.,0.)) ;
#69776=DIRECTION('ref_axis',(0.,0.45781237757936,-0.889048832705568)) ;
#69777=DIRECTION('',(1.,0.,0.)) ;
#69778=DIRECTION('center_axis',(1.,0.,0.)) ;
#69779=DIRECTION('ref_axis',(0.,-1.,5.29386630725752E-15)) ;
#69780=DIRECTION('center_axis',(-1.,0.,0.)) ;
#69781=DIRECTION('ref_axis',(0.,0.45781237757936,-0.889048832705568)) ;
#69782=DIRECTION('',(1.,0.,0.)) ;
#69783=DIRECTION('center_axis',(-1.,0.,0.)) ;
#69784=DIRECTION('ref_axis',(0.,0.45781237757936,-0.889048832705568)) ;
#69785=DIRECTION('',(1.,0.,0.)) ;
#69786=DIRECTION('center_axis',(-1.,0.,0.)) ;
#69787=DIRECTION('ref_axis',(0.,0.45781237757936,-0.889048832705568)) ;
#69788=DIRECTION('',(1.,0.,0.)) ;
#69789=DIRECTION('center_axis',(-1.,0.,0.)) ;
#69790=DIRECTION('ref_axis',(0.,0.457902639548171,-0.889002346844381)) ;
#69791=DIRECTION('',(1.,0.,0.)) ;
#69792=DIRECTION('center_axis',(1.,0.,0.)) ;
#69793=DIRECTION('ref_axis',(0.,-1.,5.29386630725752E-15)) ;
#69794=DIRECTION('center_axis',(-1.,0.,0.)) ;
#69795=DIRECTION('ref_axis',(0.,0.457902639548171,-0.889002346844381)) ;
#69796=DIRECTION('',(1.,0.,0.)) ;
#69797=DIRECTION('center_axis',(-1.,0.,0.)) ;
#69798=DIRECTION('ref_axis',(0.,0.457902639548171,-0.889002346844381)) ;
#69799=DIRECTION('',(1.,0.,0.)) ;
#69800=DIRECTION('center_axis',(-1.,0.,0.)) ;
#69801=DIRECTION('ref_axis',(0.,0.457902639548171,-0.889002346844381)) ;
#69802=DIRECTION('',(1.,0.,0.)) ;
#69803=DIRECTION('center_axis',(-1.,0.,0.)) ;
#69804=DIRECTION('ref_axis',(0.,0.457902639548171,-0.889002346844381)) ;
#69805=DIRECTION('',(1.,0.,0.)) ;
#69806=DIRECTION('center_axis',(-1.,0.,0.)) ;
#69807=DIRECTION('ref_axis',(0.,0.457902639548171,-0.889002346844381)) ;
#69808=DIRECTION('',(1.,0.,0.)) ;
#69809=DIRECTION('center_axis',(-1.,0.,0.)) ;
#69810=DIRECTION('ref_axis',(0.,-1.,0.)) ;
#69811=DIRECTION('center_axis',(1.,0.,0.)) ;
#69812=DIRECTION('ref_axis',(0.,-1.,0.)) ;
#69813=DIRECTION('center_axis',(-1.,0.,0.)) ;
#69814=DIRECTION('ref_axis',(0.,-1.,0.)) ;
#69815=DIRECTION('center_axis',(1.,0.,0.)) ;
#69816=DIRECTION('ref_axis',(0.,-1.,0.)) ;
#69817=DIRECTION('center_axis',(-1.,0.,0.)) ;
#69818=DIRECTION('ref_axis',(0.,-1.,0.)) ;
#69819=DIRECTION('center_axis',(1.,0.,0.)) ;
#69820=DIRECTION('ref_axis',(0.,-1.,0.)) ;
#69821=DIRECTION('center_axis',(1.,0.,0.)) ;
#69822=DIRECTION('ref_axis',(0.,-1.,0.)) ;
#69823=DIRECTION('center_axis',(-1.,0.,0.)) ;
#69824=DIRECTION('ref_axis',(0.,0.457902639548171,-0.889002346844381)) ;
#69825=DIRECTION('center_axis',(-1.,0.,0.)) ;
#69826=DIRECTION('ref_axis',(0.,-1.,5.29386630725752E-15)) ;
#69827=DIRECTION('center_axis',(-1.,0.,0.)) ;
#69828=DIRECTION('ref_axis',(0.,0.45781237757936,-0.889048832705568)) ;
#69829=DIRECTION('center_axis',(-1.,0.,0.)) ;
#69830=DIRECTION('ref_axis',(0.,-1.,5.29386630725752E-15)) ;
#69831=DIRECTION('center_axis',(1.,0.,0.)) ;
#69832=DIRECTION('ref_axis',(0.,0.,-1.)) ;
#69833=DIRECTION('center_axis',(1.,0.,0.)) ;
#69834=DIRECTION('ref_axis',(0.,0.,-1.)) ;
#69835=DIRECTION('center_axis',(1.,0.,0.)) ;
#69836=DIRECTION('ref_axis',(0.,0.,-1.)) ;
#69837=DIRECTION('center_axis',(1.,0.,0.)) ;
#69838=DIRECTION('ref_axis',(0.,0.,-1.)) ;
#69839=DIRECTION('center_axis',(-1.,0.,0.)) ;
#69840=DIRECTION('ref_axis',(0.,-1.,0.)) ;
#69841=DIRECTION('center_axis',(-1.,0.,0.)) ;
#69842=DIRECTION('ref_axis',(0.,-1.,0.)) ;
#109197=CARTESIAN_POINT('',(0.,0.,0.)) ;
#109198=CARTESIAN_POINT('Origin',(67.8645744874958,248.040265107786,23.0213203435596)) ;
#109199=CARTESIAN_POINT('',(66.6775101468938,247.272170391243,24.5129220226009)) ;
#109200=CARTESIAN_POINT('',(66.7760547678839,247.272170398758,24.5129220264705)) ;
#109201=CARTESIAN_POINT('',(67.8645744874958,247.272170391302,24.5129220226314)) ;
#109202=CARTESIAN_POINT('',(66.9402651077865,248.99748421711,21.6434318722943)) ;
#109203=CARTESIAN_POINT('Ctrl Pts',(66.6775101468938,247.272170391243,24.5129220226009)) ;
#109204=CARTESIAN_POINT('Ctrl Pts',(66.677589495217,247.27066246832,24.5121455233208)) ;
#109205=CARTESIAN_POINT('Ctrl Pts',(66.6776689190512,247.269155710994,24.5113667312804)) ;
#109206=CARTESIAN_POINT('Ctrl Pts',(66.6791016407658,247.242022407589,24.4972902623795)) ;
#109207=CARTESIAN_POINT('Ctrl Pts',(66.6804764523606,247.216743161287,24.4833361073896)) ;
#109208=CARTESIAN_POINT('Ctrl Pts',(66.6838763528271,247.156118525715,24.4477999566119)) ;
#109209=CARTESIAN_POINT('Ctrl Pts',(66.6859237159345,247.121188973355,24.4255489497983)) ;
#109210=CARTESIAN_POINT('Ctrl Pts',(66.6905785877253,247.045196098053,24.3730887816372)) ;
#109211=CARTESIAN_POINT('Ctrl Pts',(66.6932043974035,247.004614632758,24.3422547967654)) ;
#109212=CARTESIAN_POINT('Ctrl Pts',(66.7005043372691,246.897316724161,24.2527417542348)) ;
#109213=CARTESIAN_POINT('Ctrl Pts',(66.7052453931358,246.833757851215,24.1905378350948)) ;
#109214=CARTESIAN_POINT('Ctrl Pts',(66.7121603957986,246.746503512077,24.090414949827)) ;
#109215=CARTESIAN_POINT('Ctrl Pts',(66.7144187371205,246.71890128238,24.0561055536296)) ;
#109216=CARTESIAN_POINT('Ctrl Pts',(66.7175997681525,246.680795494484,24.0047253430734)) ;
#109217=CARTESIAN_POINT('Ctrl Pts',(66.7185772458303,246.669198241514,23.9884908220179)) ;
#109218=CARTESIAN_POINT('Ctrl Pts',(66.7203334479191,246.648502004517,23.9583983321257)) ;
#109219=CARTESIAN_POINT('Ctrl Pts',(66.7211170566993,246.639314211992,23.9446059362019)) ;
#109220=CARTESIAN_POINT('Ctrl Pts',(66.723139446091,246.615774834301,23.9081088486848)) ;
#109221=CARTESIAN_POINT('Ctrl Pts',(66.7243591509514,246.601761119866,23.885191166995)) ;
#109222=CARTESIAN_POINT('Ctrl Pts',(66.727136033152,246.570548443607,23.8312793875019)) ;
#109223=CARTESIAN_POINT('Ctrl Pts',(66.728675983708,246.553769105835,23.8000568535244)) ;
#109224=CARTESIAN_POINT('Ctrl Pts',(66.7350389622131,246.487679759062,23.6671469696579)) ;
#109225=CARTESIAN_POINT('Ctrl Pts',(66.7396748067044,246.447718995985,23.5611454754844)) ;
#109226=CARTESIAN_POINT('Ctrl Pts',(66.746836208827,246.40525673722,23.4012450590947)) ;
#109227=CARTESIAN_POINT('Ctrl Pts',(66.7491533706109,246.394181727546,23.3499601749954)) ;
#109228=CARTESIAN_POINT('Ctrl Pts',(66.7529194256483,246.380530714064,23.2683891944497)) ;
#109229=CARTESIAN_POINT('Ctrl Pts',(66.754320259486,246.3763436531,23.2384068153772)) ;
#109230=CARTESIAN_POINT('Ctrl Pts',(66.7571290346595,246.369695429576,23.179133758156)) ;
#109231=CARTESIAN_POINT('Ctrl Pts',(66.7585350539675,246.36718836913,23.1498591431466)) ;
#109232=CARTESIAN_POINT('Ctrl Pts',(66.7622064319954,246.362724258965,23.0745016512219)) ;
#109233=CARTESIAN_POINT('Ctrl Pts',(66.7645038638689,246.361896476781,23.028378542832)) ;
#109234=CARTESIAN_POINT('Ctrl Pts',(66.7727046558224,246.365650040328,22.8671042789749)) ;
#109235=CARTESIAN_POINT('Ctrl Pts',(66.7788557938352,246.380187517667,22.7525145458225)) ;
#109236=CARTESIAN_POINT('Ctrl Pts',(66.7879140723522,246.419358406331,22.5845248105605)) ;
#109237=CARTESIAN_POINT('Ctrl Pts',(66.7908865423378,246.435222833392,22.5294168978723)) ;
#109238=CARTESIAN_POINT('Ctrl Pts',(66.7947732274432,246.460589101807,22.4557286402266)) ;
#109239=CARTESIAN_POINT('Ctrl Pts',(66.7957863875769,246.467660000436,22.4363558108457)) ;
#109240=CARTESIAN_POINT('Ctrl Pts',(66.797576050284,246.481031886641,22.4017161359753)) ;
#109241=CARTESIAN_POINT('Ctrl Pts',(66.798358657287,246.487203710612,22.3864046667242)) ;
#109242=CARTESIAN_POINT('Ctrl Pts',(66.8003312840557,246.503576010695,22.3474551513525)) ;
#109243=CARTESIAN_POINT('Ctrl Pts',(66.8015046235481,246.514096136701,22.3239566890586)) ;
#109244=CARTESIAN_POINT('Ctrl Pts',(66.8041443689531,246.539424984486,22.2707018828668)) ;
#109245=CARTESIAN_POINT('Ctrl Pts',(66.8055962555243,246.554585512081,22.2411245656152)) ;
#109246=CARTESIAN_POINT('Ctrl Pts',(66.8111134378521,246.616348325701,22.1289668447959)) ;
#109247=CARTESIAN_POINT('Ctrl Pts',(66.8150350209205,246.669039513265,22.0499424395502)) ;
#109248=CARTESIAN_POINT('Ctrl Pts',(66.8218681372491,246.768756808877,21.9247972156988)) ;
#109249=CARTESIAN_POINT('Ctrl Pts',(66.8247044336688,246.812324516317,21.8762188654033)) ;
#109250=CARTESIAN_POINT('Ctrl Pts',(66.8291253105473,246.881868058254,21.8072218688268)) ;
#109251=CARTESIAN_POINT('Ctrl Pts',(66.830629253651,246.9058002168,21.7848301163973)) ;
#109252=CARTESIAN_POINT('Ctrl Pts',(66.8335062751651,246.951936980499,21.7441304954835)) ;
#109253=CARTESIAN_POINT('Ctrl Pts',(66.8348723255865,246.97398682311,21.7256650951107)) ;
#109254=CARTESIAN_POINT('Ctrl Pts',(66.8381689391688,247.0274643318,21.6831709195566)) ;
#109255=CARTESIAN_POINT('Ctrl Pts',(66.840118057264,247.059287763348,21.6596697127395)) ;
#109256=CARTESIAN_POINT('Ctrl Pts',(66.8444830759063,247.130995574921,21.6105337130148)) ;
#109257=CARTESIAN_POINT('Ctrl Pts',(66.8469132559169,247.171195675123,21.5854206623276)) ;
#109258=CARTESIAN_POINT('Ctrl Pts',(66.8542990423983,247.294686396303,21.5153631363168)) ;
#109259=CARTESIAN_POINT('Ctrl Pts',(66.8593535462031,247.380767499731,21.4757276380051)) ;
#109260=CARTESIAN_POINT('Ctrl Pts',(66.8667041686732,247.513376272754,21.4277747664925)) ;
#109261=CARTESIAN_POINT('Ctrl Pts',(66.8690884760933,247.557663384699,21.4138081540797)) ;
#109262=CARTESIAN_POINT('Ctrl Pts',(66.8723880681245,247.621744251482,21.3964868788731)) ;
#109263=CARTESIAN_POINT('Ctrl Pts',(66.8733657184046,247.641105699513,21.3916224189345)) ;
#109264=CARTESIAN_POINT('Ctrl Pts',(66.8751381584295,247.677023634178,21.3832767778421)) ;
#109265=CARTESIAN_POINT('Ctrl Pts',(66.8759373524931,247.693553850535,21.3796984628091)) ;
#109266=CARTESIAN_POINT('Ctrl Pts',(66.8780298931353,247.73763191715,21.3708523168368)) ;
#109267=CARTESIAN_POINT('Ctrl Pts',(66.8793023530883,247.765263447124,21.3660240603119)) ;
#109268=CARTESIAN_POINT('Ctrl Pts',(66.8822311821563,247.830297485916,21.356333759192)) ;
#109269=CARTESIAN_POINT('Ctrl Pts',(66.8838681097253,247.86776892858,21.3520354644793)) ;
#109270=CARTESIAN_POINT('Ctrl Pts',(66.8914009094704,248.042892544921,21.3379077512273)) ;
#109271=CARTESIAN_POINT('Ctrl Pts',(66.8970665204552,248.18126848814,21.3438211107561)) ;
#109272=CARTESIAN_POINT('Ctrl Pts',(66.9048506159575,248.353018815771,21.3725822466916)) ;
#109273=CARTESIAN_POINT('Ctrl Pts',(66.9064955152177,248.388472650282,21.3797042202269)) ;
#109274=CARTESIAN_POINT('Ctrl Pts',(66.9095037958456,248.451533646708,21.3945067215273)) ;
#109275=CARTESIAN_POINT('Ctrl Pts',(66.9108538964968,248.47922678199,21.4017596296088)) ;
#109276=CARTESIAN_POINT('Ctrl Pts',(66.9139175008519,248.540628767216,21.4195315302631)) ;
#109277=CARTESIAN_POINT('Ctrl Pts',(66.9156416071258,248.574217745349,21.4304131944191)) ;
#109278=CARTESIAN_POINT('Ctrl Pts',(66.9218759832484,248.692238902346,21.4728067195242)) ;
#109279=CARTESIAN_POINT('Ctrl Pts',(66.9265555086629,248.774440746881,21.5100468643801)) ;
#109280=CARTESIAN_POINT('Ctrl Pts',(66.9342921276663,248.902815547265,21.5811596995484)) ;
#109281=CARTESIAN_POINT('Ctrl Pts',(66.9372988470437,248.950955657761,21.611108482509)) ;
#109282=CARTESIAN_POINT('Ctrl Pts',(66.9402651077865,248.99748421711,21.6434318722943)) ;
#109283=CARTESIAN_POINT('',(66.9402651077866,247.065925086493,21.6554848536836)) ;
#109284=CARTESIAN_POINT('Origin',(66.9402651077866,248.040265107786,23.0213203435596)) ;
#109285=CARTESIAN_POINT('Ctrl Pts',(66.9402651077869,247.065925086493,21.6554848536832)) ;
#109286=CARTESIAN_POINT('Ctrl Pts',(66.9396667652069,247.055655376798,21.662810911057)) ;
#109287=CARTESIAN_POINT('Ctrl Pts',(66.9390747274394,247.045468389277,21.6702527272938)) ;
#109288=CARTESIAN_POINT('Ctrl Pts',(66.9377500820969,247.022652288243,21.6873183636409)) ;
#109289=CARTESIAN_POINT('Ctrl Pts',(66.9370207683082,247.010073823175,21.6970080414531)) ;
#109290=CARTESIAN_POINT('Ctrl Pts',(66.9305114561942,246.897933188338,21.7859590655746)) ;
#109291=CARTESIAN_POINT('Ctrl Pts',(66.9251900559135,246.807547014657,21.8761346376893)) ;
#109292=CARTESIAN_POINT('Ctrl Pts',(66.9176770011432,246.700047100627,22.0110211304123)) ;
#109293=CARTESIAN_POINT('Ctrl Pts',(66.9156857672986,246.673312831565,22.0474979577537)) ;
#109294=CARTESIAN_POINT('Ctrl Pts',(66.9119145015543,246.626500509914,22.1171021179088)) ;
#109295=CARTESIAN_POINT('Ctrl Pts',(66.9101467604585,246.606033204961,22.1499309015644)) ;
#109296=CARTESIAN_POINT('Ctrl Pts',(66.9069079117755,246.571355558215,22.2100890547301)) ;
#109297=CARTESIAN_POINT('Ctrl Pts',(66.90545079394,246.556728440201,22.2371581847755)) ;
#109298=CARTESIAN_POINT('Ctrl Pts',(66.9021015713666,246.525349759796,22.2992519276511)) ;
#109299=CARTESIAN_POINT('Ctrl Pts',(66.9001962886567,246.509053389052,22.3344857903657)) ;
#109300=CARTESIAN_POINT('Ctrl Pts',(66.8924653337291,246.449074523345,22.4769339858134)) ;
#109301=CARTESIAN_POINT('Ctrl Pts',(66.8863507974608,246.415320799033,22.5879679183732)) ;
#109302=CARTESIAN_POINT('Ctrl Pts',(66.8755249468204,246.376533100155,22.7877630291077)) ;
#109303=CARTESIAN_POINT('Ctrl Pts',(66.8708568005199,246.366590976947,22.8751356895038)) ;
#109304=CARTESIAN_POINT('Ctrl Pts',(66.8652862956974,246.362736369824,22.9857465047002)) ;
#109305=CARTESIAN_POINT('Ctrl Pts',(66.8641530262041,246.362407267465,23.0086189873426)) ;
#109306=CARTESIAN_POINT('Ctrl Pts',(66.8622491506825,246.362645058344,23.0478403303629)) ;
#109307=CARTESIAN_POINT('Ctrl Pts',(66.8614679558607,246.362983098206,23.0641857098725)) ;
#109308=CARTESIAN_POINT('Ctrl Pts',(66.8596284129968,246.364363324888,23.1032741773016)) ;
#109309=CARTESIAN_POINT('Ctrl Pts',(66.8585808952561,246.365629514157,23.1260052564638)) ;
#109310=CARTESIAN_POINT('Ctrl Pts',(66.8533778600519,246.374362107618,23.2406884841878)) ;
#109311=CARTESIAN_POINT('Ctrl Pts',(66.8494973621617,246.388941443014,23.3319454566303)) ;
#109312=CARTESIAN_POINT('Ctrl Pts',(66.841621769976,246.433320860933,23.5126133967525)) ;
#109313=CARTESIAN_POINT('Ctrl Pts',(66.837636011074,246.463285368154,23.601641092563)) ;
#109314=CARTESIAN_POINT('Ctrl Pts',(66.8319022845595,246.514031654486,23.7188964443653)) ;
#109315=CARTESIAN_POINT('Ctrl Pts',(66.8303501366459,246.528480067574,23.7496793115379)) ;
#109316=CARTESIAN_POINT('Ctrl Pts',(66.8274768431064,246.556383029008,23.8047147592589)) ;
#109317=CARTESIAN_POINT('Ctrl Pts',(66.8261665734354,246.569522763633,23.829113438509)) ;
#109318=CARTESIAN_POINT('Ctrl Pts',(66.8231597257058,246.60055188431,23.8834613867776)) ;
#109319=CARTESIAN_POINT('Ctrl Pts',(66.8214515534895,246.618782828753,23.9131999631784)) ;
#109320=CARTESIAN_POINT('Ctrl Pts',(66.8134162094592,246.707213717487,24.0478431595334)) ;
#109321=CARTESIAN_POINT('Ctrl Pts',(66.8066933520668,246.788176496121,24.1451714051298)) ;
#109322=CARTESIAN_POINT('Ctrl Pts',(66.7959645933761,246.933483548018,24.2844592372969)) ;
#109323=CARTESIAN_POINT('Ctrl Pts',(66.7919836347308,246.991131322703,24.3327337132411)) ;
#109324=CARTESIAN_POINT('Ctrl Pts',(66.7870684111828,247.069871480798,24.3901447279616)) ;
#109325=CARTESIAN_POINT('Ctrl Pts',(66.7859595508096,247.088181865371,24.402943148782)) ;
#109326=CARTESIAN_POINT('Ctrl Pts',(66.7841052750378,247.119875740253,24.4241668345064)) ;
#109327=CARTESIAN_POINT('Ctrl Pts',(66.7833491088747,247.13313102736,24.4327744329739)) ;
#109328=CARTESIAN_POINT('Ctrl Pts',(66.7816144860752,247.164292992633,24.4523897261082)) ;
#109329=CARTESIAN_POINT('Ctrl Pts',(66.7806445405037,247.182288044758,24.4632503534813)) ;
#109330=CARTESIAN_POINT('Ctrl Pts',(66.7784542596184,247.224061045493,24.4874027943518)) ;
#109331=CARTESIAN_POINT('Ctrl Pts',(66.7772452853061,247.247964004995,24.5004570345183)) ;
#109332=CARTESIAN_POINT('Ctrl Pts',(66.7760547678839,247.272170398758,24.5129220264705)) ;
#109333=CARTESIAN_POINT('Origin',(67.8645744874958,248.040265107786,23.0213203435596)) ;
#109334=CARTESIAN_POINT('',(66.1803112149446,247.2721703913,24.51292202263)) ;
#109335=CARTESIAN_POINT('',(66.2786264835566,247.272170393047,24.5129220235297)) ;
#109336=CARTESIAN_POINT('',(67.8645744874958,247.272170391302,24.5129220226314)) ;
#109337=CARTESIAN_POINT('Ctrl Pts',(66.1803112149446,247.2721703913,24.51292202263)) ;
#109338=CARTESIAN_POINT('Ctrl Pts',(66.1813433707766,247.252559808362,24.5028236261527)) ;
#109339=CARTESIAN_POINT('Ctrl Pts',(66.1823542298636,247.233149391274,24.4923390118849)) ;
#109340=CARTESIAN_POINT('Ctrl Pts',(66.1875253071974,247.133303961512,24.4358355602508)) ;
#109341=CARTESIAN_POINT('Ctrl Pts',(66.1914076081278,247.056570630232,24.3835903719263)) ;
#109342=CARTESIAN_POINT('Ctrl Pts',(66.1995787953728,246.905796268944,24.261518189032)) ;
#109343=CARTESIAN_POINT('Ctrl Pts',(66.2038619131075,246.832992279066,24.1907650147767)) ;
#109344=CARTESIAN_POINT('Ctrl Pts',(66.2099411111492,246.744806082918,24.0879948669146)) ;
#109345=CARTESIAN_POINT('Ctrl Pts',(66.2114992468374,246.723388374238,24.0614376996361)) ;
#109346=CARTESIAN_POINT('Ctrl Pts',(66.2144126350155,246.685628776196,24.0115798954605)) ;
#109347=CARTESIAN_POINT('Ctrl Pts',(66.2157579827885,246.669041507144,23.9884807720735)) ;
#109348=CARTESIAN_POINT('Ctrl Pts',(66.218866033917,246.632676359447,23.935022181925)) ;
#109349=CARTESIAN_POINT('Ctrl Pts',(66.2206413827271,246.613279257904,23.9044218569684)) ;
#109350=CARTESIAN_POINT('Ctrl Pts',(66.2274407600937,246.544086080448,23.7870250333236)) ;
#109351=CARTESIAN_POINT('Ctrl Pts',(66.2326779323192,246.501100428625,23.6964675500411)) ;
#109352=CARTESIAN_POINT('Ctrl Pts',(66.2426141220224,246.435905778428,23.5199613514512)) ;
#109353=CARTESIAN_POINT('Ctrl Pts',(66.247282847654,246.411930371038,23.4350101637201)) ;
#109354=CARTESIAN_POINT('Ctrl Pts',(66.2528474822375,246.390306964967,23.3262786015287)) ;
#109355=CARTESIAN_POINT('Ctrl Pts',(66.2539707882866,246.386327819247,23.3039029805037)) ;
#109356=CARTESIAN_POINT('Ctrl Pts',(66.2558609765731,246.380277271449,23.2653512480786)) ;
#109357=CARTESIAN_POINT('Ctrl Pts',(66.2566381563459,246.377985074659,23.2492146791449)) ;
#109358=CARTESIAN_POINT('Ctrl Pts',(66.2584759021051,246.373043953528,23.2103733257162)) ;
#109359=CARTESIAN_POINT('Ctrl Pts',(66.2595253780448,246.370623215279,23.1876436573217)) ;
#109360=CARTESIAN_POINT('Ctrl Pts',(66.2659164827693,246.358506598636,23.0465495853369)) ;
#109361=CARTESIAN_POINT('Ctrl Pts',(66.2707929661402,246.360936047135,22.927473977817)) ;
#109362=CARTESIAN_POINT('Ctrl Pts',(66.2781260976021,246.382782027693,22.7557049790287)) ;
#109363=CARTESIAN_POINT('Ctrl Pts',(66.2804531518485,246.392260230318,22.7021319452076)) ;
#109364=CARTESIAN_POINT('Ctrl Pts',(66.2847382334814,246.413891640272,22.6070559651377)) ;
#109365=CARTESIAN_POINT('Ctrl Pts',(66.2866711898336,246.425078814962,22.5653833463018)) ;
#109366=CARTESIAN_POINT('Ctrl Pts',(66.2899874852909,246.446471308085,22.4964287018514)) ;
#109367=CARTESIAN_POINT('Ctrl Pts',(66.2913437830984,246.455803507772,22.4688972888353)) ;
#109368=CARTESIAN_POINT('Ctrl Pts',(66.29420161315,246.476617878492,22.412366840157)) ;
#109369=CARTESIAN_POINT('Ctrl Pts',(66.2957059918197,246.488202854992,22.3834178127161)) ;
#109370=CARTESIAN_POINT('Ctrl Pts',(66.300114035265,246.523898489675,22.3009588805755)) ;
#109371=CARTESIAN_POINT('Ctrl Pts',(66.3030796610631,246.55001708755,22.2483725592334)) ;
#109372=CARTESIAN_POINT('Ctrl Pts',(66.3123282536655,246.638004823593,22.0923295861903)) ;
#109373=CARTESIAN_POINT('Ctrl Pts',(66.3188137172501,246.708300127418,21.9940790822397)) ;
#109374=CARTESIAN_POINT('Ctrl Pts',(66.3264318419567,246.806541128242,21.8839972401355)) ;
#109375=CARTESIAN_POINT('Ctrl Pts',(66.3278142847729,246.825063353164,21.8642276482552)) ;
#109376=CARTESIAN_POINT('Ctrl Pts',(66.3302898413743,246.859689241534,21.8290189006079)) ;
#109377=CARTESIAN_POINT('Ctrl Pts',(66.3313906171093,246.875637679484,21.8134357692751)) ;
#109378=CARTESIAN_POINT('Ctrl Pts',(66.3332585807155,246.903780084173,21.7870137658914)) ;
#109379=CARTESIAN_POINT('Ctrl Pts',(66.3340352350746,246.915828982252,21.7760274591387)) ;
#109380=CARTESIAN_POINT('Ctrl Pts',(66.3358929538339,246.945491779348,21.7497622702217)) ;
#109381=CARTESIAN_POINT('Ctrl Pts',(66.3369620250232,246.963267069211,21.7346720269874)) ;
#109382=CARTESIAN_POINT('Ctrl Pts',(66.3421462388854,247.052503339811,21.6620609139343)) ;
#109383=CARTESIAN_POINT('Ctrl Pts',(66.3459917798339,247.128288778479,21.6100934858166)) ;
#109384=CARTESIAN_POINT('Ctrl Pts',(66.3540036519011,247.293450909869,21.515727092631)) ;
#109385=CARTESIAN_POINT('Ctrl Pts',(66.3581629994262,247.383086146486,21.4744988396476)) ;
#109386=CARTESIAN_POINT('Ctrl Pts',(66.3641487966006,247.509119373181,21.4294723281427)) ;
#109387=CARTESIAN_POINT('Ctrl Pts',(66.3657589138963,247.542791267655,21.418630267983)) ;
#109388=CARTESIAN_POINT('Ctrl Pts',(66.3687211974726,247.604069326491,21.4010164909781)) ;
#109389=CARTESIAN_POINT('Ctrl Pts',(66.3700611097827,247.631552937364,21.393866631955)) ;
#109390=CARTESIAN_POINT('Ctrl Pts',(66.3731197439098,247.693679024002,21.3793774898711)) ;
#109391=CARTESIAN_POINT('Ctrl Pts',(66.3748496628768,247.728398350681,21.3724306705407)) ;
#109392=CARTESIAN_POINT('Ctrl Pts',(66.3823405135124,247.876925771365,21.3475714137341)) ;
#109393=CARTESIAN_POINT('Ctrl Pts',(66.3884055174911,247.992186747832,21.3403093220466)) ;
#109394=CARTESIAN_POINT('Ctrl Pts',(66.3985316136585,248.18381146681,21.347968023991)) ;
#109395=CARTESIAN_POINT('Ctrl Pts',(66.4025633935918,248.260061519177,21.3562664659935)) ;
#109396=CARTESIAN_POINT('Ctrl Pts',(66.4075384096676,248.357679684639,21.3737155420066)) ;
#109397=CARTESIAN_POINT('Ctrl Pts',(66.4086526386034,248.379797239721,21.3781308796469)) ;
#109398=CARTESIAN_POINT('Ctrl Pts',(66.4105339272271,248.417739280072,21.3865041217997)) ;
#109399=CARTESIAN_POINT('Ctrl Pts',(66.4113109456865,248.43360583474,21.3902489357526)) ;
#109400=CARTESIAN_POINT('Ctrl Pts',(66.4131569463465,248.471764108648,21.3998442741033)) ;
#109401=CARTESIAN_POINT('Ctrl Pts',(66.4142144733173,248.493993974325,21.4059237248676)) ;
#109402=CARTESIAN_POINT('Ctrl Pts',(66.4195273178358,248.606950080852,21.43933096478)) ;
#109403=CARTESIAN_POINT('Ctrl Pts',(66.4234915730814,248.69537549886,21.4738529163656)) ;
#109404=CARTESIAN_POINT('Ctrl Pts',(66.4316893608181,248.870019415013,21.5597043765571)) ;
#109405=CARTESIAN_POINT('Ctrl Pts',(66.43591533074,248.955506052543,21.611658771381)) ;
#109406=CARTESIAN_POINT('Ctrl Pts',(66.4419265758015,249.063261427622,21.691101416567)) ;
#109407=CARTESIAN_POINT('Ctrl Pts',(66.4434818519492,249.090038813524,21.7121301917032)) ;
#109408=CARTESIAN_POINT('Ctrl Pts',(66.4463928703559,249.13798156533,21.7521975657878)) ;
#109409=CARTESIAN_POINT('Ctrl Pts',(66.44773884653,249.159337830941,21.7709883185167)) ;
#109410=CARTESIAN_POINT('Ctrl Pts',(66.4508526923697,249.206857025458,21.8149921273443)) ;
#109411=CARTESIAN_POINT('Ctrl Pts',(66.4526333823141,249.232698739022,21.8405298178118)) ;
#109412=CARTESIAN_POINT('Ctrl Pts',(66.4590334921456,249.320937170429,21.9335828241501)) ;
#109413=CARTESIAN_POINT('Ctrl Pts',(66.4638258052329,249.378590235261,22.0053593298391)) ;
#109414=CARTESIAN_POINT('Ctrl Pts',(66.4721979422453,249.467482101721,22.1368109230564)) ;
#109415=CARTESIAN_POINT('Ctrl Pts',(66.4757402991034,249.501557157053,22.1943190499528)) ;
#109416=CARTESIAN_POINT('Ctrl Pts',(66.4812548747535,249.550300941525,22.289051986342)) ;
#109417=CARTESIAN_POINT('Ctrl Pts',(66.483279816849,249.567227026516,22.3250353245085)) ;
#109418=CARTESIAN_POINT('Ctrl Pts',(66.4861640374801,249.590167909187,22.3786759759734)) ;
#109419=CARTESIAN_POINT('Ctrl Pts',(66.4870696114554,249.597191957824,22.3958850441892)) ;
#109420=CARTESIAN_POINT('Ctrl Pts',(66.4887838818375,249.610176935599,22.429273835447)) ;
#109421=CARTESIAN_POINT('Ctrl Pts',(66.4895943418289,249.616177078331,22.4454352076101)) ;
#109422=CARTESIAN_POINT('Ctrl Pts',(66.491835433538,249.632321015476,22.4910619162574)) ;
#109423=CARTESIAN_POINT('Ctrl Pts',(66.4932380895439,249.64189497613,22.5207227332288)) ;
#109424=CARTESIAN_POINT('Ctrl Pts',(66.4965706464777,249.663072976935,22.5931796846697)) ;
#109425=CARTESIAN_POINT('Ctrl Pts',(66.4984718910945,249.673817859092,22.6362028131126)) ;
#109426=CARTESIAN_POINT('Ctrl Pts',(66.5059738419224,249.709820300481,22.8092605717972)) ;
#109427=CARTESIAN_POINT('Ctrl Pts',(66.5114318524569,249.721346846575,22.9416488271284)) ;
#109428=CARTESIAN_POINT('Ctrl Pts',(66.5189266491568,249.716089524742,23.1089522508896)) ;
#109429=CARTESIAN_POINT('Ctrl Pts',(66.5205195603772,249.713900222963,23.1438443783018)) ;
#109430=CARTESIAN_POINT('Ctrl Pts',(66.5234646076773,249.707961017773,23.2069039348667)) ;
#109431=CARTESIAN_POINT('Ctrl Pts',(66.5248052370053,249.70458237105,23.2350932417736)) ;
#109432=CARTESIAN_POINT('Ctrl Pts',(66.5278851467738,249.695329222162,23.2986100873906)) ;
#109433=CARTESIAN_POINT('Ctrl Pts',(66.5296363786789,249.68903569244,23.3338617907631)) ;
#109434=CARTESIAN_POINT('Ctrl Pts',(66.5355841613892,249.664291945331,23.4507131688029)) ;
#109435=CARTESIAN_POINT('Ctrl Pts',(66.539919604221,249.640870750907,23.5311248654465)) ;
#109436=CARTESIAN_POINT('Ctrl Pts',(66.5500777890073,249.573219509862,23.7118672785298)) ;
#109437=CARTESIAN_POINT('Ctrl Pts',(66.5559297626788,249.524961690004,23.810295640799)) ;
#109438=CARTESIAN_POINT('Ctrl Pts',(66.5624651069322,249.456263635375,23.9214577718262)) ;
#109439=CARTESIAN_POINT('Ctrl Pts',(66.5635151307348,249.444715394716,23.9393719142512)) ;
#109440=CARTESIAN_POINT('Ctrl Pts',(66.5653344144998,249.423717332963,23.9706210697346)) ;
#109441=CARTESIAN_POINT('Ctrl Pts',(66.5661112394953,249.414409217415,23.9840455991035)) ;
#109442=CARTESIAN_POINT('Ctrl Pts',(66.5680012349603,249.390925402805,24.0168801582264)) ;
#109443=CARTESIAN_POINT('Ctrl Pts',(66.5691010007004,249.376526352373,24.0361250349577)) ;
#109444=CARTESIAN_POINT('Ctrl Pts',(66.5715363590945,249.3431517713,24.0787887461828)) ;
#109445=CARTESIAN_POINT('Ctrl Pts',(66.5728605366494,249.323948567457,24.1020191862595)) ;
#109446=CARTESIAN_POINT('Ctrl Pts',(66.5774386753978,249.254434287927,24.1816427137725)) ;
#109447=CARTESIAN_POINT('Ctrl Pts',(66.5805906138049,249.200948957556,24.2351442704249)) ;
#109448=CARTESIAN_POINT('Ctrl Pts',(66.5871961043524,249.08309164241,24.3380992979809)) ;
#109449=CARTESIAN_POINT('Ctrl Pts',(66.5906485378677,249.018376199185,24.3868574369339)) ;
#109450=CARTESIAN_POINT('Ctrl Pts',(66.5958732170954,248.920036147092,24.4503599800255)) ;
#109451=CARTESIAN_POINT('Ctrl Pts',(66.5975155661291,248.889049297604,24.468979335324)) ;
#109452=CARTESIAN_POINT('Ctrl Pts',(66.6005105289135,248.83266991517,24.5004238283064)) ;
#109453=CARTESIAN_POINT('Ctrl Pts',(66.6018494713179,248.807506669269,24.5136315614698)) ;
#109454=CARTESIAN_POINT('Ctrl Pts',(66.6048715551597,248.750891062974,24.5415375405759)) ;
#109455=CARTESIAN_POINT('Ctrl Pts',(66.6065645988116,248.719294019325,24.555911202305)) ;
#109456=CARTESIAN_POINT('Ctrl Pts',(66.6102195017308,248.651369151631,24.5843019148011)) ;
#109457=CARTESIAN_POINT('Ctrl Pts',(66.6121880085618,248.614953475018,24.5980551222346)) ;
#109458=CARTESIAN_POINT('Ctrl Pts',(66.6182653362812,248.502830294328,24.636000476212)) ;
#109459=CARTESIAN_POINT('Ctrl Pts',(66.622464789576,248.425855514463,24.656091673371)) ;
#109460=CARTESIAN_POINT('Ctrl Pts',(66.6304919812157,248.276375435229,24.6839594030375)) ;
#109461=CARTESIAN_POINT('Ctrl Pts',(66.6343105948735,248.204206445034,24.6926195689881)) ;
#109462=CARTESIAN_POINT('Ctrl Pts',(66.6391644383837,248.107935743506,24.6978740064464)) ;
#109463=CARTESIAN_POINT('Ctrl Pts',(66.6403442568994,248.084145184136,24.6986653106294)) ;
#109464=CARTESIAN_POINT('Ctrl Pts',(66.6422929520108,248.044004342234,24.6991457608791)) ;
#109465=CARTESIAN_POINT('Ctrl Pts',(66.6430741543972,248.027662126044,24.6991026082971)) ;
#109466=CARTESIAN_POINT('Ctrl Pts',(66.6448756920634,247.989371233389,24.6984419333739)) ;
#109467=CARTESIAN_POINT('Ctrl Pts',(66.6458867725033,247.967429763483,24.6976323981297)) ;
#109468=CARTESIAN_POINT('Ctrl Pts',(66.6480805523382,247.919058359992,24.6948961249696)) ;
#109469=CARTESIAN_POINT('Ctrl Pts',(66.6492552200846,247.892645265416,24.6927734398668)) ;
#109470=CARTESIAN_POINT('Ctrl Pts',(66.6554023650222,247.752723802649,24.6781857982299)) ;
#109471=CARTESIAN_POINT('Ctrl Pts',(66.6600807567697,247.640656613757,24.6547825211783)) ;
#109472=CARTESIAN_POINT('Ctrl Pts',(66.6676940274392,247.471135374613,24.6008750044367)) ;
#109473=CARTESIAN_POINT('Ctrl Pts',(66.670474229424,247.411591411855,24.5781344447023)) ;
#109474=CARTESIAN_POINT('Ctrl Pts',(66.6747189934773,247.326034152191,24.539748667258)) ;
#109475=CARTESIAN_POINT('Ctrl Pts',(66.6761026158922,247.298918886678,24.5266960604741)) ;
#109476=CARTESIAN_POINT('Ctrl Pts',(66.6775101468938,247.272170391243,24.5129220226009)) ;
#109477=CARTESIAN_POINT('Ctrl Pts',(66.7760547678839,247.272170398758,24.5129220264705)) ;
#109478=CARTESIAN_POINT('Ctrl Pts',(66.7746260058025,247.30122094173,24.5278814949449)) ;
#109479=CARTESIAN_POINT('Ctrl Pts',(66.7732237782137,247.330708514315,24.5419922776791)) ;
#109480=CARTESIAN_POINT('Ctrl Pts',(66.7670524975973,247.463406236797,24.6007899101927)) ;
#109481=CARTESIAN_POINT('Ctrl Pts',(66.7624140234548,247.57053297492,24.6358921340749)) ;
#109482=CARTESIAN_POINT('Ctrl Pts',(66.7554925396234,247.72504518138,24.6698269201577)) ;
#109483=CARTESIAN_POINT('Ctrl Pts',(66.7534508186818,247.770104091084,24.67780764622)) ;
#109484=CARTESIAN_POINT('Ctrl Pts',(66.7500001725226,247.844744109367,24.6879011472955)) ;
#109485=CARTESIAN_POINT('Ctrl Pts',(66.7486233362743,247.874155812901,24.6910890746417)) ;
#109486=CARTESIAN_POINT('Ctrl Pts',(66.7457616483045,247.934415189029,24.6960127256743)) ;
#109487=CARTESIAN_POINT('Ctrl Pts',(66.7442752550599,247.965257197395,24.6976772410028)) ;
#109488=CARTESIAN_POINT('Ctrl Pts',(66.7400501988935,248.051591037136,24.6999493183941)) ;
#109489=CARTESIAN_POINT('Ctrl Pts',(66.7372587974006,248.107089863153,24.6986566814682)) ;
#109490=CARTESIAN_POINT('Ctrl Pts',(66.7281543674001,248.283881268916,24.6857505253967)) ;
#109491=CARTESIAN_POINT('Ctrl Pts',(66.7216190595541,248.40400683852,24.663686267586)) ;
#109492=CARTESIAN_POINT('Ctrl Pts',(66.7139415018536,248.546759586007,24.6210231980383)) ;
#109493=CARTESIAN_POINT('Ctrl Pts',(66.7125546810463,248.572645306484,24.6125957164748)) ;
#109494=CARTESIAN_POINT('Ctrl Pts',(66.7100703821569,248.619448747485,24.5960881203137)) ;
#109495=CARTESIAN_POINT('Ctrl Pts',(66.7089653361317,248.640431553691,24.5882113930192)) ;
#109496=CARTESIAN_POINT('Ctrl Pts',(66.7070853766348,248.676562264737,24.5738159593817)) ;
#109497=CARTESIAN_POINT('Ctrl Pts',(66.7063011777376,248.691781978999,24.5674906154246)) ;
#109498=CARTESIAN_POINT('Ctrl Pts',(66.7044104191885,248.72882797282,24.5514500199998)) ;
#109499=CARTESIAN_POINT('Ctrl Pts',(66.7033166386824,248.75054399774,24.541491268422)) ;
#109500=CARTESIAN_POINT('Ctrl Pts',(66.6991362639863,248.834155148673,24.5009649874613)) ;
#109501=CARTESIAN_POINT('Ctrl Pts',(66.6961915715714,248.894356498031,24.4670515714953)) ;
#109502=CARTESIAN_POINT('Ctrl Pts',(66.6898114863581,249.021057481715,24.3849925749504)) ;
#109503=CARTESIAN_POINT('Ctrl Pts',(66.6863924717727,249.08646071182,24.3354855302863)) ;
#109504=CARTESIAN_POINT('Ctrl Pts',(66.6811458698143,249.177639297353,24.2553317003306)) ;
#109505=CARTESIAN_POINT('Ctrl Pts',(66.6794141458992,249.206363539487,24.2282247780209)) ;
#109506=CARTESIAN_POINT('Ctrl Pts',(66.6760747774206,249.258751821425,24.175168608329)) ;
#109507=CARTESIAN_POINT('Ctrl Pts',(66.6744757298295,249.282609669363,24.1494406778354)) ;
#109508=CARTESIAN_POINT('Ctrl Pts',(66.6715180740521,249.324368770513,24.1014759530029)) ;
#109509=CARTESIAN_POINT('Ctrl Pts',(66.6701709728188,249.342542641005,24.0794939918291)) ;
#109510=CARTESIAN_POINT('Ctrl Pts',(66.6670727237618,249.382395269289,24.0287083108948)) ;
#109511=CARTESIAN_POINT('Ctrl Pts',(66.6653094409075,249.40372325872,23.9996482675196)) ;
#109512=CARTESIAN_POINT('Ctrl Pts',(66.658078213854,249.485809388289,23.8799003123941)) ;
#109513=CARTESIAN_POINT('Ctrl Pts',(66.6523467487962,249.53858264882,23.7840769448208)) ;
#109514=CARTESIAN_POINT('Ctrl Pts',(66.6422501659289,249.614112463005,23.6083454299327)) ;
#109515=CARTESIAN_POINT('Ctrl Pts',(66.6379183902125,249.640966593167,23.5305847452125)) ;
#109516=CARTESIAN_POINT('Ctrl Pts',(66.6327016987057,249.667660571226,23.4298718929731)) ;
#109517=CARTESIAN_POINT('Ctrl Pts',(66.6316152393811,249.672884913724,23.4084676204684)) ;
#109518=CARTESIAN_POINT('Ctrl Pts',(66.6297608359402,249.681244338317,23.3710327246674)) ;
#109519=CARTESIAN_POINT('Ctrl Pts',(66.6289839721954,249.684569379557,23.355049392568)) ;
#109520=CARTESIAN_POINT('Ctrl Pts',(66.6271101753576,249.692144048794,23.3157715865528)) ;
#109521=CARTESIAN_POINT('Ctrl Pts',(66.6260259476179,249.696134776591,23.2924315848488)) ;
#109522=CARTESIAN_POINT('Ctrl Pts',(66.6214111606782,249.711276519546,23.190993044962)) ;
#109523=CARTESIAN_POINT('Ctrl Pts',(66.6180740139388,249.717406403861,23.1122421198656)) ;
#109524=CARTESIAN_POINT('Ctrl Pts',(66.6115603529938,249.718514756525,22.9576382593858)) ;
#109525=CARTESIAN_POINT('Ctrl Pts',(66.6083892208669,249.71393207545,22.8819797664537)) ;
#109526=CARTESIAN_POINT('Ctrl Pts',(66.6034630176377,249.699392269194,22.7691492301083)) ;
#109527=CARTESIAN_POINT('Ctrl Pts',(66.6017904699721,249.693246119073,22.7315846184465)) ;
#109528=CARTESIAN_POINT('Ctrl Pts',(66.5985513916876,249.679171002658,22.6607668524994)) ;
#109529=CARTESIAN_POINT('Ctrl Pts',(66.5969923996442,249.671492795986,22.6274835724027)) ;
#109530=CARTESIAN_POINT('Ctrl Pts',(66.5940856369422,249.655608301905,22.5671051469266)) ;
#109531=CARTESIAN_POINT('Ctrl Pts',(66.5927480954021,249.647721712694,22.5399387580991)) ;
#109532=CARTESIAN_POINT('Ctrl Pts',(66.5896718865396,249.628322388765,22.4789212221474)) ;
#109533=CARTESIAN_POINT('Ctrl Pts',(66.5879211814873,249.616406993283,22.4452133534045)) ;
#109534=CARTESIAN_POINT('Ctrl Pts',(66.5807965439382,249.564502251018,22.3120751267256)) ;
#109535=CARTESIAN_POINT('Ctrl Pts',(66.5751680679827,249.516108225971,22.2162053244757)) ;
#109536=CARTESIAN_POINT('Ctrl Pts',(66.5650278432338,249.413677381476,22.0539720887832)) ;
#109537=CARTESIAN_POINT('Ctrl Pts',(66.5605501432138,249.363078582201,21.9858542324839)) ;
#109538=CARTESIAN_POINT('Ctrl Pts',(66.5552205830076,249.29331441755,21.9054421131403)) ;
#109539=CARTESIAN_POINT('Ctrl Pts',(66.554149583085,249.278763246229,21.8893136128457)) ;
#109540=CARTESIAN_POINT('Ctrl Pts',(66.5523123682857,249.252761508665,21.861595069506)) ;
#109541=CARTESIAN_POINT('Ctrl Pts',(66.5515377065103,249.241449043364,21.8498821635411)) ;
#109542=CARTESIAN_POINT('Ctrl Pts',(66.5496598646258,249.213180120709,21.8214527612052)) ;
#109543=CARTESIAN_POINT('Ctrl Pts',(66.5485697281867,249.196035492092,21.8049294698952)) ;
#109544=CARTESIAN_POINT('Ctrl Pts',(66.5443833462662,249.127675848237,21.7417979802871)) ;
#109545=CARTESIAN_POINT('Ctrl Pts',(66.5414308997888,249.073944433215,21.6980109000327)) ;
#109546=CARTESIAN_POINT('Ctrl Pts',(66.5350558600926,248.951295785619,21.6101029699729)) ;
#109547=CARTESIAN_POINT('Ctrl Pts',(66.5316491198968,248.881550375901,21.5674461356559)) ;
#109548=CARTESIAN_POINT('Ctrl Pts',(66.5257699369946,248.760598629428,21.5050989736082)) ;
#109549=CARTESIAN_POINT('Ctrl Pts',(66.5233696573372,248.711036569657,21.482530982679)) ;
#109550=CARTESIAN_POINT('Ctrl Pts',(66.5195002956231,248.632002613909,21.451087786692)) ;
#109551=CARTESIAN_POINT('Ctrl Pts',(66.518083865029,248.603234035771,21.4405454038247)) ;
#109552=CARTESIAN_POINT('Ctrl Pts',(66.515260050051,248.546341212787,21.4214468374385)) ;
#109553=CARTESIAN_POINT('Ctrl Pts',(66.5138551748204,248.51824881191,21.4128304580471)) ;
#109554=CARTESIAN_POINT('Ctrl Pts',(66.5102218867648,248.44620808186,21.3927883669801)) ;
#109555=CARTESIAN_POINT('Ctrl Pts',(66.5079632221664,248.401997377095,21.3824013663251)) ;
#109556=CARTESIAN_POINT('Ctrl Pts',(66.5000030746146,248.247989208181,21.3527535525927)) ;
#109557=CARTESIAN_POINT('Ctrl Pts',(66.4940715821999,248.136735613736,21.3426440522411)) ;
#109558=CARTESIAN_POINT('Ctrl Pts',(66.4850479824135,247.965100932978,21.3441735386682)) ;
#109559=CARTESIAN_POINT('Ctrl Pts',(66.4819158122742,247.904955690021,21.3479514935566)) ;
#109560=CARTESIAN_POINT('Ctrl Pts',(66.4778460981594,247.824085839844,21.3574210153989)) ;
#109561=CARTESIAN_POINT('Ctrl Pts',(66.4768021572404,247.803078659241,21.3602853912995)) ;
#109562=CARTESIAN_POINT('Ctrl Pts',(66.4749879001035,247.765964581455,21.3660644842077)) ;
#109563=CARTESIAN_POINT('Ctrl Pts',(66.4742102736576,247.749837354732,21.3688178530435)) ;
#109564=CARTESIAN_POINT('Ctrl Pts',(66.4723095312937,247.709904599137,21.3762381893585)) ;
#109565=CARTESIAN_POINT('Ctrl Pts',(66.4712002280521,247.686155827551,21.3811861789226)) ;
#109566=CARTESIAN_POINT('Ctrl Pts',(66.4687383944685,247.632770014284,21.3935226772839)) ;
#109567=CARTESIAN_POINT('Ctrl Pts',(66.4673976724533,247.603210410797,21.4012089825697)) ;
#109568=CARTESIAN_POINT('Ctrl Pts',(66.4627079699437,247.499121090916,21.4313314980471)) ;
#109569=CARTESIAN_POINT('Ctrl Pts',(66.4594658248662,247.425959780457,21.4581405427182)) ;
#109570=CARTESIAN_POINT('Ctrl Pts',(66.4528733965416,247.28353497792,21.5218799962939)) ;
#109571=CARTESIAN_POINT('Ctrl Pts',(66.4495295860475,247.214472648948,21.5587788630213)) ;
#109572=CARTESIAN_POINT('Ctrl Pts',(66.4444322179629,247.117795631709,21.6194690087539)) ;
#109573=CARTESIAN_POINT('Ctrl Pts',(66.4427980899802,247.087975658428,21.6395527437328)) ;
#109574=CARTESIAN_POINT('Ctrl Pts',(66.4398120180902,247.035791991214,21.6771904005733)) ;
#109575=CARTESIAN_POINT('Ctrl Pts',(66.43847339613,247.0131856024,21.6943843531252)) ;
#109576=CARTESIAN_POINT('Ctrl Pts',(66.4354443339418,246.963835150169,21.733936192661)) ;
#109577=CARTESIAN_POINT('Ctrl Pts',(66.4337437102941,246.937329989998,21.7565700436083)) ;
#109578=CARTESIAN_POINT('Ctrl Pts',(66.4273404585247,246.841945861539,21.8433023262077)) ;
#109579=CARTESIAN_POINT('Ctrl Pts',(66.4224481469518,246.777795351718,21.9123287626435)) ;
#109580=CARTESIAN_POINT('Ctrl Pts',(66.4122562516643,246.658570100657,22.0644466034939)) ;
#109581=CARTESIAN_POINT('Ctrl Pts',(66.4069702007148,246.604412402534,22.1478118410557)) ;
#109582=CARTESIAN_POINT('Ctrl Pts',(66.4008579163586,246.547354882143,22.2554387607092)) ;
#109583=CARTESIAN_POINT('Ctrl Pts',(66.3997413969471,246.537176004263,22.2756134471926)) ;
#109584=CARTESIAN_POINT('Ctrl Pts',(66.3978583437663,246.520364381107,22.3106782134209)) ;
#109585=CARTESIAN_POINT('Ctrl Pts',(66.3970817493275,246.513536043084,22.3254691703481)) ;
#109586=CARTESIAN_POINT('Ctrl Pts',(66.3952399503525,246.49760490167,22.361341806325)) ;
#109587=CARTESIAN_POINT('Ctrl Pts',(66.3941860552735,246.488717625122,22.3825146784016)) ;
#109588=CARTESIAN_POINT('Ctrl Pts',(66.3918760824001,246.469873282128,22.4301247473335)) ;
#109589=CARTESIAN_POINT('Ctrl Pts',(66.3906296235424,246.460143549805,22.4566445995034)) ;
#109590=CARTESIAN_POINT('Ctrl Pts',(66.3865342775035,246.429954626768,22.5458314235494)) ;
#109591=CARTESIAN_POINT('Ctrl Pts',(66.3837671257855,246.41251838099,22.6094578036103)) ;
#109592=CARTESIAN_POINT('Ctrl Pts',(66.3770678641161,246.379587455675,22.7650616052376)) ;
#109593=CARTESIAN_POINT('Ctrl Pts',(66.3731309786512,246.367925485131,22.85762042588)) ;
#109594=CARTESIAN_POINT('Ctrl Pts',(66.3673624905043,246.362473781355,22.9869567235963)) ;
#109595=CARTESIAN_POINT('Ctrl Pts',(66.365714524909,246.36212312572,23.0232883115724)) ;
#109596=CARTESIAN_POINT('Ctrl Pts',(66.3627155375746,246.36360030673,23.088012219576)) ;
#109597=CARTESIAN_POINT('Ctrl Pts',(66.3613785083754,246.364970439127,23.1164009524269)) ;
#109598=CARTESIAN_POINT('Ctrl Pts',(66.3583956892156,246.369560152878,23.1786237154051)) ;
#109599=CARTESIAN_POINT('Ctrl Pts',(66.356741295661,246.373088024749,23.2124218230698)) ;
#109600=CARTESIAN_POINT('Ctrl Pts',(66.3502387329908,246.390670619754,23.342481683184)) ;
#109601=CARTESIAN_POINT('Ctrl Pts',(66.345181320729,246.412058631375,23.4375493679102)) ;
#109602=CARTESIAN_POINT('Ctrl Pts',(66.3348658700508,246.471383231633,23.6239178409833)) ;
#109603=CARTESIAN_POINT('Ctrl Pts',(66.3296285504755,246.50938998515,23.7148166169628)) ;
#109604=CARTESIAN_POINT('Ctrl Pts',(66.3235545872295,246.565691239186,23.821939633711)) ;
#109605=CARTESIAN_POINT('Ctrl Pts',(66.3224336160856,246.576648060666,23.8417986001987)) ;
#109606=CARTESIAN_POINT('Ctrl Pts',(66.3205462347099,246.596160543956,23.8755289644073)) ;
#109607=CARTESIAN_POINT('Ctrl Pts',(66.3197695962981,246.604521011534,23.889507700196)) ;
#109608=CARTESIAN_POINT('Ctrl Pts',(66.3179319715617,246.62510505987,23.9228134787423)) ;
#109609=CARTESIAN_POINT('Ctrl Pts',(66.3168821103347,246.637522289801,23.9420160084296)) ;
#109610=CARTESIAN_POINT('Ctrl Pts',(66.312503861122,246.691857407885,24.0223898010052)) ;
#109611=CARTESIAN_POINT('Ctrl Pts',(66.3093487905346,246.737416069323,24.0810039240524)) ;
#109612=CARTESIAN_POINT('Ctrl Pts',(66.3012494422756,246.86493954656,24.2243623970562)) ;
#109613=CARTESIAN_POINT('Ctrl Pts',(66.2963437600446,246.952205316677,24.3038275948203)) ;
#109614=CARTESIAN_POINT('Ctrl Pts',(66.2895040320248,247.075373183139,24.3942959719754)) ;
#109615=CARTESIAN_POINT('Ctrl Pts',(66.2879041695097,247.104323067194,24.414191768733)) ;
#109616=CARTESIAN_POINT('Ctrl Pts',(66.2849523246596,247.157763036749,24.4484997266618)) ;
#109617=CARTESIAN_POINT('Ctrl Pts',(66.2836121503365,247.182035619835,24.4632263496245)) ;
#109618=CARTESIAN_POINT('Ctrl Pts',(66.2810583911226,247.228238561312,24.4896785004803)) ;
#109619=CARTESIAN_POINT('Ctrl Pts',(66.2798502066838,247.250077654912,24.5015454505323)) ;
#109620=CARTESIAN_POINT('Ctrl Pts',(66.2786264835566,247.272170393047,24.5129220235297)) ;
#109621=CARTESIAN_POINT('Origin',(67.8645744874958,248.040265107786,23.0213203435596)) ;
#109622=CARTESIAN_POINT('',(65.6787784786721,247.273150902455,24.5110052762898)) ;
#109623=CARTESIAN_POINT('',(65.7773991381782,247.271019322241,24.5151747855319)) ;
#109624=CARTESIAN_POINT('',(67.8645744874958,247.272170391302,24.5129220226314)) ;
#109625=CARTESIAN_POINT('',(66.0159551384008,249.720171106522,23.0220506151371)) ;
#109626=CARTESIAN_POINT('Ctrl Pts',(66.0159551384008,249.720171106522,23.0220506151371)) ;
#109627=CARTESIAN_POINT('Ctrl Pts',(65.9924478890589,249.717352510068,22.5280345358421)) ;
#109628=CARTESIAN_POINT('Ctrl Pts',(65.9431670940094,249.230820605579,21.4875383102286)) ;
#109629=CARTESIAN_POINT('Ctrl Pts',(65.8681127532527,247.483588425899,21.135600117915)) ;
#109630=CARTESIAN_POINT('Ctrl Pts',(65.7907921161305,246.169079052195,22.4175852103976)) ;
#109631=CARTESIAN_POINT('Ctrl Pts',(65.7276806912704,246.428124491481,23.8937448247901)) ;
#109632=CARTESIAN_POINT('Ctrl Pts',(65.6903428121175,247.05537004442,24.3995509628447)) ;
#109633=CARTESIAN_POINT('Ctrl Pts',(65.6787784786721,247.273150902455,24.5110052762898)) ;
#109634=CARTESIAN_POINT('Ctrl Pts',(66.017195723299,249.718014971169,23.0219974094422)) ;
#109635=CARTESIAN_POINT('Ctrl Pts',(66.0183307318067,249.718006022754,23.0441713249733)) ;
#109636=CARTESIAN_POINT('Ctrl Pts',(66.0194529908537,249.717557483142,23.0663438085581)) ;
#109637=CARTESIAN_POINT('Ctrl Pts',(66.021465334691,249.715940060581,23.1067040054386)) ;
#109638=CARTESIAN_POINT('Ctrl Pts',(66.0223609644086,249.714914173444,23.1248938511936)) ;
#109639=CARTESIAN_POINT('Ctrl Pts',(66.0239984203668,249.712457011443,23.1586667450493)) ;
#109640=CARTESIAN_POINT('Ctrl Pts',(66.0247434850627,249.711103734731,23.1742520498825)) ;
#109641=CARTESIAN_POINT('Ctrl Pts',(66.0265597681603,249.70721549077,23.2127720293691)) ;
#109642=CARTESIAN_POINT('Ctrl Pts',(66.0276184783189,249.704425149736,23.2356769875758)) ;
#109643=CARTESIAN_POINT('Ctrl Pts',(66.0328458013089,249.688038012043,23.3504224814466)) ;
#109644=CARTESIAN_POINT('Ctrl Pts',(66.0367357202072,249.667306265743,23.4410863473143)) ;
#109645=CARTESIAN_POINT('Ctrl Pts',(66.0449183114521,249.608454766642,23.626226805628)) ;
#109646=CARTESIAN_POINT('Ctrl Pts',(66.0492050618568,249.569032217515,23.7198903405972)) ;
#109647=CARTESIAN_POINT('Ctrl Pts',(66.0552895113974,249.505360238047,23.8395543279455)) ;
#109648=CARTESIAN_POINT('Ctrl Pts',(66.0568488359026,249.488408110045,23.8691954879158)) ;
#109649=CARTESIAN_POINT('Ctrl Pts',(66.0597632646483,249.45570255263,23.9225363415388)) ;
#109650=CARTESIAN_POINT('Ctrl Pts',(66.0611084086615,249.440227748398,23.9463921930167)) ;
#109651=CARTESIAN_POINT('Ctrl Pts',(66.0642142910449,249.403697978,23.9996889655832)) ;
#109652=CARTESIAN_POINT('Ctrl Pts',(66.0659876070543,249.382281997893,24.0288642802643)) ;
#109653=CARTESIAN_POINT('Ctrl Pts',(66.0721834043994,249.305597893543,24.1265455949657)) ;
#109654=CARTESIAN_POINT('Ctrl Pts',(66.0767615615587,249.245898013545,24.1913787261678)) ;
#109655=CARTESIAN_POINT('Ctrl Pts',(66.0850758752835,249.130282496361,24.2986490598222)) ;
#109656=CARTESIAN_POINT('Ctrl Pts',(66.0887786124962,249.076262594256,24.3428407015681)) ;
#109657=CARTESIAN_POINT('Ctrl Pts',(66.0938953160846,248.996084900296,24.4004852683806)) ;
#109658=CARTESIAN_POINT('Ctrl Pts',(66.0953822343774,248.972083987731,24.4168134712521)) ;
#109659=CARTESIAN_POINT('Ctrl Pts',(66.0980191405281,248.927983240968,24.4451705569346)) ;
#109660=CARTESIAN_POINT('Ctrl Pts',(66.0991783383882,248.908032119533,24.4574169362175)) ;
#109661=CARTESIAN_POINT('Ctrl Pts',(66.1011048873075,248.873756109275,24.4774809717395)) ;
#109662=CARTESIAN_POINT('Ctrl Pts',(66.1018838491254,248.859562755676,24.4855137853536)) ;
#109663=CARTESIAN_POINT('Ctrl Pts',(66.1036754997755,248.826121581469,24.5038014164912)) ;
#109664=CARTESIAN_POINT('Ctrl Pts',(66.1046791770869,248.806787291003,24.5138900564829)) ;
#109665=CARTESIAN_POINT('Ctrl Pts',(66.1110360019845,248.681024783047,24.5764244379773)) ;
#109666=CARTESIAN_POINT('Ctrl Pts',(66.1159123410292,248.569475347406,24.6178363717818)) ;
#109667=CARTESIAN_POINT('Ctrl Pts',(66.1232769014826,248.400841243134,24.6608001380958)) ;
#109668=CARTESIAN_POINT('Ctrl Pts',(66.125642992403,248.346558997878,24.6718029448756)) ;
#109669=CARTESIAN_POINT('Ctrl Pts',(66.1299885237556,248.248709121012,24.6866427419714)) ;
#109670=CARTESIAN_POINT('Ctrl Pts',(66.1319415846934,248.205347785647,24.6914984695287)) ;
#109671=CARTESIAN_POINT('Ctrl Pts',(66.1352812621692,248.132794340044,24.696770130613)) ;
#109672=CARTESIAN_POINT('Ctrl Pts',(66.1366398584891,248.103691522083,24.6981240347842)) ;
#109673=CARTESIAN_POINT('Ctrl Pts',(66.1394930739171,248.043532547513,24.6993543303389)) ;
#109674=CARTESIAN_POINT('Ctrl Pts',(66.140990222113,248.012485630232,24.6991275100511)) ;
#109675=CARTESIAN_POINT('Ctrl Pts',(66.1453372502987,247.923879381478,24.6960201650657)) ;
#109676=CARTESIAN_POINT('Ctrl Pts',(66.1482462447078,247.866441389921,24.6910357596945)) ;
#109677=CARTESIAN_POINT('Ctrl Pts',(66.1574990457002,247.688730677397,24.6663447055157)) ;
#109678=CARTESIAN_POINT('Ctrl Pts',(66.1640580625483,247.570277716357,24.636495508201)) ;
#109679=CARTESIAN_POINT('Ctrl Pts',(66.1717533023906,247.430598429913,24.5846155480122)) ;
#109680=CARTESIAN_POINT('Ctrl Pts',(66.1731423478088,247.405325839823,24.5745227103385)) ;
#109681=CARTESIAN_POINT('Ctrl Pts',(66.1756281601356,247.35974615837,24.5550215057614)) ;
#109682=CARTESIAN_POINT('Ctrl Pts',(66.1767326836644,247.339360362305,24.5458130193764)) ;
#109683=CARTESIAN_POINT('Ctrl Pts',(66.1786043328474,247.304442562548,24.5291917141201)) ;
#109684=CARTESIAN_POINT('Ctrl Pts',(66.1793810626801,247.289824813099,24.5219702977892)) ;
#109685=CARTESIAN_POINT('Ctrl Pts',(66.1802009438783,247.274264917999,24.5139991966942)) ;
#109686=CARTESIAN_POINT('Ctrl Pts',(66.1802561097733,247.273217369381,24.5134611600847)) ;
#109687=CARTESIAN_POINT('Ctrl Pts',(66.1803112149446,247.2721703913,24.51292202263)) ;
#109688=CARTESIAN_POINT('',(66.1145741302299,249.716961070455,23.0201358258391)) ;
#109689=CARTESIAN_POINT('Ctrl Pts',(66.2786264835566,247.272170393047,24.5129220235297)) ;
#109690=CARTESIAN_POINT('Ctrl Pts',(66.2780959412381,247.281748648333,24.5178543103196)) ;
#109691=CARTESIAN_POINT('Ctrl Pts',(66.2775624890064,247.291374580145,24.5226944240961)) ;
#109692=CARTESIAN_POINT('Ctrl Pts',(66.2729300042456,247.374926310296,24.5637023836631)) ;
#109693=CARTESIAN_POINT('Ctrl Pts',(66.2686688738934,247.451366986508,24.5944747791049)) ;
#109694=CARTESIAN_POINT('Ctrl Pts',(66.2587731205218,247.630559375766,24.6517146979187)) ;
#109695=CARTESIAN_POINT('Ctrl Pts',(66.2531111661463,247.734191361197,24.6743069365427)) ;
#109696=CARTESIAN_POINT('Ctrl Pts',(66.2465757706648,247.863019263849,24.6898531020637)) ;
#109697=CARTESIAN_POINT('Ctrl Pts',(66.2453890978721,247.886835529114,24.6922114595139)) ;
#109698=CARTESIAN_POINT('Ctrl Pts',(66.2434342945908,247.926972257001,24.6953204415881)) ;
#109699=CARTESIAN_POINT('Ctrl Pts',(66.242653548385,247.943266761729,24.6963436184616)) ;
#109700=CARTESIAN_POINT('Ctrl Pts',(66.2408608095576,247.981319477784,24.6981758461444)) ;
#109701=CARTESIAN_POINT('Ctrl Pts',(66.2398577550726,248.003082770755,24.6987995578256)) ;
#109702=CARTESIAN_POINT('Ctrl Pts',(66.2350509636585,248.109181875366,24.699774251177)) ;
#109703=CARTESIAN_POINT('Ctrl Pts',(66.2314849324052,248.193456178054,24.6941896580212)) ;
#109704=CARTESIAN_POINT('Ctrl Pts',(66.2234132367607,248.383057119953,24.6671709658645)) ;
#109705=CARTESIAN_POINT('Ctrl Pts',(66.2189212295562,248.487460871254,24.6419205868222)) ;
#109706=CARTESIAN_POINT('Ctrl Pts',(66.2125422512741,248.622542624032,24.5951937602889)) ;
#109707=CARTESIAN_POINT('Ctrl Pts',(66.2109172226369,248.655964213954,24.5824222134172)) ;
#109708=CARTESIAN_POINT('Ctrl Pts',(66.2079415574842,248.715144469431,24.5576112039242)) ;
#109709=CARTESIAN_POINT('Ctrl Pts',(66.2066038915539,248.741053969619,24.5459667350772)) ;
#109710=CARTESIAN_POINT('Ctrl Pts',(66.2035962932795,248.797705710801,24.5187566179239)) ;
#109711=CARTESIAN_POINT('Ctrl Pts',(66.2019168993095,248.828288674192,24.5028905640462)) ;
#109712=CARTESIAN_POINT('Ctrl Pts',(66.1954817284678,248.94153181943,24.4396428293417)) ;
#109713=CARTESIAN_POINT('Ctrl Pts',(66.1905288118633,249.020587385653,24.3861958647092)) ;
#109714=CARTESIAN_POINT('Ctrl Pts',(66.1802806195899,249.171752811789,24.2640593751003)) ;
#109715=CARTESIAN_POINT('Ctrl Pts',(66.1750012444952,249.243165919496,24.1950733020853)) ;
#109716=CARTESIAN_POINT('Ctrl Pts',(66.1688944934997,249.322877015503,24.1031070800742)) ;
#109717=CARTESIAN_POINT('Ctrl Pts',(66.1677776148412,249.337333631833,24.0857305937707)) ;
#109718=CARTESIAN_POINT('Ctrl Pts',(66.1658941588295,249.36159977872,24.0553344506698)) ;
#109719=CARTESIAN_POINT('Ctrl Pts',(66.16511750987,249.371577815513,24.0424554945693)) ;
#109720=CARTESIAN_POINT('Ctrl Pts',(66.1632757834583,249.395161333476,24.0110820600265)) ;
#109721=CARTESIAN_POINT('Ctrl Pts',(66.1622220061168,249.408577416785,23.9924503814133)) ;
#109722=CARTESIAN_POINT('Ctrl Pts',(66.1576468161301,249.466135375677,23.9089543776519)) ;
#109723=CARTESIAN_POINT('Ctrl Pts',(66.1543207900658,249.506081012181,23.8413116154289)) ;
#109724=CARTESIAN_POINT('Ctrl Pts',(66.1462641006527,249.59146658526,23.6703937581057)) ;
#109725=CARTESIAN_POINT('Ctrl Pts',(66.1415556208221,249.631517182786,23.5648621199517)) ;
#109726=CARTESIAN_POINT('Ctrl Pts',(66.1349394962132,249.669851065968,23.4219984157488)) ;
#109727=CARTESIAN_POINT('Ctrl Pts',(66.1333309432536,249.677926693574,23.3875957153835)) ;
#109728=CARTESIAN_POINT('Ctrl Pts',(66.1303708693538,249.690520215476,23.3251437116456)) ;
#109729=CARTESIAN_POINT('Ctrl Pts',(66.1290315545452,249.695423342456,23.2971856461358)) ;
#109730=CARTESIAN_POINT('Ctrl Pts',(66.1263670620569,249.703631006821,23.2422238340263)) ;
#109731=CARTESIAN_POINT('Ctrl Pts',(66.1250440486545,249.70699260088,23.2152374125494)) ;
#109732=CARTESIAN_POINT('Ctrl Pts',(66.1209327491675,249.71527946995,23.1323282828555)) ;
#109733=CARTESIAN_POINT('Ctrl Pts',(66.118085034826,249.718055118912,23.0762344201526)) ;
#109734=CARTESIAN_POINT('Ctrl Pts',(66.1151815854425,249.718014672093,23.0201112243472)) ;
#109735=CARTESIAN_POINT('Ctrl Pts',(66.1145741302299,249.716961070455,23.0201358258391)) ;
#109736=CARTESIAN_POINT('Ctrl Pts',(66.1062954533008,249.718173463304,22.8452907521841)) ;
#109737=CARTESIAN_POINT('Ctrl Pts',(66.0722432306643,249.614025132092,22.1275182747943)) ;
#109738=CARTESIAN_POINT('Ctrl Pts',(66.0124174623205,248.596941784018,21.1356001370716)) ;
#109739=CARTESIAN_POINT('Ctrl Pts',(65.9350968251983,246.796951235849,21.4981652426359)) ;
#109740=CARTESIAN_POINT('Ctrl Pts',(65.8577761880761,246.081263858291,23.1890860546867)) ;
#109741=CARTESIAN_POINT('Ctrl Pts',(65.8052102924027,246.756193730657,24.2391790716563)) ;
#109742=CARTESIAN_POINT('Ctrl Pts',(65.7784179424368,247.25196421432,24.5054393601585)) ;
#109743=CARTESIAN_POINT('Ctrl Pts',(65.7773991381782,247.271019322241,24.5151747855319)) ;
#109744=CARTESIAN_POINT('Origin',(67.8645744874958,248.040265107786,23.0213203435596)) ;
#109745=CARTESIAN_POINT('',(65.1788202510297,247.272170391302,24.5129220226313)) ;
#109746=CARTESIAN_POINT('',(65.2787248749179,247.272170391302,24.5129220226314)) ;
#109747=CARTESIAN_POINT('',(67.8645744874958,247.272170391302,24.5129220226314)) ;
#109748=CARTESIAN_POINT('',(65.5159557280774,249.717822745899,23.0208879934084)) ;
#109749=CARTESIAN_POINT('Ctrl Pts',(65.5159557280774,249.718015052066,23.0208879438461)) ;
#109750=CARTESIAN_POINT('Ctrl Pts',(65.5128383103028,249.717998033866,22.9548557931966)) ;
#109751=CARTESIAN_POINT('Ctrl Pts',(65.5097208925282,249.714078457698,22.8889248391981)) ;
#109752=CARTESIAN_POINT('Ctrl Pts',(65.5066034747536,249.706317429151,22.8235459140342)) ;
#109753=CARTESIAN_POINT('Ctrl Pts',(65.5034791103217,249.698539106417,22.7580213025946)) ;
#109754=CARTESIAN_POINT('Ctrl Pts',(65.5003547458898,249.686902320308,22.6930515529353)) ;
#109755=CARTESIAN_POINT('Ctrl Pts',(65.4972303814579,249.671519178825,22.6290765185997)) ;
#109756=CARTESIAN_POINT('Ctrl Pts',(65.4940947990912,249.656080804643,22.5648717838627)) ;
#109757=CARTESIAN_POINT('Ctrl Pts',(65.4909592167245,249.636869280332,22.5016692784945)) ;
#109758=CARTESIAN_POINT('Ctrl Pts',(65.4878236343579,249.614046703296,22.4398940351297)) ;
#109759=CARTESIAN_POINT('Ctrl Pts',(65.4857189454525,249.59872756348,22.3984287970561)) ;
#109760=CARTESIAN_POINT('Ctrl Pts',(65.4836142565472,249.581782486181,22.3576061933882)) ;
#109761=CARTESIAN_POINT('Ctrl Pts',(65.4815095676419,249.563272157893,22.317548656274)) ;
#109762=CARTESIAN_POINT('Ctrl Pts',(65.4785924797904,249.537616939375,22.2620291186446)) ;
#109763=CARTESIAN_POINT('Ctrl Pts',(65.4756753919389,249.508873303146,22.2078089745261)) ;
#109764=CARTESIAN_POINT('Ctrl Pts',(65.4727583040873,249.477195952274,22.1552517488974)) ;
#109765=CARTESIAN_POINT('Ctrl Pts',(65.4698460395561,249.445570978984,22.1027814251191)) ;
#109766=CARTESIAN_POINT('Ctrl Pts',(65.4669337750249,249.411022183956,22.0519689904515)) ;
#109767=CARTESIAN_POINT('Ctrl Pts',(65.4640215104936,249.373750954022,22.0031550522693)) ;
#109768=CARTESIAN_POINT('Ctrl Pts',(65.4611119374221,249.336514169453,21.9543862270041)) ;
#109769=CARTESIAN_POINT('Ctrl Pts',(65.4582023643506,249.296560244532,21.907612637462)) ;
#109770=CARTESIAN_POINT('Ctrl Pts',(65.455292791279,249.254133936172,21.8631461209263)) ;
#109771=CARTESIAN_POINT('Ctrl Pts',(65.4523848522289,249.211731454502,21.8187045768651)) ;
#109772=CARTESIAN_POINT('Ctrl Pts',(65.4494769131787,249.166859692877,21.7765679018234)) ;
#109773=CARTESIAN_POINT('Ctrl Pts',(65.4465689741286,249.119802454161,21.7370134564484)) ;
#109774=CARTESIAN_POINT('Ctrl Pts',(65.4436616139098,249.072754582287,21.697466884468)) ;
#109775=CARTESIAN_POINT('Ctrl Pts',(65.440754253691,249.023522485433,21.6605018469641)) ;
#109776=CARTESIAN_POINT('Ctrl Pts',(65.4378468934721,248.972423926319,21.6263561864822)) ;
#109777=CARTESIAN_POINT('Ctrl Pts',(65.4349370717318,248.921282104523,21.5921816165183)) ;
#109778=CARTESIAN_POINT('Ctrl Pts',(65.4320272499915,248.868271084647,21.5608314763569)) ;
#109779=CARTESIAN_POINT('Ctrl Pts',(65.4291174282511,248.813737561792,21.5325001981444)) ;
#109780=CARTESIAN_POINT('Ctrl Pts',(65.4262064361497,248.759182104976,21.5041575247916)) ;
#109781=CARTESIAN_POINT('Ctrl Pts',(65.4232954440482,248.703103386298,21.4788363449978)) ;
#109782=CARTESIAN_POINT('Ctrl Pts',(65.4203844519467,248.645869944603,21.4566836943262)) ;
#109783=CARTESIAN_POINT('Ctrl Pts',(65.4174682764158,248.588534590742,21.4344915977549)) ;
#109784=CARTESIAN_POINT('Ctrl Pts',(65.4145521008848,248.530040888254,21.4154794629481)) ;
#109785=CARTESIAN_POINT('Ctrl Pts',(65.4116359253539,248.470773655906,21.3997447355487)) ;
#109786=CARTESIAN_POINT('Ctrl Pts',(65.4091535937425,248.42032370088,21.3863508877483)) ;
#109787=CARTESIAN_POINT('Ctrl Pts',(65.4066712621311,248.369313663447,21.3753309846636)) ;
#109788=CARTESIAN_POINT('Ctrl Pts',(65.4041889305196,248.317984969375,21.3667156351839)) ;
#109789=CARTESIAN_POINT('Ctrl Pts',(65.4012720962684,248.257671797575,21.3565922711929)) ;
#109790=CARTESIAN_POINT('Ctrl Pts',(65.3983552620171,248.196690065062,21.3497517539178)) ;
#109791=CARTESIAN_POINT('Ctrl Pts',(65.3954384277659,248.135427179136,21.3462713166125)) ;
#109792=CARTESIAN_POINT('Ctrl Pts',(65.3925264077411,248.074265407425,21.3427966237589)) ;
#109793=CARTESIAN_POINT('Ctrl Pts',(65.3896143877162,248.012823906315,21.3426710261847)) ;
#109794=CARTESIAN_POINT('Ctrl Pts',(65.3867023676914,247.951497483721,21.3459202804649)) ;
#109795=CARTESIAN_POINT('Ctrl Pts',(65.3837930334048,247.89022762211,21.3491665379778)) ;
#109796=CARTESIAN_POINT('Ctrl Pts',(65.3808836991181,247.829073132597,21.3557814495652)) ;
#109797=CARTESIAN_POINT('Ctrl Pts',(65.3779743648315,247.768429519284,21.3657387311576)) ;
#109798=CARTESIAN_POINT('Ctrl Pts',(65.3750666584934,247.707819839741,21.3756904410486)) ;
#109799=CARTESIAN_POINT('Ctrl Pts',(65.3721589521552,247.647720968723,21.3889807291357)) ;
#109800=CARTESIAN_POINT('Ctrl Pts',(65.3692512458171,247.588521954332,21.4055316241388)) ;
#109801=CARTESIAN_POINT('Ctrl Pts',(65.3663441118793,247.52933459364,21.4220792609939)) ;
#109802=CARTESIAN_POINT('Ctrl Pts',(65.3634369779414,247.471047225645,21.4418860930771)) ;
#109803=CARTESIAN_POINT('Ctrl Pts',(65.3605298440036,247.414035409919,21.46482381995)) ;
#109804=CARTESIAN_POINT('Ctrl Pts',(65.3576202368912,247.356975092755,21.4877810605449)) ;
#109805=CARTESIAN_POINT('Ctrl Pts',(65.3547106297788,247.301192967862,21.5138743293845)) ;
#109806=CARTESIAN_POINT('Ctrl Pts',(65.3518010226664,247.24704505771,21.5429269538768)) ;
#109807=CARTESIAN_POINT('Ctrl Pts',(65.3488902390681,247.192875253107,21.5719913256603)) ;
#109808=CARTESIAN_POINT('Ctrl Pts',(65.3459794554698,247.140341415325,21.6040171760256)) ;
#109809=CARTESIAN_POINT('Ctrl Pts',(65.3430686718716,247.089772737581,21.6387830685893)) ;
#109810=CARTESIAN_POINT('Ctrl Pts',(65.3401526922266,247.039113789571,21.6736110218302)) ;
#109811=CARTESIAN_POINT('Ctrl Pts',(65.3372367125816,246.99042741484,21.7111884815772)) ;
#109812=CARTESIAN_POINT('Ctrl Pts',(65.3343207329366,246.944011029941,21.7512526054813)) ;
#109813=CARTESIAN_POINT('Ctrl Pts',(65.3318365864236,246.904468538313,21.7853835548748)) ;
#109814=CARTESIAN_POINT('Ctrl Pts',(65.3293524399105,246.866573031895,21.8213183879479)) ;
#109815=CARTESIAN_POINT('Ctrl Pts',(65.3268682933975,246.830486267395,21.8588745513426)) ;
#109816=CARTESIAN_POINT('Ctrl Pts',(65.3239534845639,246.78814334624,21.9029416127029)) ;
#109817=CARTESIAN_POINT('Ctrl Pts',(65.3210386757303,246.748130245474,21.9494095769339)) ;
#109818=CARTESIAN_POINT('Ctrl Pts',(65.3181238668967,246.710729112967,21.9980026504742)) ;
#109819=CARTESIAN_POINT('Ctrl Pts',(65.3152138828244,246.673389888992,22.0465152899298)) ;
#109820=CARTESIAN_POINT('Ctrl Pts',(65.3123038987521,246.63865435526,22.0971456540691)) ;
#109821=CARTESIAN_POINT('Ctrl Pts',(65.3093939146798,246.606766356824,22.1495827721025)) ;
#109822=CARTESIAN_POINT('Ctrl Pts',(65.3064866210556,246.574907840681,22.2019714089964)) ;
#109823=CARTESIAN_POINT('Ctrl Pts',(65.3035793274314,246.545891903166,22.25616305621)) ;
#109824=CARTESIAN_POINT('Ctrl Pts',(65.3006720338072,246.519919828641,22.3118167884718)) ;
#109825=CARTESIAN_POINT('Ctrl Pts',(65.2977663690951,246.493962305872,22.3674393387992)) ;
#109826=CARTESIAN_POINT('Ctrl Pts',(65.294860704383,246.471045477772,22.424521890027)) ;
#109827=CARTESIAN_POINT('Ctrl Pts',(65.2919550396709,246.451324316602,22.482699674988)) ;
#109828=CARTESIAN_POINT('Ctrl Pts',(65.2890499445796,246.43160702153,22.5408660548911)) ;
#109829=CARTESIAN_POINT('Ctrl Pts',(65.2861448494882,246.415084311733,22.6001267612825)) ;
#109830=CARTESIAN_POINT('Ctrl Pts',(65.2832397543969,246.401861995641,22.6600997674362)) ;
#109831=CARTESIAN_POINT('Ctrl Pts',(65.2803321655009,246.38862832919,22.7201242558858)) ;
#109832=CARTESIAN_POINT('Ctrl Pts',(65.2774245766048,246.378700827985,22.7808617691219)) ;
#109833=CARTESIAN_POINT('Ctrl Pts',(65.2745169877088,246.372134338007,22.8419191244501)) ;
#109834=CARTESIAN_POINT('Ctrl Pts',(65.2716082137543,246.365565171697,22.9030013651862)) ;
#109835=CARTESIAN_POINT('Ctrl Pts',(65.2686994397998,246.362359775844,22.964403199947)) ;
#109836=CARTESIAN_POINT('Ctrl Pts',(65.2657906658453,246.362520898481,23.0257283639149)) ;
#109837=CARTESIAN_POINT('Ctrl Pts',(65.2628766566017,246.362682311111,23.0871639025526)) ;
#109838=CARTESIAN_POINT('Ctrl Pts',(65.259962647358,246.366222321665,23.1485219860933)) ;
#109839=CARTESIAN_POINT('Ctrl Pts',(65.2570486381144,246.373091563555,23.2094092478441)) ;
#109840=CARTESIAN_POINT('Ctrl Pts',(65.2545483108347,246.378985626151,23.2616527614408)) ;
#109841=CARTESIAN_POINT('Ctrl Pts',(65.252047983555,246.387329856001,23.3135495519082)) ;
#109842=CARTESIAN_POINT('Ctrl Pts',(65.2495476562753,246.398063312116,23.3648582960463)) ;
#109843=CARTESIAN_POINT('Ctrl Pts',(65.2466006810568,246.410714147644,23.4253326182277)) ;
#109844=CARTESIAN_POINT('Ctrl Pts',(65.2436537058382,246.426733710662,23.4852213825265)) ;
#109845=CARTESIAN_POINT('Ctrl Pts',(65.2407067306196,246.446050225804,23.5441242958844)) ;
#109846=CARTESIAN_POINT('Ctrl Pts',(65.2377909266074,246.465162423286,23.6024041721524)) ;
#109847=CARTESIAN_POINT('Ctrl Pts',(65.2348751225951,246.487502027005,23.6597184543634)) ;
#109848=CARTESIAN_POINT('Ctrl Pts',(65.2319593185829,246.512948324416,23.7156894858295)) ;
#109849=CARTESIAN_POINT('Ctrl Pts',(65.2290462723041,246.538370555016,23.7716075805463)) ;
#109850=CARTESIAN_POINT('Ctrl Pts',(65.2261332260252,246.56689344367,23.8261844859753)) ;
#109851=CARTESIAN_POINT('Ctrl Pts',(65.2232201797464,246.598347602175,23.8790609625773)) ;
#109852=CARTESIAN_POINT('Ctrl Pts',(65.2203088400178,246.629783333888,23.9319064625492)) ;
#109853=CARTESIAN_POINT('Ctrl Pts',(65.2173975002891,246.664146669705,23.9830530769868)) ;
#109854=CARTESIAN_POINT('Ctrl Pts',(65.2144861605604,246.701222489793,24.0321664889742)) ;
#109855=CARTESIAN_POINT('Ctrl Pts',(65.2115140014328,246.739072843018,24.0823059056439)) ;
#109856=CARTESIAN_POINT('Ctrl Pts',(65.2085418423053,246.779750030088,24.1303257300894)) ;
#109857=CARTESIAN_POINT('Ctrl Pts',(65.2055696831777,246.822979955493,24.1759033507563)) ;
#109858=CARTESIAN_POINT('Ctrl Pts',(65.2026572829908,246.865340689703,24.2205645769067)) ;
#109859=CARTESIAN_POINT('Ctrl Pts',(65.1997448828038,246.910152044671,24.2628805765233)) ;
#109860=CARTESIAN_POINT('Ctrl Pts',(65.1968324826169,246.957118595572,24.3025848344348)) ;
#109861=CARTESIAN_POINT('Ctrl Pts',(65.193830444019,247.005530691974,24.3435111176029)) ;
#109862=CARTESIAN_POINT('Ctrl Pts',(65.1908284054212,247.056232409242,24.3816618563829)) ;
#109863=CARTESIAN_POINT('Ctrl Pts',(65.1878263668233,247.10886539866,24.4167914626949)) ;
#109864=CARTESIAN_POINT('Ctrl Pts',(65.1848243282255,247.161498388079,24.451921069007)) ;
#109865=CARTESIAN_POINT('Ctrl Pts',(65.1818222896276,247.216062125856,24.4840292807919)) ;
#109866=CARTESIAN_POINT('Ctrl Pts',(65.1788202510297,247.272170391302,24.5129220226314)) ;
#109867=CARTESIAN_POINT('Ctrl Pts',(65.6787784786721,247.273150902455,24.5110052762898)) ;
#109868=CARTESIAN_POINT('Ctrl Pts',(65.6645692664101,247.540740422681,24.6479503068636)) ;
#109869=CARTESIAN_POINT('Ctrl Pts',(65.6245865084408,248.393573021656,24.8412580942799)) ;
#109870=CARTESIAN_POINT('Ctrl Pts',(65.5703122582425,249.494912575159,24.1717753210047)) ;
#109871=CARTESIAN_POINT('Ctrl Pts',(65.5302472203063,249.715145368677,23.3232200710915)) ;
#109872=CARTESIAN_POINT('Ctrl Pts',(65.5159557280774,249.715873122799,23.0208884958769)) ;
#109873=CARTESIAN_POINT('',(65.6145744874959,249.719484537996,23.0224181452927)) ;
#109874=CARTESIAN_POINT('Ctrl Pts',(65.7773991381782,247.271019322241,24.5151747855319)) ;
#109875=CARTESIAN_POINT('Ctrl Pts',(65.7526443967294,247.734017259182,24.7517245800444)) ;
#109876=CARTESIAN_POINT('Ctrl Pts',(65.7021161095732,248.923660698597,24.7653398940284)) ;
#109877=CARTESIAN_POINT('Ctrl Pts',(65.6478412260124,249.679932032969,23.7216704578517)) ;
#109878=CARTESIAN_POINT('Ctrl Pts',(65.6183210839004,249.720089797457,23.1012396421188)) ;
#109879=CARTESIAN_POINT('Ctrl Pts',(65.6145744874959,249.719484537996,23.0224181452927)) ;
#109880=CARTESIAN_POINT('Ctrl Pts',(65.2787248749179,247.272170391302,24.5129220226314)) ;
#109881=CARTESIAN_POINT('Ctrl Pts',(65.2787251604049,247.272165032388,24.5129192630787)) ;
#109882=CARTESIAN_POINT('Ctrl Pts',(65.278725445891,247.272159673489,24.512916503497)) ;
#109883=CARTESIAN_POINT('Ctrl Pts',(65.2801133552695,247.246107015076,24.49950042904)) ;
#109884=CARTESIAN_POINT('Ctrl Pts',(65.2814781085148,247.220414718267,24.4854067141748)) ;
#109885=CARTESIAN_POINT('Ctrl Pts',(65.2848794516747,247.156328053296,24.4480351672425)) ;
#109886=CARTESIAN_POINT('Ctrl Pts',(65.2868854010309,247.118474008147,24.4238756659129)) ;
#109887=CARTESIAN_POINT('Ctrl Pts',(65.2913925336548,247.034042371573,24.3650924671633)) ;
#109888=CARTESIAN_POINT('Ctrl Pts',(65.2938636731129,246.988200616357,24.3295131520187)) ;
#109889=CARTESIAN_POINT('Ctrl Pts',(65.3010003376567,246.860303295283,24.2191684344408)) ;
#109890=CARTESIAN_POINT('Ctrl Pts',(65.3055809102225,246.783715368561,24.1385618226974)) ;
#109891=CARTESIAN_POINT('Ctrl Pts',(65.3116269153918,246.701398169249,24.0326657289751)) ;
#109892=CARTESIAN_POINT('Ctrl Pts',(65.3126918567843,246.687530974627,24.0140410709375)) ;
#109893=CARTESIAN_POINT('Ctrl Pts',(65.3145449454229,246.664596390981,23.981865094348)) ;
#109894=CARTESIAN_POINT('Ctrl Pts',(65.3153212784597,246.655332341131,23.9684591063175)) ;
#109895=CARTESIAN_POINT('Ctrl Pts',(65.3171919504421,246.633824620252,23.9363449278579)) ;
#109896=CARTESIAN_POINT('Ctrl Pts',(65.3182958844824,246.621757662664,23.9175242141664)) ;
#109897=CARTESIAN_POINT('Ctrl Pts',(65.3207803355331,246.595853010081,23.8752865730941)) ;
#109898=CARTESIAN_POINT('Ctrl Pts',(65.3221686027896,246.582201406051,23.8517628516253)) ;
#109899=CARTESIAN_POINT('Ctrl Pts',(65.3298577335332,246.510623849625,23.7212141198065)) ;
#109900=CARTESIAN_POINT('Ctrl Pts',(65.336411255635,246.463901164489,23.6084600415325)) ;
#109901=CARTESIAN_POINT('Ctrl Pts',(65.345663437879,246.413614234233,23.4362656595576)) ;
#109902=CARTESIAN_POINT('Ctrl Pts',(65.348576409491,246.400309053115,23.3800928278022)) ;
#109903=CARTESIAN_POINT('Ctrl Pts',(65.3529269233677,246.384336808603,23.2928155010469)) ;
#109904=CARTESIAN_POINT('Ctrl Pts',(65.3544238202099,246.379598112549,23.2621386009732)) ;
#109905=CARTESIAN_POINT('Ctrl Pts',(65.3572752977917,246.37207064708,23.2024800752714)) ;
#109906=CARTESIAN_POINT('Ctrl Pts',(65.3586324492277,246.369179785801,23.1735227491316)) ;
#109907=CARTESIAN_POINT('Ctrl Pts',(65.3619655614132,246.363849652597,23.1011226534158)) ;
#109908=CARTESIAN_POINT('Ctrl Pts',(65.3639137021724,246.362344080841,23.05763214007)) ;
#109909=CARTESIAN_POINT('Ctrl Pts',(65.3682449836589,246.362766770456,22.9590030410233)) ;
#109910=CARTESIAN_POINT('Ctrl Pts',(65.3706020249864,246.365719932988,22.9039195112528)) ;
#109911=CARTESIAN_POINT('Ctrl Pts',(65.3779883922573,246.383636634124,22.7303198055549)) ;
#109912=CARTESIAN_POINT('Ctrl Pts',(65.3828917689606,246.40853370839,22.613219200442)) ;
#109913=CARTESIAN_POINT('Ctrl Pts',(65.3892784100183,246.452384887201,22.4791468955633)) ;
#109914=CARTESIAN_POINT('Ctrl Pts',(65.3902771503213,246.459527437132,22.4586623801986)) ;
#109915=CARTESIAN_POINT('Ctrl Pts',(65.3920635401806,246.472729948615,22.4230358147814)) ;
#109916=CARTESIAN_POINT('Ctrl Pts',(65.3928423826101,246.478616937231,22.4078337534041)) ;
#109917=CARTESIAN_POINT('Ctrl Pts',(65.3947737097523,246.493531245029,22.3709266885103)) ;
#109918=CARTESIAN_POINT('Ctrl Pts',(65.3959380073934,246.502794473464,22.3493222034538)) ;
#109919=CARTESIAN_POINT('Ctrl Pts',(65.3985892806452,246.524575729568,22.301331906094)) ;
#109920=CARTESIAN_POINT('Ctrl Pts',(65.4000856119861,246.537335019653,22.2750639124343)) ;
#109921=CARTESIAN_POINT('Ctrl Pts',(65.4052595685095,246.583278770671,22.1864406222688)) ;
#109922=CARTESIAN_POINT('Ctrl Pts',(65.4090114474638,246.619711198304,22.1258541807603)) ;
#109923=CARTESIAN_POINT('Ctrl Pts',(65.4173111465078,246.709218627299,21.9962816305537)) ;
#109924=CARTESIAN_POINT('Ctrl Pts',(65.4218272120108,246.764063484794,21.9287540899728)) ;
#109925=CARTESIAN_POINT('Ctrl Pts',(65.4279623017477,246.848770742242,21.8395882949436)) ;
#109926=CARTESIAN_POINT('Ctrl Pts',(65.4297322298052,246.874485847982,21.8142128883417)) ;
#109927=CARTESIAN_POINT('Ctrl Pts',(65.4328341767626,246.921863363349,21.7703886016868)) ;
#109928=CARTESIAN_POINT('Ctrl Pts',(65.434178668651,246.943213088448,21.751623661276)) ;
#109929=CARTESIAN_POINT('Ctrl Pts',(65.4370937445044,246.991258376166,21.7115122065079)) ;
#109930=CARTESIAN_POINT('Ctrl Pts',(65.4386542991453,247.018150410036,21.6904205718303)) ;
#109931=CARTESIAN_POINT('Ctrl Pts',(65.4445965678961,247.124773141631,21.6119347870737)) ;
#109932=CARTESIAN_POINT('Ctrl Pts',(65.4487577439654,247.208841680642,21.5607622513343)) ;
#109933=CARTESIAN_POINT('Ctrl Pts',(65.4569526253967,247.383225950798,21.4745767918507)) ;
#109934=CARTESIAN_POINT('Ctrl Pts',(65.4609765818969,247.473050731389,21.4394287615949)) ;
#109935=CARTESIAN_POINT('Ctrl Pts',(65.4663537933726,247.587337636108,21.4057010584497)) ;
#109936=CARTESIAN_POINT('Ctrl Pts',(65.4674046480988,247.609420007946,21.3996726068345)) ;
#109937=CARTESIAN_POINT('Ctrl Pts',(65.4692435415761,247.647421883392,21.390129127431)) ;
#109938=CARTESIAN_POINT('Ctrl Pts',(65.4700204214036,247.663281139555,21.3863910994407)) ;
#109939=CARTESIAN_POINT('Ctrl Pts',(65.4719079220205,247.701339515509,21.3780039424865)) ;
#109940=CARTESIAN_POINT('Ctrl Pts',(65.4730287551434,247.723581797488,21.373573110626)) ;
#109941=CARTESIAN_POINT('Ctrl Pts',(65.4755595190611,247.773225000526,21.3647260443167)) ;
#109942=CARTESIAN_POINT('Ctrl Pts',(65.4769776308851,247.800659549744,21.3605361459666)) ;
#109943=CARTESIAN_POINT('Ctrl Pts',(65.4816986909607,247.891247202965,21.3489925524759)) ;
#109944=CARTESIAN_POINT('Ctrl Pts',(65.4850656301792,247.954714461548,21.3445474587606)) ;
#109945=CARTESIAN_POINT('Ctrl Pts',(65.4935234272992,248.114909464125,21.3424480098814)) ;
#109946=CARTESIAN_POINT('Ctrl Pts',(65.4985749878756,248.211477082246,21.3495327070713)) ;
#109947=CARTESIAN_POINT('Ctrl Pts',(65.5052113220985,248.342756622173,21.3706651342026)) ;
#109948=CARTESIAN_POINT('Ctrl Pts',(65.5069917015127,248.378413240225,21.3775990125917)) ;
#109949=CARTESIAN_POINT('Ctrl Pts',(65.510104566423,248.441530932365,21.3920140983603)) ;
#109950=CARTESIAN_POINT('Ctrl Pts',(65.5114498825721,248.469078979458,21.3990466676376)) ;
#109951=CARTESIAN_POINT('Ctrl Pts',(65.514358806751,248.529161377567,21.416022259653)) ;
#109952=CARTESIAN_POINT('Ctrl Pts',(65.5159126842182,248.561599106234,21.4262615548055)) ;
#109953=CARTESIAN_POINT('Ctrl Pts',(65.5218657125502,248.686749484563,21.469992704685)) ;
#109954=CARTESIAN_POINT('Ctrl Pts',(65.5260417031075,248.776752628797,21.5106425754533)) ;
#109955=CARTESIAN_POINT('Ctrl Pts',(65.5342601391638,248.946792333908,21.6062696522357)) ;
#109956=CARTESIAN_POINT('Ctrl Pts',(65.5382928781597,249.026670321995,21.6607462513169)) ;
#109957=CARTESIAN_POINT('Ctrl Pts',(65.5436796871986,249.119128040101,21.736243404269)) ;
#109958=CARTESIAN_POINT('Ctrl Pts',(65.5447295886078,249.136542013623,21.7510665005758)) ;
#109959=CARTESIAN_POINT('Ctrl Pts',(65.5465674037911,249.165834684351,21.7770520327555)) ;
#109960=CARTESIAN_POINT('Ctrl Pts',(65.5473441965105,249.177863027752,21.7880395822384)) ;
#109961=CARTESIAN_POINT('Ctrl Pts',(65.5492322487321,249.206258311595,21.8147467780886)) ;
#109962=CARTESIAN_POINT('Ctrl Pts',(65.5503537497323,249.222468918479,21.8306255961116)) ;
#109963=CARTESIAN_POINT('Ctrl Pts',(65.5528863816545,249.257793171086,21.8666594628687)) ;
#109964=CARTESIAN_POINT('Ctrl Pts',(65.5543057122949,249.27673841995,21.8869703245343)) ;
#109965=CARTESIAN_POINT('Ctrl Pts',(65.5590336541357,249.337436027233,21.9553711461487)) ;
#109966=CARTESIAN_POINT('Ctrl Pts',(65.5624064163098,249.376955019651,22.0053676825847)) ;
#109967=CARTESIAN_POINT('Ctrl Pts',(65.5708611051912,249.468958568187,22.136454546869)) ;
#109968=CARTESIAN_POINT('Ctrl Pts',(65.5759037432801,249.517471887109,22.2200613676321)) ;
#109969=CARTESIAN_POINT('Ctrl Pts',(65.58253208066,249.573986140451,22.3402449527344)) ;
#109970=CARTESIAN_POINT('Ctrl Pts',(65.5843125817513,249.588369220925,22.3736029778339)) ;
#109971=CARTESIAN_POINT('Ctrl Pts',(65.5874255138225,249.61206008712,22.4338566617689)) ;
#109972=CARTESIAN_POINT('Ctrl Pts',(65.5887707820689,249.621787599742,22.4605710632023)) ;
#109973=CARTESIAN_POINT('Ctrl Pts',(65.5916794326902,249.641650009961,22.5197552421261)) ;
#109974=CARTESIAN_POINT('Ctrl Pts',(65.5932330914424,249.651485988112,22.5523122334519)) ;
#109975=CARTESIAN_POINT('Ctrl Pts',(65.5991772599446,249.685899499949,22.6801329498468)) ;
#109976=CARTESIAN_POINT('Ctrl Pts',(65.6033456360179,249.703070745726,22.777188221211)) ;
#109977=CARTESIAN_POINT('Ctrl Pts',(65.6095610206486,249.71592081736,22.9241629434479)) ;
#109978=CARTESIAN_POINT('Ctrl Pts',(65.6116258859239,249.718047910538,22.9732975817688)) ;
#109979=CARTESIAN_POINT('Ctrl Pts',(65.6137281789529,249.718014725454,23.0224530012129)) ;
#109980=CARTESIAN_POINT('Origin',(61.8645744874958,248.040265107786,23.0213203435596)) ;
#109981=CARTESIAN_POINT('',(60.6787800750062,247.272018954284,24.5128440309777)) ;
#109982=CARTESIAN_POINT('',(60.7756980793888,247.272018954284,24.5128440309778)) ;
#109983=CARTESIAN_POINT('',(61.8645744874958,247.272018954284,24.5128440309778)) ;
#109984=CARTESIAN_POINT('',(60.940227675589,249.014561429937,21.655453681274)) ;
#109985=CARTESIAN_POINT('Ctrl Pts',(60.940227675589,249.014561429937,21.655453681274)) ;
#109986=CARTESIAN_POINT('Ctrl Pts',(60.9372127561583,248.963091283515,21.6187391353054)) ;
#109987=CARTESIAN_POINT('Ctrl Pts',(60.9341978367275,248.909424109754,21.5848535129617)) ;
#109988=CARTESIAN_POINT('Ctrl Pts',(60.9311829172968,248.853911725446,21.5540697705248)) ;
#109989=CARTESIAN_POINT('Ctrl Pts',(60.9283156924155,248.801118775861,21.5247940587582)) ;
#109990=CARTESIAN_POINT('Ctrl Pts',(60.9254484675342,248.746657684804,21.4983237503668)) ;
#109991=CARTESIAN_POINT('Ctrl Pts',(60.9225812426529,248.690862876965,21.4748509435263)) ;
#109992=CARTESIAN_POINT('Ctrl Pts',(60.9197165162814,248.635116688918,21.4513985909722)) ;
#109993=CARTESIAN_POINT('Ctrl Pts',(60.91685178991,248.578039567083,21.430938769325)) ;
#109994=CARTESIAN_POINT('Ctrl Pts',(60.9139870635385,248.519989426209,21.4136171244258)) ;
#109995=CARTESIAN_POINT('Ctrl Pts',(60.911123712368,248.461967152084,21.396303794716)) ;
#109996=CARTESIAN_POINT('Ctrl Pts',(60.9082603611976,248.402973286455,21.3821258056995)) ;
#109997=CARTESIAN_POINT('Ctrl Pts',(60.9053970100271,248.343382425444,21.3711794543516)) ;
#109998=CARTESIAN_POINT('Ctrl Pts',(60.9025339129334,248.283796852173,21.3602340743183)) ;
#109999=CARTESIAN_POINT('Ctrl Pts',(60.8996708158398,248.223614904701,21.3525198551716)) ;
#110000=CARTESIAN_POINT('Ctrl Pts',(60.8968077187462,248.163220700734,21.3480818714156)) ;
#110001=CARTESIAN_POINT('Ctrl Pts',(60.8939419153504,248.102769409998,21.343639692718)) ;
#110002=CARTESIAN_POINT('Ctrl Pts',(60.8910761119546,248.042105986334,21.3424799663762)) ;
#110003=CARTESIAN_POINT('Ctrl Pts',(60.8882103085588,247.981617458099,21.3445957043638)) ;
#110004=CARTESIAN_POINT('Ctrl Pts',(60.8853429246568,247.921095570111,21.3467126091925)) ;
#110005=CARTESIAN_POINT('Ctrl Pts',(60.8824755407547,247.860749291517,21.35210852332)) ;
#110006=CARTESIAN_POINT('Ctrl Pts',(60.8796081568527,247.800960246066,21.3607245933371)) ;
#110007=CARTESIAN_POINT('Ctrl Pts',(60.876735943038,247.741070490045,21.3693551765366)) ;
#110008=CARTESIAN_POINT('Ctrl Pts',(60.8738637292232,247.6817403521,21.3812166293377)) ;
#110009=CARTESIAN_POINT('Ctrl Pts',(60.8709915154085,247.623339591769,21.396199370649)) ;
#110010=CARTESIAN_POINT('Ctrl Pts',(60.8699508800227,247.602180339122,21.4016277864256)) ;
#110011=CARTESIAN_POINT('Ctrl Pts',(60.8689102446368,247.581142917275,21.407465464781)) ;
#110012=CARTESIAN_POINT('Ctrl Pts',(60.867869609251,247.560244271735,21.4137056324247)) ;
#110013=CARTESIAN_POINT('Ctrl Pts',(60.8649570713242,247.501752989794,21.4311706592527)) ;
#110014=CARTESIAN_POINT('Ctrl Pts',(60.8620445333974,247.444100412217,21.451866578102)) ;
#110015=CARTESIAN_POINT('Ctrl Pts',(60.8591319954706,247.387667546907,21.4756937761009)) ;
#110016=CARTESIAN_POINT('Ctrl Pts',(60.8561992107954,247.330842383862,21.4996866108386)) ;
#110017=CARTESIAN_POINT('Ctrl Pts',(60.8532664261202,247.275254476981,21.5268543518343)) ;
#110018=CARTESIAN_POINT('Ctrl Pts',(60.850333641445,247.221278510744,21.5570437247593)) ;
#110019=CARTESIAN_POINT('Ctrl Pts',(60.8474288575414,247.167817880227,21.5869448645441)) ;
#110020=CARTESIAN_POINT('Ctrl Pts',(60.8445240736378,247.115939000221,21.6198099425868)) ;
#110021=CARTESIAN_POINT('Ctrl Pts',(60.8416192897342,247.065984729456,21.6554423084112)) ;
#110022=CARTESIAN_POINT('Ctrl Pts',(60.8387162072254,247.016059717989,21.6910538035876)) ;
#110023=CARTESIAN_POINT('Ctrl Pts',(60.8358131247166,246.968057493728,21.7294290772779)) ;
#110024=CARTESIAN_POINT('Ctrl Pts',(60.8329100422078,246.922292452755,21.7703278555314)) ;
#110025=CARTESIAN_POINT('Ctrl Pts',(60.8300075968063,246.876537455328,21.8112176581835)) ;
#110026=CARTESIAN_POINT('Ctrl Pts',(60.8271051514049,246.833019045543,21.854629526766)) ;
#110027=CARTESIAN_POINT('Ctrl Pts',(60.8242027060034,246.792017410026,21.9002838822717)) ;
#110028=CARTESIAN_POINT('Ctrl Pts',(60.8212479107753,246.750276250343,21.9467616805193)) ;
#110029=CARTESIAN_POINT('Ctrl Pts',(60.8182931155471,246.711143946213,21.9955632832225)) ;
#110030=CARTESIAN_POINT('Ctrl Pts',(60.8153383203189,246.674874157318,22.0463574648406)) ;
#110031=CARTESIAN_POINT('Ctrl Pts',(60.8124321301431,246.639200990136,22.0963161050191)) ;
#110032=CARTESIAN_POINT('Ctrl Pts',(60.8095259399674,246.606297086554,22.1482017830271)) ;
#110033=CARTESIAN_POINT('Ctrl Pts',(60.8066197497916,246.576359287954,22.2016711422781)) ;
#110034=CARTESIAN_POINT('Ctrl Pts',(60.8036406520372,246.545670439949,22.2564818870804)) ;
#110035=CARTESIAN_POINT('Ctrl Pts',(60.8006615542829,246.518098805243,22.3129563487326)) ;
#110036=CARTESIAN_POINT('Ctrl Pts',(60.7976824565285,246.493804490034,22.3707016993125)) ;
#110037=CARTESIAN_POINT('Ctrl Pts',(60.7947033587741,246.469510174825,22.4284470498924)) ;
#110038=CARTESIAN_POINT('Ctrl Pts',(60.7917242610198,246.448493306057,22.4874627311267)) ;
#110039=CARTESIAN_POINT('Ctrl Pts',(60.7887451632654,246.430858864895,22.5473407998624)) ;
#110040=CARTESIAN_POINT('Ctrl Pts',(60.7858386217233,246.413653912243,22.6057605324766)) ;
#110041=CARTESIAN_POINT('Ctrl Pts',(60.7829320801812,246.399598409989,22.6652389656913)) ;
#110042=CARTESIAN_POINT('Ctrl Pts',(60.7800255386391,246.388817625871,22.7254043470751)) ;
#110043=CARTESIAN_POINT('Ctrl Pts',(60.7770920044158,246.377936721983,22.7861284766945)) ;
#110044=CARTESIAN_POINT('Ctrl Pts',(60.7741584701925,246.370391906018,22.847551900403)) ;
#110045=CARTESIAN_POINT('Ctrl Pts',(60.7712249359692,246.366260596378,22.9092758957446)) ;
#110046=CARTESIAN_POINT('Ctrl Pts',(60.7683263931628,246.362178565311,22.9702636426268)) ;
#110047=CARTESIAN_POINT('Ctrl Pts',(60.7654278503564,246.361429090042,23.0315443067775)) ;
#110048=CARTESIAN_POINT('Ctrl Pts',(60.7625293075499,246.364035269663,23.0927247711881)) ;
#110049=CARTESIAN_POINT('Ctrl Pts',(60.759632539937,246.366639853146,23.1538677660251)) ;
#110050=CARTESIAN_POINT('Ctrl Pts',(60.7567357723241,246.37259599498,23.2149101729716)) ;
#110051=CARTESIAN_POINT('Ctrl Pts',(60.7538390047112,246.381874709416,23.2754587882954)) ;
#110052=CARTESIAN_POINT('Ctrl Pts',(60.7509429373374,246.391151180896,23.3359927671289)) ;
#110053=CARTESIAN_POINT('Ctrl Pts',(60.7480468699636,246.403748553129,23.3960326860824)) ;
#110054=CARTESIAN_POINT('Ctrl Pts',(60.7451508025899,246.419586222929,23.4551924614458)) ;
#110055=CARTESIAN_POINT('Ctrl Pts',(60.7421899621474,246.435778116006,23.5156753967019)) ;
#110056=CARTESIAN_POINT('Ctrl Pts',(60.7392291217049,246.455356913336,23.5752377911731)) ;
#110057=CARTESIAN_POINT('Ctrl Pts',(60.7362682812624,246.478182388077,23.6334826090456)) ;
#110058=CARTESIAN_POINT('Ctrl Pts',(60.7333685507391,246.500536759107,23.6905252898268)) ;
#110059=CARTESIAN_POINT('Ctrl Pts',(60.7304688202159,246.526004774298,23.7463038198903)) ;
#110060=CARTESIAN_POINT('Ctrl Pts',(60.7275690896927,246.554406672558,23.8004671673109)) ;
#110061=CARTESIAN_POINT('Ctrl Pts',(60.7245776942905,246.58370639789,23.8563427002747)) ;
#110062=CARTESIAN_POINT('Ctrl Pts',(60.7215862988884,246.616128349212,23.9104986900731)) ;
#110063=CARTESIAN_POINT('Ctrl Pts',(60.7185949034863,246.651426535596,23.9625814565875)) ;
#110064=CARTESIAN_POINT('Ctrl Pts',(60.7156035080842,246.686724721981,24.0146642231019)) ;
#110065=CARTESIAN_POINT('Ctrl Pts',(60.712612112682,246.724898729234,24.0646733408183)) ;
#110066=CARTESIAN_POINT('Ctrl Pts',(60.7096207172799,246.765658802135,24.1122941416385)) ;
#110067=CARTESIAN_POINT('Ctrl Pts',(60.7067130024914,246.80527866204,24.1585828090228)) ;
#110068=CARTESIAN_POINT('Ctrl Pts',(60.703805287703,246.847504173481,24.2028048745381)) ;
#110069=CARTESIAN_POINT('Ctrl Pts',(60.7008975729145,246.892091487186,24.244652841067)) ;
#110070=CARTESIAN_POINT('Ctrl Pts',(60.6979937914438,246.936618486835,24.2864441991037)) ;
#110071=CARTESIAN_POINT('Ctrl Pts',(60.6950900099731,246.983500589642,24.32586747502)) ;
#110072=CARTESIAN_POINT('Ctrl Pts',(60.6921862285023,247.032454689335,24.3626492454181)) ;
#110073=CARTESIAN_POINT('Ctrl Pts',(60.6892856669198,247.081354505766,24.3993902299686)) ;
#110074=CARTESIAN_POINT('Ctrl Pts',(60.6863851053373,247.132321354308,24.4334952153625)) ;
#110075=CARTESIAN_POINT('Ctrl Pts',(60.6834845437548,247.185038029898,24.4647300940279)) ;
#110076=CARTESIAN_POINT('Ctrl Pts',(60.6819163875053,247.213538712241,24.4816168825995)) ;
#110077=CARTESIAN_POINT('Ctrl Pts',(60.6803482312557,247.242550279933,24.4976654616331)) ;
#110078=CARTESIAN_POINT('Ctrl Pts',(60.6787800750062,247.272018954284,24.5128440309778)) ;
#110079=CARTESIAN_POINT('',(60.9402651077866,247.065925086493,21.6554848536836)) ;
#110080=CARTESIAN_POINT('Origin',(60.9402651077866,248.040265107786,23.0213203435596)) ;
#110081=CARTESIAN_POINT('Ctrl Pts',(60.9402651077869,247.065925086493,21.6554848536831)) ;
#110082=CARTESIAN_POINT('Ctrl Pts',(60.9396867647248,247.055998640425,21.6625660386021)) ;
#110083=CARTESIAN_POINT('Ctrl Pts',(60.9391145488013,247.046149459394,21.6697553872395)) ;
#110084=CARTESIAN_POINT('Ctrl Pts',(60.9377470480283,247.022577449097,21.6873587177246)) ;
#110085=CARTESIAN_POINT('Ctrl Pts',(60.9369572365182,247.008934778977,21.6978780237137)) ;
#110086=CARTESIAN_POINT('Ctrl Pts',(60.9335105960238,246.949447707252,21.7452246655429)) ;
#110087=CARTESIAN_POINT('Ctrl Pts',(60.9309500858802,246.905393691192,21.7842389538113)) ;
#110088=CARTESIAN_POINT('Ctrl Pts',(60.92518819345,246.810011803345,21.8781017813637)) ;
#110089=CARTESIAN_POINT('Ctrl Pts',(60.9220089750807,246.760135358974,21.9342418382204)) ;
#110090=CARTESIAN_POINT('Ctrl Pts',(60.9170000430791,246.689467121177,22.0254199173532)) ;
#110091=CARTESIAN_POINT('Ctrl Pts',(60.9152280878726,246.665910284633,22.0581892549186)) ;
#110092=CARTESIAN_POINT('Ctrl Pts',(60.9119646114264,246.625515443228,22.1188853236253)) ;
#110093=CARTESIAN_POINT('Ctrl Pts',(60.910485682088,246.608266535942,22.1465143478789)) ;
#110094=CARTESIAN_POINT('Ctrl Pts',(60.9080063213577,246.581193941108,22.1928272329416)) ;
#110095=CARTESIAN_POINT('Ctrl Pts',(60.9070213098529,246.570899078315,22.211225946749)) ;
#110096=CARTESIAN_POINT('Ctrl Pts',(60.9050354726144,246.551079395075,22.2482685496161)) ;
#110097=CARTESIAN_POINT('Ctrl Pts',(60.9040349879792,246.541551405675,22.26690642732)) ;
#110098=CARTESIAN_POINT('Ctrl Pts',(60.9015011388585,246.518574142374,22.3140068144291)) ;
#110099=CARTESIAN_POINT('Ctrl Pts',(60.8999537124246,246.505572902896,22.342677947094)) ;
#110100=CARTESIAN_POINT('Ctrl Pts',(60.891820612325,246.442540613751,22.4927699565146)) ;
#110101=CARTESIAN_POINT('Ctrl Pts',(60.8848046578023,246.406091410028,22.6193796112316)) ;
#110102=CARTESIAN_POINT('Ctrl Pts',(60.873091660205,246.370638855896,22.8348390986218)) ;
#110103=CARTESIAN_POINT('Ctrl Pts',(60.8684410143515,246.363210501457,22.9217354108926)) ;
#110104=CARTESIAN_POINT('Ctrl Pts',(60.8631745389201,246.362429865603,23.0265114899575)) ;
#110105=CARTESIAN_POINT('Ctrl Pts',(60.8622971625612,246.362577881107,23.0442040284292)) ;
#110106=CARTESIAN_POINT('Ctrl Pts',(60.860896988545,246.363271947923,23.0728975400407)) ;
#110107=CARTESIAN_POINT('Ctrl Pts',(60.8603654784424,246.363646504033,23.0839009961984)) ;
#110108=CARTESIAN_POINT('Ctrl Pts',(60.8592973572389,246.364628201922,23.1062638624013)) ;
#110109=CARTESIAN_POINT('Ctrl Pts',(60.8587611606733,246.36524260645,23.1176223426978)) ;
#110110=CARTESIAN_POINT('Ctrl Pts',(60.8573069279922,246.367244052481,23.14875000601)) ;
#110111=CARTESIAN_POINT('Ctrl Pts',(60.8564009465218,246.368865938047,23.168502693823)) ;
#110112=CARTESIAN_POINT('Ctrl Pts',(60.852477944768,246.377539470122,23.2552590034297)) ;
#110113=CARTESIAN_POINT('Ctrl Pts',(60.8496135629811,246.388273699,23.3218357141254)) ;
#110114=CARTESIAN_POINT('Ctrl Pts',(60.8443246245783,246.415756471825,23.4446878375553)) ;
#110115=CARTESIAN_POINT('Ctrl Pts',(60.841895438994,246.431507497226,23.5010778840882)) ;
#110116=CARTESIAN_POINT('Ctrl Pts',(60.8363359680186,246.473521197085,23.6258994598745)) ;
#110117=CARTESIAN_POINT('Ctrl Pts',(60.8331866541431,246.501383272451,23.6936624628327)) ;
#110118=CARTESIAN_POINT('Ctrl Pts',(60.8287680082623,246.544564766011,23.7818130819286)) ;
#110119=CARTESIAN_POINT('Ctrl Pts',(60.8276280218364,246.556049771089,23.8039910764275)) ;
#110120=CARTESIAN_POINT('Ctrl Pts',(60.8256301604299,246.576719212668,23.8418123561527)) ;
#110121=CARTESIAN_POINT('Ctrl Pts',(60.8247807287349,246.585670321803,23.8575785016638)) ;
#110122=CARTESIAN_POINT('Ctrl Pts',(60.8230019298047,246.604733888494,23.8899239347454)) ;
#110123=CARTESIAN_POINT('Ctrl Pts',(60.8220713071847,246.614882187956,23.9064788446261)) ;
#110124=CARTESIAN_POINT('Ctrl Pts',(60.8195773404605,246.642520506606,23.9498569892743)) ;
#110125=CARTESIAN_POINT('Ctrl Pts',(60.8179957968244,246.66049440445,23.9763611276772)) ;
#110126=CARTESIAN_POINT('Ctrl Pts',(60.8096084557132,246.75807404293,24.1117423521865)) ;
#110127=CARTESIAN_POINT('Ctrl Pts',(60.8023153144641,246.849829528678,24.2112309089791)) ;
#110128=CARTESIAN_POINT('Ctrl Pts',(60.792432542256,246.990100397675,24.3306869456728)) ;
#110129=CARTESIAN_POINT('Ctrl Pts',(60.7898016721395,247.029119870425,24.3610488833073)) ;
#110130=CARTESIAN_POINT('Ctrl Pts',(60.7861158787418,247.087115783232,24.4021975944882)) ;
#110131=CARTESIAN_POINT('Ctrl Pts',(60.7850053541749,247.105049846946,24.4144061643936)) ;
#110132=CARTESIAN_POINT('Ctrl Pts',(60.7830396281911,247.137750903115,24.4357511248514)) ;
#110133=CARTESIAN_POINT('Ctrl Pts',(60.7821778845666,247.152432438562,24.4450125580265)) ;
#110134=CARTESIAN_POINT('Ctrl Pts',(60.7808134620318,247.176302589428,24.4595574822181)) ;
#110135=CARTESIAN_POINT('Ctrl Pts',(60.7803018029719,247.18540183663,24.4649844698352)) ;
#110136=CARTESIAN_POINT('Ctrl Pts',(60.779265837799,247.20414302895,24.4759227777364)) ;
#110137=CARTESIAN_POINT('Ctrl Pts',(60.7787419818932,247.213789109344,24.4814250688233)) ;
#110138=CARTESIAN_POINT('Ctrl Pts',(60.7773672882245,247.239521947716,24.4957667959593)) ;
#110139=CARTESIAN_POINT('Ctrl Pts',(60.7765263339732,247.255700655054,24.5044388874851)) ;
#110140=CARTESIAN_POINT('Ctrl Pts',(60.7756980793889,247.272018954284,24.5128440309776)) ;
#110141=CARTESIAN_POINT('Origin',(61.8645744874958,248.040265107786,23.0213203435596)) ;
#110142=CARTESIAN_POINT('',(60.178415027332,247.272018800728,24.5128439518851)) ;
#110143=CARTESIAN_POINT('',(60.2784744057375,247.272018982637,24.5128440455817)) ;
#110144=CARTESIAN_POINT('',(61.8645744874958,247.272018954284,24.5128440309778)) ;
#110145=CARTESIAN_POINT('',(60.5159557281095,249.718015041886,23.0217905853416)) ;
#110146=CARTESIAN_POINT('Ctrl Pts',(60.178415027332,247.272018800728,24.5128439518851)) ;
#110147=CARTESIAN_POINT('Ctrl Pts',(60.1811705889247,247.213831808876,24.4828732954635)) ;
#110148=CARTESIAN_POINT('Ctrl Pts',(60.1839757745729,247.157415788768,24.4495065124652)) ;
#110149=CARTESIAN_POINT('Ctrl Pts',(60.1882301766301,247.078122707203,24.3961045007148)) ;
#110150=CARTESIAN_POINT('Ctrl Pts',(60.1895902049024,247.053635880327,24.3786383312463)) ;
#110151=CARTESIAN_POINT('Ctrl Pts',(60.191868695306,247.014142009741,24.3488342070395)) ;
#110152=CARTESIAN_POINT('Ctrl Pts',(60.1927724821908,246.998855964066,24.3368767384678)) ;
#110153=CARTESIAN_POINT('Ctrl Pts',(60.1945815551,246.969028882844,24.3126989245764)) ;
#110154=CARTESIAN_POINT('Ctrl Pts',(60.1954862600071,246.954481119213,24.300491474847)) ;
#110155=CARTESIAN_POINT('Ctrl Pts',(60.1977392628852,246.919169348636,24.2698238983159)) ;
#110156=CARTESIAN_POINT('Ctrl Pts',(60.1990987197496,246.898651165582,24.2510903713293)) ;
#110157=CARTESIAN_POINT('Ctrl Pts',(60.2059852468756,246.798617310351,24.1550957229905)) ;
#110158=CARTESIAN_POINT('Ctrl Pts',(60.2118247025089,246.726441138572,24.0706042579183)) ;
#110159=CARTESIAN_POINT('Ctrl Pts',(60.2224827440213,246.612126515002,23.9063284304355)) ;
#110160=CARTESIAN_POINT('Ctrl Pts',(60.2272541985357,246.567051464706,23.8290718136566)) ;
#110161=CARTESIAN_POINT('Ctrl Pts',(60.2327745233088,246.519648160462,23.7305248824824)) ;
#110162=CARTESIAN_POINT('Ctrl Pts',(60.2337724854315,246.511281990191,23.7123034604854)) ;
#110163=CARTESIAN_POINT('Ctrl Pts',(60.2353124276838,246.498653815277,23.6834463022867)) ;
#110164=CARTESIAN_POINT('Ctrl Pts',(60.2358663507129,246.494170896116,23.6729098345444)) ;
#110165=CARTESIAN_POINT('Ctrl Pts',(60.2369372579101,246.485611802032,23.6522071026085)) ;
#110166=CARTESIAN_POINT('Ctrl Pts',(60.2374546879911,246.481526686834,23.6420453585046)) ;
#110167=CARTESIAN_POINT('Ctrl Pts',(60.2387894501942,246.471135165012,23.6154467612984)) ;
#110168=CARTESIAN_POINT('Ctrl Pts',(60.239597986921,246.464987280693,23.5989489330212)) ;
#110169=CARTESIAN_POINT('Ctrl Pts',(60.2441819501055,246.431114055562,23.5034842683512)) ;
#110170=CARTESIAN_POINT('Ctrl Pts',(60.2476991211754,246.409066403289,23.4226211171969)) ;
#110171=CARTESIAN_POINT('Ctrl Pts',(60.2560977517516,246.370794914273,23.2250876269592)) ;
#110172=CARTESIAN_POINT('Ctrl Pts',(60.260953232974,246.360625820245,23.1077034773157)) ;
#110173=CARTESIAN_POINT('Ctrl Pts',(60.2675013718757,246.36334880304,22.9607937346077)) ;
#110174=CARTESIAN_POINT('Ctrl Pts',(60.268834271811,246.364669003289,22.9313795871221)) ;
#110175=CARTESIAN_POINT('Ctrl Pts',(60.2710798620106,246.368133877454,22.8827770579642)) ;
#110176=CARTESIAN_POINT('Ctrl Pts',(60.2719787780596,246.36983708027,22.8635633732702)) ;
#110177=CARTESIAN_POINT('Ctrl Pts',(60.2737879069914,246.373883861288,22.8254049236208)) ;
#110178=CARTESIAN_POINT('Ctrl Pts',(60.2746977671713,246.376220246872,22.806462310032)) ;
#110179=CARTESIAN_POINT('Ctrl Pts',(60.2769831638854,246.382825443789,22.7595169007374)) ;
#110180=CARTESIAN_POINT('Ctrl Pts',(60.2783705875292,246.387481110738,22.7315752457179)) ;
#110181=CARTESIAN_POINT('Ctrl Pts',(60.2842982973178,246.410041152097,22.6145372652656)) ;
#110182=CARTESIAN_POINT('Ctrl Pts',(60.2890358102792,246.434459543021,22.5268631904767)) ;
#110183=CARTESIAN_POINT('Ctrl Pts',(60.2996583956505,246.503619773932,22.3390349618594)) ;
#110184=CARTESIAN_POINT('Ctrl Pts',(60.3055593102924,246.551321389504,22.2403974576678)) ;
#110185=CARTESIAN_POINT('Ctrl Pts',(60.3120451237019,246.618380286035,22.130554177403)) ;
#110186=CARTESIAN_POINT('Ctrl Pts',(60.31300866222,246.628767127593,22.1141851172961)) ;
#110187=CARTESIAN_POINT('Ctrl Pts',(60.3145080453651,246.645662011748,22.0885528124602)) ;
#110188=CARTESIAN_POINT('Ctrl Pts',(60.3150548807429,246.651983874632,22.0791694567574)) ;
#110189=CARTESIAN_POINT('Ctrl Pts',(60.3161235023812,246.664671823486,22.0607421463588)) ;
#110190=CARTESIAN_POINT('Ctrl Pts',(60.3166455009921,246.671033320294,22.051695840326)) ;
#110191=CARTESIAN_POINT('Ctrl Pts',(60.3180089703817,246.688064867842,22.027978185396)) ;
#110192=CARTESIAN_POINT('Ctrl Pts',(60.3188409069329,246.698884480097,22.0134154920811)) ;
#110193=CARTESIAN_POINT('Ctrl Pts',(60.3206890541358,246.723812832313,21.9809757150205)) ;
#110194=CARTESIAN_POINT('Ctrl Pts',(60.3216979336936,246.738053743316,21.963204484442)) ;
#110195=CARTESIAN_POINT('Ctrl Pts',(60.3250061150887,246.78661993943,21.905064935095)) ;
#110196=CARTESIAN_POINT('Ctrl Pts',(60.3272403118247,246.822496100017,21.8660318697313)) ;
#110197=CARTESIAN_POINT('Ctrl Pts',(60.3347604134617,246.950303633682,21.7395591581177)) ;
#110198=CARTESIAN_POINT('Ctrl Pts',(60.3399709896441,247.050262283888,21.6608716316085)) ;
#110199=CARTESIAN_POINT('Ctrl Pts',(60.3469015939312,247.182198562016,21.5793191472611)) ;
#110200=CARTESIAN_POINT('Ctrl Pts',(60.3481854385056,247.206638058707,21.5650540615996)) ;
#110201=CARTESIAN_POINT('Ctrl Pts',(60.3502840909381,247.246474995144,21.5431331519946)) ;
#110202=CARTESIAN_POINT('Ctrl Pts',(60.351084852309,247.26165011277,21.5350838953927)) ;
#110203=CARTESIAN_POINT('Ctrl Pts',(60.3527858571736,247.293810892603,21.5186527685344)) ;
#110204=CARTESIAN_POINT('Ctrl Pts',(60.3536877568611,247.310820195851,21.5103227191475)) ;
#110205=CARTESIAN_POINT('Ctrl Pts',(60.3559229685263,247.352848697118,21.4906149504757)) ;
#110206=CARTESIAN_POINT('Ctrl Pts',(60.3572670441465,247.378012866435,21.4795609001742)) ;
#110207=CARTESIAN_POINT('Ctrl Pts',(60.3634639044702,247.493513829258,21.4321734444685)) ;
#110208=CARTESIAN_POINT('Ctrl Pts',(60.3685504548122,247.586627091968,21.403132035691)) ;
#110209=CARTESIAN_POINT('Ctrl Pts',(60.3793636933516,247.785424136848,21.35964350066)) ;
#110210=CARTESIAN_POINT('Ctrl Pts',(60.3850818917271,247.891049231485,21.3468501489587)) ;
#110211=CARTESIAN_POINT('Ctrl Pts',(60.3913544923533,248.015741089614,21.3436468202095)) ;
#110212=CARTESIAN_POINT('Ctrl Pts',(60.3922758013978,248.034311530069,21.3434781326632)) ;
#110213=CARTESIAN_POINT('Ctrl Pts',(60.393725341286,248.064027634494,21.3437016008822)) ;
#110214=CARTESIAN_POINT('Ctrl Pts',(60.39426343295,248.075172867825,21.3438964955723)) ;
#110215=CARTESIAN_POINT('Ctrl Pts',(60.395330569705,248.097531247299,21.3445104150266)) ;
#110216=CARTESIAN_POINT('Ctrl Pts',(60.3958595175572,248.108743767186,21.3449308801168)) ;
#110217=CARTESIAN_POINT('Ctrl Pts',(60.3972650958725,248.138851398337,21.3463624875682)) ;
#110218=CARTESIAN_POINT('Ctrl Pts',(60.3981310897179,248.157735420768,21.3475808617472)) ;
#110219=CARTESIAN_POINT('Ctrl Pts',(60.4024502929226,248.253264443539,21.3553690986169)) ;
#110220=CARTESIAN_POINT('Ctrl Pts',(60.4056949701534,248.329419110123,21.3668856789759)) ;
#110221=CARTESIAN_POINT('Ctrl Pts',(60.4140548037342,248.524691430933,21.4103169502864)) ;
#110222=CARTESIAN_POINT('Ctrl Pts',(60.4191244793235,248.641547874058,21.4501875437323)) ;
#110223=CARTESIAN_POINT('Ctrl Pts',(60.425903326889,248.779041935032,21.5147075856406)) ;
#110224=CARTESIAN_POINT('Ctrl Pts',(60.4272078751849,248.804773819481,21.5276003158052)) ;
#110225=CARTESIAN_POINT('Ctrl Pts',(60.429419345957,248.84707229154,21.5501729392805)) ;
#110226=CARTESIAN_POINT('Ctrl Pts',(60.4303134226966,248.863827613651,21.559486810022)) ;
#110227=CARTESIAN_POINT('Ctrl Pts',(60.4321238349279,248.897042112574,21.5787022282945)) ;
#110228=CARTESIAN_POINT('Ctrl Pts',(60.433040071941,248.913498152863,21.5886033882758)) ;
#110229=CARTESIAN_POINT('Ctrl Pts',(60.4353642952565,248.954343588767,21.6141441399071)) ;
#110230=CARTESIAN_POINT('Ctrl Pts',(60.436785047033,248.97850398986,21.6301366714241)) ;
#110231=CARTESIAN_POINT('Ctrl Pts',(60.4421684081947,249.067064902063,21.6921145110272)) ;
#110232=CARTESIAN_POINT('Ctrl Pts',(60.4462721951324,249.128595431866,21.7420076747762)) ;
#110233=CARTESIAN_POINT('Ctrl Pts',(60.4568123768335,249.274166564319,21.8781736391898)) ;
#110234=CARTESIAN_POINT('Ctrl Pts',(60.4633375740573,249.352881552832,21.9694950356638)) ;
#110235=CARTESIAN_POINT('Ctrl Pts',(60.4703539246244,249.432010599461,22.0841680348933)) ;
#110236=CARTESIAN_POINT('Ctrl Pts',(60.4713028533939,249.442590869066,22.1000752741307)) ;
#110237=CARTESIAN_POINT('Ctrl Pts',(60.4727850108929,249.458970246633,22.1256376491726)) ;
#110238=CARTESIAN_POINT('Ctrl Pts',(60.4733288340088,249.464947581473,22.1351760989331)) ;
#110239=CARTESIAN_POINT('Ctrl Pts',(60.4743964479814,249.476629760029,22.1542419506994)) ;
#110240=CARTESIAN_POINT('Ctrl Pts',(60.474920351834,249.482336882512,22.1637672198921)) ;
#110241=CARTESIAN_POINT('Ctrl Pts',(60.4762964678703,249.497238432476,22.1892076156252)) ;
#110242=CARTESIAN_POINT('Ctrl Pts',(60.4771388026686,249.50626683707,22.2052187333813)) ;
#110243=CARTESIAN_POINT('Ctrl Pts',(60.4814826501672,249.552151512365,22.2898109894164)) ;
#110244=CARTESIAN_POINT('Ctrl Pts',(60.4847667762189,249.584466937395,22.3607531136743)) ;
#110245=CARTESIAN_POINT('Ctrl Pts',(60.4908119799773,249.635139035958,22.4962628569805)) ;
#110246=CARTESIAN_POINT('Ctrl Pts',(60.4935758249554,249.654779644228,22.5601794688302)) ;
#110247=CARTESIAN_POINT('Ctrl Pts',(60.4991576355374,249.68587489522,22.6881228634387)) ;
#110248=CARTESIAN_POINT('Ctrl Pts',(60.5019671094267,249.697524210488,22.7519813499238)) ;
#110249=CARTESIAN_POINT('Ctrl Pts',(60.5059970770317,249.708452116705,22.8407600485552)) ;
#110250=CARTESIAN_POINT('Ctrl Pts',(60.5071204011434,249.710919546307,22.8652319318812)) ;
#110251=CARTESIAN_POINT('Ctrl Pts',(60.5091055429909,249.714277774323,22.9079227996584)) ;
#110252=CARTESIAN_POINT('Ctrl Pts',(60.5099596821151,249.715411080149,22.9261187119359)) ;
#110253=CARTESIAN_POINT('Ctrl Pts',(60.5114560893805,249.716860866305,22.9576783431437)) ;
#110254=CARTESIAN_POINT('Ctrl Pts',(60.5120939908299,249.717314580784,22.9710342204351)) ;
#110255=CARTESIAN_POINT('Ctrl Pts',(60.5133377228246,249.717883585693,22.9968806246684)) ;
#110256=CARTESIAN_POINT('Ctrl Pts',(60.513942882745,249.718019031575,23.0093697979911)) ;
#110257=CARTESIAN_POINT('Ctrl Pts',(60.5145522989917,249.718015021295,23.0218590659304)) ;
#110258=CARTESIAN_POINT('Ctrl Pts',(60.6787800750062,247.272018954284,24.5128440309778)) ;
#110259=CARTESIAN_POINT('Ctrl Pts',(60.6758817378808,247.326484287654,24.5408977475989)) ;
#110260=CARTESIAN_POINT('Ctrl Pts',(60.6729834007554,247.382512350534,24.5659766848025)) ;
#110261=CARTESIAN_POINT('Ctrl Pts',(60.67008506363,247.439744604203,24.5879154371548)) ;
#110262=CARTESIAN_POINT('Ctrl Pts',(60.6671868492106,247.496974434847,24.6098532606924)) ;
#110263=CARTESIAN_POINT('Ctrl Pts',(60.6642886347913,247.55540787763,24.6286509827448)) ;
#110264=CARTESIAN_POINT('Ctrl Pts',(60.6613904203719,247.61466777786,24.6441918650485)) ;
#110265=CARTESIAN_POINT('Ctrl Pts',(60.6584892760978,247.673987584943,24.6597484578976)) ;
#110266=CARTESIAN_POINT('Ctrl Pts',(60.6555881318236,247.734135022389,24.6720415091348)) ;
#110267=CARTESIAN_POINT('Ctrl Pts',(60.6526869875494,247.794720421271,24.6810049128149)) ;
#110268=CARTESIAN_POINT('Ctrl Pts',(60.6497842408534,247.855339283972,24.6899732673532)) ;
#110269=CARTESIAN_POINT('Ctrl Pts',(60.6468814941574,247.916396080965,24.6956082659881)) ;
#110270=CARTESIAN_POINT('Ctrl Pts',(60.6439787474614,247.977496717446,24.6978957792839)) ;
#110271=CARTESIAN_POINT('Ctrl Pts',(60.641070832045,248.038706151607,24.7001873657965)) ;
#110272=CARTESIAN_POINT('Ctrl Pts',(60.6381629166285,248.099959070422,24.6991195769611)) ;
#110273=CARTESIAN_POINT('Ctrl Pts',(60.6352550012121,248.160863169467,24.6947303859637)) ;
#110274=CARTESIAN_POINT('Ctrl Pts',(60.6336687579062,248.194085841236,24.6923361193359)) ;
#110275=CARTESIAN_POINT('Ctrl Pts',(60.6320825146003,248.227204831506,24.6889544394523)) ;
#110276=CARTESIAN_POINT('Ctrl Pts',(60.6304962712944,248.260157771901,24.684597914733)) ;
#110277=CARTESIAN_POINT('Ctrl Pts',(60.627587417587,248.320586889225,24.6766089176896)) ;
#110278=CARTESIAN_POINT('Ctrl Pts',(60.6246785638795,248.38070298245,24.6653061876332)) ;
#110279=CARTESIAN_POINT('Ctrl Pts',(60.6217697101721,248.440114926134,24.6507267340181)) ;
#110280=CARTESIAN_POINT('Ctrl Pts',(60.6188364649694,248.500025054425,24.6360250278909)) ;
#110281=CARTESIAN_POINT('Ctrl Pts',(60.6159032197668,248.559218639349,24.6179913754864)) ;
#110282=CARTESIAN_POINT('Ctrl Pts',(60.6129699745642,248.617300469956,24.5967171993725)) ;
#110283=CARTESIAN_POINT('Ctrl Pts',(60.6100690397587,248.674742515314,24.5756773633943)) ;
#110284=CARTESIAN_POINT('Ctrl Pts',(60.6071681049532,248.731096683785,24.5514682099505)) ;
#110285=CARTESIAN_POINT('Ctrl Pts',(60.6042671701477,248.78599392584,24.52422872148)) ;
#110286=CARTESIAN_POINT('Ctrl Pts',(60.6013679874107,248.840858011781,24.497005684758)) ;
#110287=CARTESIAN_POINT('Ctrl Pts',(60.5984688046737,248.894266459826,24.4667561685163)) ;
#110288=CARTESIAN_POINT('Ctrl Pts',(60.5955696219366,248.94587133027,24.4336667714231)) ;
#110289=CARTESIAN_POINT('Ctrl Pts',(60.5926711203359,248.997464076625,24.4005851483787)) ;
#110290=CARTESIAN_POINT('Ctrl Pts',(60.5897726187351,249.047253657176,24.3646652444936)) ;
#110291=CARTESIAN_POINT('Ctrl Pts',(60.5868741171344,249.094919624155,24.3261379222279)) ;
#110292=CARTESIAN_POINT('Ctrl Pts',(60.5839155928156,249.143572666972,24.2868127689035)) ;
#110293=CARTESIAN_POINT('Ctrl Pts',(60.5809570684968,249.190012693819,24.244771299182)) ;
#110294=CARTESIAN_POINT('Ctrl Pts',(60.577998544178,249.233934908198,24.2003018828912)) ;
#110295=CARTESIAN_POINT('Ctrl Pts',(60.5750963603741,249.27702069201,24.1566793177811)) ;
#110296=CARTESIAN_POINT('Ctrl Pts',(60.5721941765702,249.317683431554,24.1107209130333)) ;
#110297=CARTESIAN_POINT('Ctrl Pts',(60.5692919927664,249.355674923129,24.0627338446237)) ;
#110298=CARTESIAN_POINT('Ctrl Pts',(60.5663052981901,249.394772716206,24.0133494063403)) ;
#110299=CARTESIAN_POINT('Ctrl Pts',(60.5633186036139,249.431040904279,23.9618167711563)) ;
#110300=CARTESIAN_POINT('Ctrl Pts',(60.5603319090376,249.464257260494,23.9085020676312)) ;
#110301=CARTESIAN_POINT('Ctrl Pts',(60.5573452144614,249.497473616709,23.8551873641062)) ;
#110302=CARTESIAN_POINT('Ctrl Pts',(60.5543585198851,249.527637922912,23.8000911356975)) ;
#110303=CARTESIAN_POINT('Ctrl Pts',(60.5513718253088,249.554580836769,23.7436034843402)) ;
#110304=CARTESIAN_POINT('Ctrl Pts',(60.5482383900215,249.582847495735,23.6843405113292)) ;
#110305=CARTESIAN_POINT('Ctrl Pts',(60.5451049547341,249.60767069774,23.6233339249503)) ;
#110306=CARTESIAN_POINT('Ctrl Pts',(60.5419715194467,249.628850532698,23.5609882138808)) ;
#110307=CARTESIAN_POINT('Ctrl Pts',(60.5388459790484,249.649977003717,23.4987995867887)) ;
#110308=CARTESIAN_POINT('Ctrl Pts',(60.5357204386502,249.667478246505,23.4352789068086)) ;
#110309=CARTESIAN_POINT('Ctrl Pts',(60.5325948982519,249.681201746002,23.3708514750201)) ;
#110310=CARTESIAN_POINT('Ctrl Pts',(60.5294814213625,249.694872277521,23.3066727109147)) ;
#110311=CARTESIAN_POINT('Ctrl Pts',(60.526367944473,249.704794021286,23.2415945367422)) ;
#110312=CARTESIAN_POINT('Ctrl Pts',(60.5232544675836,249.710864391968,23.1760559056965)) ;
#110313=CARTESIAN_POINT('Ctrl Pts',(60.5208215544255,249.715607862124,23.124843128634)) ;
#110314=CARTESIAN_POINT('Ctrl Pts',(60.5183886412675,249.718000590858,23.0733496192864)) ;
#110315=CARTESIAN_POINT('Ctrl Pts',(60.5159557281095,249.718015041886,23.0217905853416)) ;
#110316=CARTESIAN_POINT('Ctrl Pts',(60.7756980793889,247.272018954284,24.5128440309776)) ;
#110317=CARTESIAN_POINT('Ctrl Pts',(60.7756882950196,247.27221172625,24.512943322945)) ;
#110318=CARTESIAN_POINT('Ctrl Pts',(60.7756785124232,247.272404517696,24.5130425776592)) ;
#110319=CARTESIAN_POINT('Ctrl Pts',(60.7708844068105,247.36691143135,24.5616743441787)) ;
#110320=CARTESIAN_POINT('Ctrl Pts',(60.7665244328513,247.465624464848,24.601158305853)) ;
#110321=CARTESIAN_POINT('Ctrl Pts',(60.758085179004,247.659911268451,24.6582291111127)) ;
#110322=CARTESIAN_POINT('Ctrl Pts',(60.75403018082,247.754575228724,24.6773755531183)) ;
#110323=CARTESIAN_POINT('Ctrl Pts',(60.7484518396211,247.878663337132,24.6915124855888)) ;
#110324=CARTESIAN_POINT('Ctrl Pts',(60.7471593590571,247.907049901099,24.6940159297791)) ;
#110325=CARTESIAN_POINT('Ctrl Pts',(60.7449585594767,247.954650642069,24.6969945255557)) ;
#110326=CARTESIAN_POINT('Ctrl Pts',(60.7440625699028,247.973834394399,24.6978646242705)) ;
#110327=CARTESIAN_POINT('Ctrl Pts',(60.7422396821312,248.012442664656,24.6989520631554)) ;
#110328=CARTESIAN_POINT('Ctrl Pts',(60.7413126878787,248.031864424137,24.6991617141892)) ;
#110329=CARTESIAN_POINT('Ctrl Pts',(60.7389405694075,248.081009530957,24.6988389103594)) ;
#110330=CARTESIAN_POINT('Ctrl Pts',(60.737481838675,248.110722385268,24.697853756757)) ;
#110331=CARTESIAN_POINT('Ctrl Pts',(60.732081154403,248.218891572664,24.6913867519337)) ;
#110332=CARTESIAN_POINT('Ctrl Pts',(60.7280040725607,248.296956449574,24.6811807978971)) ;
#110333=CARTESIAN_POINT('Ctrl Pts',(60.7195223545697,248.454473878442,24.6492076559596)) ;
#110334=CARTESIAN_POINT('Ctrl Pts',(60.7151227743156,248.533628491368,24.6269911287199)) ;
#110335=CARTESIAN_POINT('Ctrl Pts',(60.7093542847243,248.63776696951,24.5893307269102)) ;
#110336=CARTESIAN_POINT('Ctrl Pts',(60.7078792233013,248.664442732654,24.5789041953016)) ;
#110337=CARTESIAN_POINT('Ctrl Pts',(60.7053441390305,248.710645677828,24.5594674962714)) ;
#110338=CARTESIAN_POINT('Ctrl Pts',(60.7042726836258,248.730290814842,24.5507553276267)) ;
#110339=CARTESIAN_POINT('Ctrl Pts',(60.7026417578212,248.760491106601,24.5366617922452)) ;
#110340=CARTESIAN_POINT('Ctrl Pts',(60.7020685170289,248.771165296168,24.5315422229156)) ;
#110341=CARTESIAN_POINT('Ctrl Pts',(60.7009860921404,248.791459879833,24.5215429307525)) ;
#110342=CARTESIAN_POINT('Ctrl Pts',(60.7004759211982,248.801088817705,24.5166827345866)) ;
#110343=CARTESIAN_POINT('Ctrl Pts',(60.6991765729357,248.825751476529,24.5039343993476)) ;
#110344=CARTESIAN_POINT('Ctrl Pts',(60.6983953249766,248.840713921812,24.4959101197923)) ;
#110345=CARTESIAN_POINT('Ctrl Pts',(60.694546708812,248.91486447455,24.4546822810237)) ;
#110346=CARTESIAN_POINT('Ctrl Pts',(60.6916476221793,248.972125779834,24.4181337118554)) ;
#110347=CARTESIAN_POINT('Ctrl Pts',(60.6848564495383,249.102774253487,24.3231241485434)) ;
#110348=CARTESIAN_POINT('Ctrl Pts',(60.6810107040293,249.173781445533,24.2617878033091)) ;
#110349=CARTESIAN_POINT('Ctrl Pts',(60.6753721079551,249.265790247043,24.1677790671748)) ;
#110350=CARTESIAN_POINT('Ctrl Pts',(60.6737241419899,249.291356368138,24.1398237805439)) ;
#110351=CARTESIAN_POINT('Ctrl Pts',(60.6706628629479,249.336101441456,24.087442050423)) ;
#110352=CARTESIAN_POINT('Ctrl Pts',(60.6692617156258,249.355590246044,24.0633025612448)) ;
#110353=CARTESIAN_POINT('Ctrl Pts',(60.6669299425261,249.386315352493,24.0230089552003)) ;
#110354=CARTESIAN_POINT('Ctrl Pts',(60.6660152281954,249.397956759727,24.0071726021503)) ;
#110355=CARTESIAN_POINT('Ctrl Pts',(60.6642057547193,249.420168449357,23.9758171969229)) ;
#110356=CARTESIAN_POINT('Ctrl Pts',(60.6633120699751,249.430761741512,23.960317975081)) ;
#110357=CARTESIAN_POINT('Ctrl Pts',(60.6611005586341,249.456049589632,23.9219523538644)) ;
#110358=CARTESIAN_POINT('Ctrl Pts',(60.6597722976602,249.470452514102,23.8989008779105)) ;
#110359=CARTESIAN_POINT('Ctrl Pts',(60.6517310427637,249.553007381473,23.7593404150994)) ;
#110360=CARTESIAN_POINT('Ctrl Pts',(60.6445299888298,249.607448218882,23.6353153559151)) ;
#110361=CARTESIAN_POINT('Ctrl Pts',(60.6347425156901,249.660680397238,23.4589592042698)) ;
#110362=CARTESIAN_POINT('Ctrl Pts',(60.6321398812924,249.672835583179,23.4111760884053)) ;
#110363=CARTESIAN_POINT('Ctrl Pts',(60.628473696915,249.687321102699,23.3415226424904)) ;
#110364=CARTESIAN_POINT('Ctrl Pts',(60.6273600044258,249.691353604983,23.3200339255529)) ;
#110365=CARTESIAN_POINT('Ctrl Pts',(60.625380552339,249.697874976116,23.2810988537752)) ;
#110366=CARTESIAN_POINT('Ctrl Pts',(60.624508782199,249.700511158593,23.2636804990575)) ;
#110367=CARTESIAN_POINT('Ctrl Pts',(60.6231160373809,249.704345382404,23.2353357829859)) ;
#110368=CARTESIAN_POINT('Ctrl Pts',(60.6225865440398,249.705711213931,23.2244337413542)) ;
#110369=CARTESIAN_POINT('Ctrl Pts',(60.621518287902,249.708280171311,23.2021562694147)) ;
#110370=CARTESIAN_POINT('Ctrl Pts',(60.6209800218559,249.709474253776,23.1907804409843)) ;
#110371=CARTESIAN_POINT('Ctrl Pts',(60.6195120421287,249.712445946117,23.1593798266152)) ;
#110372=CARTESIAN_POINT('Ctrl Pts',(60.6185947790194,249.713980179265,23.1393334662328)) ;
#110373=CARTESIAN_POINT('Ctrl Pts',(60.613676389243,249.720375347754,23.0299722824248)) ;
#110374=CARTESIAN_POINT('Ctrl Pts',(60.609953180776,249.718448519362,22.9403987509123)) ;
#110375=CARTESIAN_POINT('Ctrl Pts',(60.6016168885664,249.698182982402,22.7413304997973)) ;
#110376=CARTESIAN_POINT('Ctrl Pts',(60.5970090634153,249.676117704702,22.6326427516485)) ;
#110377=CARTESIAN_POINT('Ctrl Pts',(60.5908208374004,249.635348857434,22.5004351797759)) ;
#110378=CARTESIAN_POINT('Ctrl Pts',(60.589561966257,249.626525091478,22.4741524664437)) ;
#110379=CARTESIAN_POINT('Ctrl Pts',(60.587408304133,249.610591504135,22.4303229589549)) ;
#110380=CARTESIAN_POINT('Ctrl Pts',(60.5865250345099,249.603828431932,22.4126557428071)) ;
#110381=CARTESIAN_POINT('Ctrl Pts',(60.5848272278056,249.59041021247,22.3793036862277)) ;
#110382=CARTESIAN_POINT('Ctrl Pts',(60.5840146965054,249.583812027777,22.3635984316594)) ;
#110383=CARTESIAN_POINT('Ctrl Pts',(60.5818568407713,249.565836837352,22.3225740722141)) ;
#110384=CARTESIAN_POINT('Ctrl Pts',(60.5804983637245,249.554068978814,22.2974327967767)) ;
#110385=CARTESIAN_POINT('Ctrl Pts',(60.5723757747726,249.481108827343,22.1511257064931)) ;
#110386=CARTESIAN_POINT('Ctrl Pts',(60.5651155371879,249.406023608246,22.0374693238109)) ;
#110387=CARTESIAN_POINT('Ctrl Pts',(60.5553237484603,249.286704425232,21.8972296846088)) ;
#110388=CARTESIAN_POINT('Ctrl Pts',(60.552764878943,249.253735585327,21.8617167236432)) ;
#110389=CARTESIAN_POINT('Ctrl Pts',(60.5491552082394,249.203911859243,21.8125037247045)) ;
#110390=CARTESIAN_POINT('Ctrl Pts',(60.5480549537141,249.18825634191,21.7976261119993)) ;
#110391=CARTESIAN_POINT('Ctrl Pts',(60.5460983017611,249.159458036674,21.7712980128618)) ;
#110392=CARTESIAN_POINT('Ctrl Pts',(60.5452359778907,249.146415803772,21.7597422364009)) ;
#110393=CARTESIAN_POINT('Ctrl Pts',(60.5438575751423,249.124938523242,21.7413019527496)) ;
#110394=CARTESIAN_POINT('Ctrl Pts',(60.5433330862607,249.116612465502,21.7342928050292)) ;
#110395=CARTESIAN_POINT('Ctrl Pts',(60.5422686903961,249.099380095688,21.7200702400599)) ;
#110396=CARTESIAN_POINT('Ctrl Pts',(60.5417293674013,249.090467056009,21.7128661904103)) ;
#110397=CARTESIAN_POINT('Ctrl Pts',(60.5402600063694,249.065712958405,21.6932743629481)) ;
#110398=CARTESIAN_POINT('Ctrl Pts',(60.5393423679675,249.049721558261,21.6810788891601)) ;
#110399=CARTESIAN_POINT('Ctrl Pts',(60.5344257611681,248.961479629719,21.6162588514937)) ;
#110400=CARTESIAN_POINT('Ctrl Pts',(60.530703392912,248.88532566335,21.5691808088167)) ;
#110401=CARTESIAN_POINT('Ctrl Pts',(60.52235692247,248.707133430032,21.4778110470787)) ;
#110402=CARTESIAN_POINT('Ctrl Pts',(60.5177380727145,248.603721629302,21.4371331550186)) ;
#110403=CARTESIAN_POINT('Ctrl Pts',(60.5115372780093,248.47037171682,21.39940088093)) ;
#110404=CARTESIAN_POINT('Ctrl Pts',(60.5102772963219,248.443499761471,21.3925121436769)) ;
#110405=CARTESIAN_POINT('Ctrl Pts',(60.5081189006906,248.397961592575,21.3820342206756)) ;
#110406=CARTESIAN_POINT('Ctrl Pts',(60.5072319080356,248.37938247349,21.378090248574)) ;
#110407=CARTESIAN_POINT('Ctrl Pts',(60.5055247244688,248.343906610515,21.3711867055994)) ;
#110408=CARTESIAN_POINT('Ctrl Pts',(60.5047065016694,248.327023548782,21.3681691843591)) ;
#110409=CARTESIAN_POINT('Ctrl Pts',(60.5025272218163,248.282388182096,21.3608957963608)) ;
#110410=CARTESIAN_POINT('Ctrl Pts',(60.50115271224,248.25457095609,21.3570769278201)) ;
#110411=CARTESIAN_POINT('Ctrl Pts',(60.4933914856086,248.099375177315,21.3397264348219)) ;
#110412=CARTESIAN_POINT('Ctrl Pts',(60.4865739325228,247.970881768513,21.3401215126213)) ;
#110413=CARTESIAN_POINT('Ctrl Pts',(60.4758300255216,247.770272905264,21.3637869690811)) ;
#110414=CARTESIAN_POINT('Ctrl Pts',(60.4719222587402,247.697486713986,21.3772956834323)) ;
#110415=CARTESIAN_POINT('Ctrl Pts',(60.467275531377,247.607914624016,21.4001294947751)) ;
#110416=CARTESIAN_POINT('Ctrl Pts',(60.4663587592489,247.590079746232,21.4049912001505)) ;
#110417=CARTESIAN_POINT('Ctrl Pts',(60.4649141409273,247.561632340025,21.4132532467426)) ;
#110418=CARTESIAN_POINT('Ctrl Pts',(60.4643765755097,247.550967348624,21.4164661970968)) ;
#110419=CARTESIAN_POINT('Ctrl Pts',(60.463308548036,247.529594499147,21.4231378798415)) ;
#110420=CARTESIAN_POINT('Ctrl Pts',(60.4627782256082,247.518887881234,21.4265985940511)) ;
#110421=CARTESIAN_POINT('Ctrl Pts',(60.4613649441349,247.490138613034,21.436211748705)) ;
#110422=CARTESIAN_POINT('Ctrl Pts',(60.4604928148477,247.472164280201,21.4425645297025)) ;
#110423=CARTESIAN_POINT('Ctrl Pts',(60.4550548068125,247.35904409104,21.4847274998758)) ;
#110424=CARTESIAN_POINT('Ctrl Pts',(60.4508590982514,247.267202078817,21.5288201309582)) ;
#110425=CARTESIAN_POINT('Ctrl Pts',(60.4424256144262,247.093567330351,21.6325353855568)) ;
#110426=CARTESIAN_POINT('Ctrl Pts',(60.4382010448268,247.012039817882,21.6917673475751)) ;
#110427=CARTESIAN_POINT('Ctrl Pts',(60.4324634142796,246.915504421682,21.7761207598601)) ;
#110428=CARTESIAN_POINT('Ctrl Pts',(60.4312079239434,246.895149846064,21.7948132941593)) ;
#110429=CARTESIAN_POINT('Ctrl Pts',(60.4290551255958,246.861616999917,21.8271706465075)) ;
#110430=CARTESIAN_POINT('Ctrl Pts',(60.4281691054647,246.848191937335,21.8405721136499)) ;
#110431=CARTESIAN_POINT('Ctrl Pts',(60.4263542050348,246.821467995756,21.8681694834337)) ;
#110432=CARTESIAN_POINT('Ctrl Pts',(60.4254249473787,246.808183032421,21.8823747666608)) ;
#110433=CARTESIAN_POINT('Ctrl Pts',(60.4230220527906,246.774854356027,21.9192779390892)) ;
#110434=CARTESIAN_POINT('Ctrl Pts',(60.4215338158998,246.755173265535,21.9422927057729)) ;
#110435=CARTESIAN_POINT('Ctrl Pts',(60.4147117881363,246.669233207805,22.0484778426541)) ;
#110436=CARTESIAN_POINT('Ctrl Pts',(60.4091032168068,246.610355916954,22.1372921443611)) ;
#110437=CARTESIAN_POINT('Ctrl Pts',(60.3984874373699,246.516465566557,22.3131295558868)) ;
#110438=CARTESIAN_POINT('Ctrl Pts',(60.3935174048435,246.47954616916,22.398698708304)) ;
#110439=CARTESIAN_POINT('Ctrl Pts',(60.3879624601977,246.444273578533,22.5036629687607)) ;
#110440=CARTESIAN_POINT('Ctrl Pts',(60.3870864591605,246.438902991245,22.5205234427913)) ;
#110441=CARTESIAN_POINT('Ctrl Pts',(60.3856903291533,246.430636301643,22.5479700439543)) ;
#110442=CARTESIAN_POINT('Ctrl Pts',(60.3851615107751,246.427575638185,22.558504945522)) ;
#110443=CARTESIAN_POINT('Ctrl Pts',(60.3840945940326,246.421539827396,22.5800676212644)) ;
#110444=CARTESIAN_POINT('Ctrl Pts',(60.3835569672277,246.418573548026,22.5910971495276)) ;
#110445=CARTESIAN_POINT('Ctrl Pts',(60.3820976712151,246.410742634974,22.6214472569034)) ;
#110446=CARTESIAN_POINT('Ctrl Pts',(60.3811881224416,246.406109033969,22.6408259805346)) ;
#110447=CARTESIAN_POINT('Ctrl Pts',(60.3761759654763,246.382102346082,22.7497721627554)) ;
#110448=CARTESIAN_POINT('Ctrl Pts',(60.372366129365,246.369746197939,22.8407338175472)) ;
#110449=CARTESIAN_POINT('Ctrl Pts',(60.3640447714708,246.35914671648,23.0401185575803)) ;
#110450=CARTESIAN_POINT('Ctrl Pts',(60.3595378802725,246.363842773623,23.1482794770371)) ;
#110451=CARTESIAN_POINT('Ctrl Pts',(60.3534536156352,246.382818964015,23.2830589160743)) ;
#110452=CARTESIAN_POINT('Ctrl Pts',(60.352178063071,246.387435369662,23.3107828668696)) ;
#110453=CARTESIAN_POINT('Ctrl Pts',(60.3500018828507,246.396343500692,23.3570721362936)) ;
#110454=CARTESIAN_POINT('Ctrl Pts',(60.3491131952654,246.400259152053,23.3757042404542)) ;
#110455=CARTESIAN_POINT('Ctrl Pts',(60.3473022120707,246.408785382454,23.4131011524053)) ;
#110456=CARTESIAN_POINT('Ctrl Pts',(60.3463797517914,246.413404740268,23.4318609661218)) ;
#110457=CARTESIAN_POINT('Ctrl Pts',(60.3440152204185,246.425931961412,23.4791987326212)) ;
#110458=CARTESIAN_POINT('Ctrl Pts',(60.3425594201409,246.434275134729,23.5076537640707)) ;
#110459=CARTESIAN_POINT('Ctrl Pts',(60.3353219573036,246.478778390795,23.6457685170047)) ;
#110460=CARTESIAN_POINT('Ctrl Pts',(60.3292055530495,246.525435192964,23.7517040998283)) ;
#110461=CARTESIAN_POINT('Ctrl Pts',(60.3185222353801,246.62474042496,23.9259656762753)) ;
#110462=CARTESIAN_POINT('Ctrl Pts',(60.3139947988517,246.672464682292,23.9966239774957)) ;
#110463=CARTESIAN_POINT('Ctrl Pts',(60.3088339231225,246.736353482213,24.0772433758745)) ;
#110464=CARTESIAN_POINT('Ctrl Pts',(60.3079566381448,246.74757744604,24.0909546884778)) ;
#110465=CARTESIAN_POINT('Ctrl Pts',(60.3065592499092,246.766098866837,24.1128631887207)) ;
#110466=CARTESIAN_POINT('Ctrl Pts',(60.306030414377,246.77326309095,24.121170924443)) ;
#110467=CARTESIAN_POINT('Ctrl Pts',(60.3049637958043,246.788046791023,24.1379781333443)) ;
#110468=CARTESIAN_POINT('Ctrl Pts',(60.3044264739577,246.79567246014,24.1464712165966)) ;
#110469=CARTESIAN_POINT('Ctrl Pts',(60.3029695896086,246.81681335625,24.1695389282979)) ;
#110470=CARTESIAN_POINT('Ctrl Pts',(60.3020620702347,246.830502139319,24.1839525835433)) ;
#110471=CARTESIAN_POINT('Ctrl Pts',(60.2959718241457,246.925568341256,24.2805553744733)) ;
#110472=CARTESIAN_POINT('Ctrl Pts',(60.2912598309266,247.015006414797,24.3543887465359)) ;
#110473=CARTESIAN_POINT('Ctrl Pts',(60.2838183154058,247.163121216806,24.4528687515382)) ;
#110474=CARTESIAN_POINT('Ctrl Pts',(60.281189755399,247.216765758693,24.4843845077685)) ;
#110475=CARTESIAN_POINT('Ctrl Pts',(60.2784744057375,247.272018982637,24.5128440455817)) ;
#110476=CARTESIAN_POINT('Origin',(61.8645744874958,248.040265107786,23.0213203435596)) ;
#110477=CARTESIAN_POINT('',(59.6804129742801,247.272018954245,24.5128440309576)) ;
#110478=CARTESIAN_POINT('',(59.7780545670443,247.272019328904,24.5128442239351)) ;
#110479=CARTESIAN_POINT('',(61.8645744874958,247.272018954284,24.5128440309778)) ;
#110480=CARTESIAN_POINT('Ctrl Pts',(59.6804129742801,247.272018954245,24.5128440309576)) ;
#110481=CARTESIAN_POINT('Ctrl Pts',(59.6806620543328,247.267515292292,24.5105243085142)) ;
#110482=CARTESIAN_POINT('Ctrl Pts',(59.680910035148,247.263022056024,24.5081841461442)) ;
#110483=CARTESIAN_POINT('Ctrl Pts',(59.6816927490163,247.248806677377,24.5006984589357)) ;
#110484=CARTESIAN_POINT('Ctrl Pts',(59.6822231433743,247.239124257337,24.4954775302037)) ;
#110485=CARTESIAN_POINT('Ctrl Pts',(59.6832900874761,247.219525017563,24.4846591336161)) ;
#110486=CARTESIAN_POINT('Ctrl Pts',(59.6838262319107,247.209612530942,24.4790552371634)) ;
#110487=CARTESIAN_POINT('Ctrl Pts',(59.6852756879414,247.182676206818,24.4634631512753)) ;
#110488=CARTESIAN_POINT('Ctrl Pts',(59.6861771656862,247.165769965694,24.4532745694072)) ;
#110489=CARTESIAN_POINT('Ctrl Pts',(59.6912317207679,247.070505234997,24.3935464652148)) ;
#110490=CARTESIAN_POINT('Ctrl Pts',(59.6950835451313,246.996173230672,24.3378740844751)) ;
#110491=CARTESIAN_POINT('Ctrl Pts',(59.7034050316022,246.846817675636,24.2053666354242)) ;
#110492=CARTESIAN_POINT('Ctrl Pts',(59.7078698496296,246.773790947453,24.1269078185332)) ;
#110493=CARTESIAN_POINT('Ctrl Pts',(59.7139114988955,246.691535368857,24.0196049521105)) ;
#110494=CARTESIAN_POINT('Ctrl Pts',(59.7151941431971,246.674908651948,23.9967411301763)) ;
#110495=CARTESIAN_POINT('Ctrl Pts',(59.7173792147044,246.648042166898,23.9577626691775)) ;
#110496=CARTESIAN_POINT('Ctrl Pts',(59.7182694917991,246.637485331802,23.9418733354475)) ;
#110497=CARTESIAN_POINT('Ctrl Pts',(59.7200810816836,246.616796745235,23.9095519603271)) ;
#110498=CARTESIAN_POINT('Ctrl Pts',(59.7210024991347,246.606673098588,23.8931181970382)) ;
#110499=CARTESIAN_POINT('Ctrl Pts',(59.7233587767216,246.58179563045,23.8511290155879)) ;
#110500=CARTESIAN_POINT('Ctrl Pts',(59.7248071498076,246.56742869951,23.8253529472319)) ;
#110501=CARTESIAN_POINT('Ctrl Pts',(59.7321061886695,246.499554335427,23.6956481816735)) ;
#110502=CARTESIAN_POINT('Ctrl Pts',(59.7383015402635,246.456336543008,23.586715429275)) ;
#110503=CARTESIAN_POINT('Ctrl Pts',(59.7488672525254,246.402785392522,23.3956896665759)) ;
#110504=CARTESIAN_POINT('Ctrl Pts',(59.7531996129895,246.386528265154,23.3156811934708)) ;
#110505=CARTESIAN_POINT('Ctrl Pts',(59.7582610935112,246.373735831642,23.2159636805495)) ;
#110506=CARTESIAN_POINT('Ctrl Pts',(59.7592044377581,246.371638914121,23.1970830737012)) ;
#110507=CARTESIAN_POINT('Ctrl Pts',(59.7606799968342,246.368812790461,23.1669857456145)) ;
#110508=CARTESIAN_POINT('Ctrl Pts',(59.7612226563386,246.367874902904,23.1557906900765)) ;
#110509=CARTESIAN_POINT('Ctrl Pts',(59.7622903191718,246.366231754429,23.1334866319748)) ;
#110510=CARTESIAN_POINT('Ctrl Pts',(59.7628153918554,246.36552446292,23.1223783844853)) ;
#110511=CARTESIAN_POINT('Ctrl Pts',(59.7641978007073,246.363936367739,23.0927975921678)) ;
#110512=CARTESIAN_POINT('Ctrl Pts',(59.7650451074473,246.363250325296,23.0743157150745)) ;
#110513=CARTESIAN_POINT('Ctrl Pts',(59.7706993737046,246.360673216758,22.9490355425851)) ;
#110514=CARTESIAN_POINT('Ctrl Pts',(59.7750907626066,246.368679309752,22.8422695042726)) ;
#110515=CARTESIAN_POINT('Ctrl Pts',(59.7834881657177,246.402793732002,22.6438876448596)) ;
#110516=CARTESIAN_POINT('Ctrl Pts',(59.7874663023605,246.426635285591,22.5523160474912)) ;
#110517=CARTESIAN_POINT('Ctrl Pts',(59.7929599491064,246.467559136449,22.4362924270615)) ;
#110518=CARTESIAN_POINT('Ctrl Pts',(59.7942559158159,246.47775166217,22.4095905351453)) ;
#110519=CARTESIAN_POINT('Ctrl Pts',(59.7964569872288,246.495897738814,22.3654693671202)) ;
#110520=CARTESIAN_POINT('Ctrl Pts',(59.7973495177739,246.503476576124,22.347902162373)) ;
#110521=CARTESIAN_POINT('Ctrl Pts',(59.799160178796,246.519276040873,22.3129366505932)) ;
#110522=CARTESIAN_POINT('Ctrl Pts',(59.8000782882456,246.527498858853,22.2955425286946)) ;
#110523=CARTESIAN_POINT('Ctrl Pts',(59.80241436431,246.548936896717,22.2521415193206)) ;
#110524=CARTESIAN_POINT('Ctrl Pts',(59.8038453742908,246.562534298642,22.2263313991135)) ;
#110525=CARTESIAN_POINT('Ctrl Pts',(59.8112745460522,246.63544887219,22.0962678079333)) ;
#110526=CARTESIAN_POINT('Ctrl Pts',(59.8176397208265,246.705144028713,21.9982486888786)) ;
#110527=CARTESIAN_POINT('Ctrl Pts',(59.8283536907305,246.838600459491,21.8476695345017)) ;
#110528=CARTESIAN_POINT('Ctrl Pts',(59.8326672965295,246.89687679133,21.7908248963279)) ;
#110529=CARTESIAN_POINT('Ctrl Pts',(59.8376454559327,246.972716823504,21.7269072492334)) ;
#110530=CARTESIAN_POINT('Ctrl Pts',(59.8385308772057,246.986569126506,21.7156062005181)) ;
#110531=CARTESIAN_POINT('Ctrl Pts',(59.8399380576791,247.00923746462,21.6977085506039)) ;
#110532=CARTESIAN_POINT('Ctrl Pts',(59.8404687494576,247.017942251053,21.6909737068636)) ;
#110533=CARTESIAN_POINT('Ctrl Pts',(59.8415356650139,247.035780964374,21.6774505018725)) ;
#110534=CARTESIAN_POINT('Ctrl Pts',(59.8420714963053,247.044918856245,21.6706685014664)) ;
#110535=CARTESIAN_POINT('Ctrl Pts',(59.843519053562,247.070064244445,21.6523997850894)) ;
#110536=CARTESIAN_POINT('Ctrl Pts',(59.8444189982827,247.086206548856,21.6411009646054)) ;
#110537=CARTESIAN_POINT('Ctrl Pts',(59.8494824127726,247.179598553874,21.5781527210778)) ;
#110538=CARTESIAN_POINT('Ctrl Pts',(59.8533428632908,247.260840683327,21.5327034850549)) ;
#110539=CARTESIAN_POINT('Ctrl Pts',(59.8602595992641,247.411897658155,21.4639728176958)) ;
#110540=CARTESIAN_POINT('Ctrl Pts',(59.8633028648079,247.480262978178,21.4381039762889)) ;
#110541=CARTESIAN_POINT('Ctrl Pts',(59.8679047265794,247.582156804546,21.4069765648762)) ;
#110542=CARTESIAN_POINT('Ctrl Pts',(59.8693743103539,247.614505270356,21.3981452235329)) ;
#110543=CARTESIAN_POINT('Ctrl Pts',(59.8721388166287,247.674660573343,21.3836444393334)) ;
#110544=CARTESIAN_POINT('Ctrl Pts',(59.8734252273868,247.702388555088,21.3776998364978)) ;
#110545=CARTESIAN_POINT('Ctrl Pts',(59.8756148182735,247.749015659346,21.3689331905283)) ;
#110546=CARTESIAN_POINT('Ctrl Pts',(59.8765057288458,247.767836680698,21.3657261115105)) ;
#110547=CARTESIAN_POINT('Ctrl Pts',(59.8783170323988,247.805769324692,21.3599267655374)) ;
#110548=CARTESIAN_POINT('Ctrl Pts',(59.8792374941412,247.824879061656,21.3573414655143)) ;
#110549=CARTESIAN_POINT('Ctrl Pts',(59.8815879433654,247.873235390856,21.3516464227134)) ;
#110550=CARTESIAN_POINT('Ctrl Pts',(59.883031307828,247.902526281754,21.3489753402142)) ;
#110551=CARTESIAN_POINT('Ctrl Pts',(59.8903697848691,248.049430745504,21.3394644534301)) ;
#110552=CARTESIAN_POINT('Ctrl Pts',(59.8966161979755,248.167451889076,21.3442573763587)) ;
#110553=CARTESIAN_POINT('Ctrl Pts',(59.9072597423143,248.36519220519,21.3732897104311)) ;
#110554=CARTESIAN_POINT('Ctrl Pts',(59.9116194942626,248.445424895147,21.3911578188894)) ;
#110555=CARTESIAN_POINT('Ctrl Pts',(59.9166655293252,248.541570827575,21.4201104334586)) ;
#110556=CARTESIAN_POINT('Ctrl Pts',(59.917573824157,248.559023520705,21.4256792938913)) ;
#110557=CARTESIAN_POINT('Ctrl Pts',(59.9190079718349,248.586894857967,21.4350782232109)) ;
#110558=CARTESIAN_POINT('Ctrl Pts',(59.919543347158,248.597372494598,21.4387276849206)) ;
#110559=CARTESIAN_POINT('Ctrl Pts',(59.9206101519694,248.618421714908,21.4462942877779)) ;
#110560=CARTESIAN_POINT('Ctrl Pts',(59.9211413817521,248.628991512373,21.4502145634733)) ;
#110561=CARTESIAN_POINT('Ctrl Pts',(59.9225610680006,248.657440004371,21.4610933589955)) ;
#110562=CARTESIAN_POINT('Ctrl Pts',(59.9234385048945,248.675240560305,21.4682526295292)) ;
#110563=CARTESIAN_POINT('Ctrl Pts',(59.9288204001479,248.785351529421,21.5147483001097)) ;
#110564=CARTESIAN_POINT('Ctrl Pts',(59.9329652812003,248.874108544832,21.5619979734944)) ;
#110565=CARTESIAN_POINT('Ctrl Pts',(59.9414086583789,249.043646344936,21.6727985130441)) ;
#110566=CARTESIAN_POINT('Ctrl Pts',(59.9456967805549,249.123887365524,21.7363900494957)) ;
#110567=CARTESIAN_POINT('Ctrl Pts',(59.9514991253078,249.217684543246,21.8257953187344)) ;
#110568=CARTESIAN_POINT('Ctrl Pts',(59.9527452136855,249.237061175161,21.8451929321733)) ;
#110569=CARTESIAN_POINT('Ctrl Pts',(59.9548866111785,249.268997066268,21.8787701020926)) ;
#110570=CARTESIAN_POINT('Ctrl Pts',(59.9557709119488,249.281807506611,21.8927036162442)) ;
#110571=CARTESIAN_POINT('Ctrl Pts',(59.9574774542275,249.305796584708,21.9196985519908)) ;
#110572=CARTESIAN_POINT('Ctrl Pts',(59.9582978318402,249.317015595051,21.9327209419725)) ;
#110573=CARTESIAN_POINT('Ctrl Pts',(59.9604938797889,249.346213569501,21.9676846215701)) ;
#110574=CARTESIAN_POINT('Ctrl Pts',(59.9618834253937,249.363839048349,21.989912799075)) ;
#110575=CARTESIAN_POINT('Ctrl Pts',(59.9695760071074,249.456831727206,22.1135006251323)) ;
#110576=CARTESIAN_POINT('Ctrl Pts',(59.9762956255979,249.521123262515,22.2226661050005)) ;
#110577=CARTESIAN_POINT('Ctrl Pts',(59.9858480768859,249.594229813972,22.3865987221059)) ;
#110578=CARTESIAN_POINT('Ctrl Pts',(59.9886687109269,249.613582853527,22.4362139139115)) ;
#110579=CARTESIAN_POINT('Ctrl Pts',(59.9925977756553,249.637820047479,22.5083053032928)) ;
#110580=CARTESIAN_POINT('Ctrl Pts',(59.9937635155822,249.644652836141,22.5300909582373)) ;
#110581=CARTESIAN_POINT('Ctrl Pts',(59.9958233867228,249.65612311291,22.5694594152369)) ;
#110582=CARTESIAN_POINT('Ctrl Pts',(59.9967242944594,249.660923431469,22.586990932214)) ;
#110583=CARTESIAN_POINT('Ctrl Pts',(59.9981497256906,249.66818654112,22.6153162635981)) ;
#110584=CARTESIAN_POINT('Ctrl Pts',(59.998683580311,249.670828974291,22.6260622006264)) ;
#110585=CARTESIAN_POINT('Ctrl Pts',(59.9997503535679,249.675955915187,22.6478387954203)) ;
#110586=CARTESIAN_POINT('Ctrl Pts',(60.0002830116965,249.678435609763,22.65886992806)) ;
#110587=CARTESIAN_POINT('Ctrl Pts',(60.0017113515012,249.684855324651,22.6888413174326)) ;
#110588=CARTESIAN_POINT('Ctrl Pts',(60.002595779097,249.688579672782,22.7078264304126)) ;
#110589=CARTESIAN_POINT('Ctrl Pts',(60.0078865104848,249.70921120396,22.8235592857794)) ;
#110590=CARTESIAN_POINT('Ctrl Pts',(60.011950079609,249.717925993855,22.9215816218335)) ;
#110591=CARTESIAN_POINT('Ctrl Pts',(60.0201232737497,249.718102523529,23.1176623295655)) ;
#110592=CARTESIAN_POINT('Ctrl Pts',(60.0242214056265,249.709629801772,23.2153307942135)) ;
#110593=CARTESIAN_POINT('Ctrl Pts',(60.0299224414467,249.6874451356,23.3415752665169)) ;
#110594=CARTESIAN_POINT('Ctrl Pts',(60.031293642495,249.681385808762,23.3713031658761)) ;
#110595=CARTESIAN_POINT('Ctrl Pts',(60.0335856870227,249.670123200892,23.4198001473)) ;
#110596=CARTESIAN_POINT('Ctrl Pts',(60.0344914771101,249.665393061834,23.4386722970718)) ;
#110597=CARTESIAN_POINT('Ctrl Pts',(60.0363006411081,249.655408946824,23.4757591950049)) ;
#110598=CARTESIAN_POINT('Ctrl Pts',(60.0372033423329,249.650172324099,23.4939756189885)) ;
#110599=CARTESIAN_POINT('Ctrl Pts',(60.0394437668875,249.636563545334,23.5384629348542)) ;
#110600=CARTESIAN_POINT('Ctrl Pts',(60.0407923706905,249.627850453181,23.5646230417524)) ;
#110601=CARTESIAN_POINT('Ctrl Pts',(60.0470888523167,249.584820661287,23.6839251770361)) ;
#110602=CARTESIAN_POINT('Ctrl Pts',(60.0522806503703,249.542928947074,23.7741112937021)) ;
#110603=CARTESIAN_POINT('Ctrl Pts',(60.0630593888772,249.441570125258,23.9497085752273)) ;
#110604=CARTESIAN_POINT('Ctrl Pts',(60.0686286752913,249.381632988268,24.0343823419641)) ;
#110605=CARTESIAN_POINT('Ctrl Pts',(60.074788335451,249.30199696185,24.127319291666)) ;
#110606=CARTESIAN_POINT('Ctrl Pts',(60.0757249585487,249.289480826448,24.1414368940227)) ;
#110607=CARTESIAN_POINT('Ctrl Pts',(60.077192575774,249.26915386275,24.1636001186608)) ;
#110608=CARTESIAN_POINT('Ctrl Pts',(60.0777338352236,249.261496174889,24.1717834461276)) ;
#110609=CARTESIAN_POINT('Ctrl Pts',(60.0788012445498,249.246053312973,24.1879583834992)) ;
#110610=CARTESIAN_POINT('Ctrl Pts',(60.0793274150755,249.238269289188,24.1959502874408)) ;
#110611=CARTESIAN_POINT('Ctrl Pts',(60.0807165071776,249.217284130595,24.2170702614548)) ;
#110612=CARTESIAN_POINT('Ctrl Pts',(60.0815692233575,249.203942941329,24.2300575338184)) ;
#110613=CARTESIAN_POINT('Ctrl Pts',(60.0834725975997,249.17322038371,24.2589848434578)) ;
#110614=CARTESIAN_POINT('Ctrl Pts',(60.084515233874,249.155713414926,24.27478602767)) ;
#110615=CARTESIAN_POINT('Ctrl Pts',(60.0879981563692,249.095260791897,24.3270785467251)) ;
#110616=CARTESIAN_POINT('Ctrl Pts',(60.0903658832081,249.050810893612,24.3617747895713)) ;
#110617=CARTESIAN_POINT('Ctrl Pts',(60.0977238833365,248.90663352903,24.4630600238041)) ;
#110618=CARTESIAN_POINT('Ctrl Pts',(60.102669048862,248.801471193271,24.5212440829292)) ;
#110619=CARTESIAN_POINT('Ctrl Pts',(60.1093138582763,248.66412148195,24.5790429401345)) ;
#110620=CARTESIAN_POINT('Ctrl Pts',(60.1106355864062,248.636937357643,24.5896565875319)) ;
#110621=CARTESIAN_POINT('Ctrl Pts',(60.1128677037412,248.591391687656,24.6060836574672)) ;
#110622=CARTESIAN_POINT('Ctrl Pts',(60.1137646863813,248.573181731164,24.6122996345218)) ;
#110623=CARTESIAN_POINT('Ctrl Pts',(60.1155741787527,248.536661596145,24.6240684642749)) ;
#110624=CARTESIAN_POINT('Ctrl Pts',(60.1164864340269,248.518355336366,24.6296240177572)) ;
#110625=CARTESIAN_POINT('Ctrl Pts',(60.1187865147663,248.472483387148,24.6426927794214)) ;
#110626=CARTESIAN_POINT('Ctrl Pts',(60.1201865581757,248.444813936547,24.6498169935464)) ;
#110627=CARTESIAN_POINT('Ctrl Pts',(60.12628226775,248.325437690679,24.6773233640216)) ;
#110628=CARTESIAN_POINT('Ctrl Pts',(60.1311899878649,248.232298598277,24.6906881914895)) ;
#110629=CARTESIAN_POINT('Ctrl Pts',(60.1418908589937,248.031209442134,24.7024874134421)) ;
#110630=CARTESIAN_POINT('Ctrl Pts',(60.1476860631058,247.923517444686,24.6984538113917)) ;
#110631=CARTESIAN_POINT('Ctrl Pts',(60.1540166341008,247.798699582628,24.681690849035)) ;
#110632=CARTESIAN_POINT('Ctrl Pts',(60.1549298848446,247.780490848836,24.6789395709323)) ;
#110633=CARTESIAN_POINT('Ctrl Pts',(60.1563698854962,247.751370037737,24.6740478533021)) ;
#110634=CARTESIAN_POINT('Ctrl Pts',(60.1569062866519,247.740427855667,24.6720978028562)) ;
#110635=CARTESIAN_POINT('Ctrl Pts',(60.1579731562519,247.718448733921,24.6679550571688)) ;
#110636=CARTESIAN_POINT('Ctrl Pts',(60.1585034649354,247.707412897652,24.6657597853227)) ;
#110637=CARTESIAN_POINT('Ctrl Pts',(60.1599175492146,247.677724596064,24.659543006165)) ;
#110638=CARTESIAN_POINT('Ctrl Pts',(60.1607904564246,247.659116875322,24.6553139764596)) ;
#110639=CARTESIAN_POINT('Ctrl Pts',(60.1655611620724,247.55624837165,24.6300817951632)) ;
#110640=CARTESIAN_POINT('Ctrl Pts',(60.1691912131327,247.473638034325,24.6028771224125)) ;
#110641=CARTESIAN_POINT('Ctrl Pts',(60.174677093633,247.352244883397,24.5521607359739)) ;
#110642=CARTESIAN_POINT('Ctrl Pts',(60.1765349147425,247.311719635658,24.5332928537005)) ;
#110643=CARTESIAN_POINT('Ctrl Pts',(60.178415027332,247.272018800728,24.5128439518851)) ;
#110644=CARTESIAN_POINT('Ctrl Pts',(60.2784744057375,247.272018982637,24.5128440455817)) ;
#110645=CARTESIAN_POINT('Ctrl Pts',(60.2776289566685,247.289222581645,24.5217051842002)) ;
#110646=CARTESIAN_POINT('Ctrl Pts',(60.2767753101108,247.306582142027,24.530270043404)) ;
#110647=CARTESIAN_POINT('Ctrl Pts',(60.2746056555497,247.350595837132,24.5510459570075)) ;
#110648=CARTESIAN_POINT('Ctrl Pts',(60.2732782937851,247.377423864104,24.5628603281162)) ;
#110649=CARTESIAN_POINT('Ctrl Pts',(60.2710394110508,247.422374309508,24.5812649347257)) ;
#110650=CARTESIAN_POINT('Ctrl Pts',(60.2701414805683,247.440325821343,24.5882565203609)) ;
#110651=CARTESIAN_POINT('Ctrl Pts',(60.2683322577767,247.476313648988,24.6015636353876)) ;
#110652=CARTESIAN_POINT('Ctrl Pts',(60.2674212700478,247.494345378787,24.6078832077013)) ;
#110653=CARTESIAN_POINT('Ctrl Pts',(60.2651288195875,247.539478463412,24.6228404752716)) ;
#110654=CARTESIAN_POINT('Ctrl Pts',(60.2637353116982,247.566698296678,24.6310993189415)) ;
#110655=CARTESIAN_POINT('Ctrl Pts',(60.2560685179331,247.715271468106,24.6720839146282)) ;
#110656=CARTESIAN_POINT('Ctrl Pts',(60.2493837110393,247.83978716468,24.6917818949342)) ;
#110657=CARTESIAN_POINT('Ctrl Pts',(60.2398496418138,248.018753539113,24.6997851073337)) ;
#110658=CARTESIAN_POINT('Ctrl Pts',(60.2370142102413,248.072280280384,24.6996177426996)) ;
#110659=CARTESIAN_POINT('Ctrl Pts',(60.2330673123463,248.148573954947,24.695727227887)) ;
#110660=CARTESIAN_POINT('Ctrl Pts',(60.2318980800607,248.171413337977,24.6940933221516)) ;
#110661=CARTESIAN_POINT('Ctrl Pts',(60.2298327726669,248.212349703012,24.6903211498672)) ;
#110662=CARTESIAN_POINT('Ctrl Pts',(60.2289298729534,248.23045877387,24.688354601587)) ;
#110663=CARTESIAN_POINT('Ctrl Pts',(60.2275020895802,248.259520507672,24.6847188976708)) ;
#110664=CARTESIAN_POINT('Ctrl Pts',(60.2269678250872,248.270494625683,24.6832355234875)) ;
#110665=CARTESIAN_POINT('Ctrl Pts',(60.225901099512,248.292632040687,24.6800197098943)) ;
#110666=CARTESIAN_POINT('Ctrl Pts',(60.2253688816639,248.303794072806,24.678282972677)) ;
#110667=CARTESIAN_POINT('Ctrl Pts',(60.2239430247819,248.333977014467,24.6732739887185)) ;
#110668=CARTESIAN_POINT('Ctrl Pts',(60.2230605731415,248.352960799856,24.6697859902233)) ;
#110669=CARTESIAN_POINT('Ctrl Pts',(60.2177403334771,248.468825812525,24.6464237890574)) ;
#110670=CARTESIAN_POINT('Ctrl Pts',(60.2136505668861,248.563861354591,24.6183412808526)) ;
#110671=CARTESIAN_POINT('Ctrl Pts',(60.2066222833348,248.720706019702,24.5564757553712)) ;
#110672=CARTESIAN_POINT('Ctrl Pts',(60.2037090470471,248.783878514843,24.5268901868337)) ;
#110673=CARTESIAN_POINT('Ctrl Pts',(60.1992785438693,248.87372764079,24.4777733020803)) ;
#110674=CARTESIAN_POINT('Ctrl Pts',(60.1978423994883,248.901963167498,24.4612478878456)) ;
#110675=CARTESIAN_POINT('Ctrl Pts',(60.1951337894306,248.953307455088,24.4291463667674)) ;
#110676=CARTESIAN_POINT('Ctrl Pts',(60.193869202453,248.976546106726,24.4137995100251)) ;
#110677=CARTESIAN_POINT('Ctrl Pts',(60.1917058411474,249.014980022186,24.3870204845665)) ;
#110678=CARTESIAN_POINT('Ctrl Pts',(60.1908186505491,249.030382630649,24.3758952935882)) ;
#110679=CARTESIAN_POINT('Ctrl Pts',(60.1890056858663,249.061114141341,24.3528939207677)) ;
#110680=CARTESIAN_POINT('Ctrl Pts',(60.1880796326852,249.076432696064,24.3410088034847)) ;
#110681=CARTESIAN_POINT('Ctrl Pts',(60.1856947277643,249.114909014026,24.3100734457593)) ;
#110682=CARTESIAN_POINT('Ctrl Pts',(60.1842216857803,249.137767696647,24.2906634844707)) ;
#110683=CARTESIAN_POINT('Ctrl Pts',(60.1771586567455,249.243146709639,24.1962078936101)) ;
#110684=CARTESIAN_POINT('Ctrl Pts',(60.1712608176561,249.31856072352,24.1136754353094)) ;
#110685=CARTESIAN_POINT('Ctrl Pts',(60.1606912426268,249.437187380823,23.9545993991115)) ;
#110686=CARTESIAN_POINT('Ctrl Pts',(60.1560600002136,249.483662343065,23.8809760304521)) ;
#110687=CARTESIAN_POINT('Ctrl Pts',(60.1507620607461,249.532830317509,23.7877630568401)) ;
#110688=CARTESIAN_POINT('Ctrl Pts',(60.1498470939627,249.541167262585,23.7713057501868)) ;
#110689=CARTESIAN_POINT('Ctrl Pts',(60.1484051218049,249.554092078485,23.7447127752868)) ;
#110690=CARTESIAN_POINT('Ctrl Pts',(60.1478684196099,249.558853369701,23.734663467821)) ;
#110691=CARTESIAN_POINT('Ctrl Pts',(60.1468017496556,249.56822610669,23.7143618984894)) ;
#110692=CARTESIAN_POINT('Ctrl Pts',(60.1462719256948,249.572835118125,23.7041091742211)) ;
#110693=CARTESIAN_POINT('Ctrl Pts',(60.1448603799075,249.58497045517,23.67637207197)) ;
#110694=CARTESIAN_POINT('Ctrl Pts',(60.1439894627165,249.592303011124,23.6588042852826)) ;
#110695=CARTESIAN_POINT('Ctrl Pts',(60.1385422714053,249.636973627156,23.546437012392)) ;
#110696=CARTESIAN_POINT('Ctrl Pts',(60.1343383950824,249.665912945952,23.4485187011399)) ;
#110697=CARTESIAN_POINT('Ctrl Pts',(60.1259017325359,249.705381695324,23.2500578618463)) ;
#110698=CARTESIAN_POINT('Ctrl Pts',(60.1216825504788,249.716086396669,23.149987297837)) ;
#110699=CARTESIAN_POINT('Ctrl Pts',(60.1159514715112,249.718242326937,23.0219504888093)) ;
#110700=CARTESIAN_POINT('Ctrl Pts',(60.1146965564959,249.718025295756,22.9943277999102)) ;
#110701=CARTESIAN_POINT('Ctrl Pts',(60.1125447908475,249.716509591761,22.9477748517733)) ;
#110702=CARTESIAN_POINT('Ctrl Pts',(60.1116592250982,249.715571501506,22.9288381203865)) ;
#110703=CARTESIAN_POINT('Ctrl Pts',(60.1098453366348,249.713022137616,22.8905274193764)) ;
#110704=CARTESIAN_POINT('Ctrl Pts',(60.1089166384687,249.71139464885,22.8711574720957)) ;
#110705=CARTESIAN_POINT('Ctrl Pts',(60.1065154503971,249.706374399746,22.8217200450597)) ;
#110706=CARTESIAN_POINT('Ctrl Pts',(60.1050283793628,249.702504234628,22.791708951012)) ;
#110707=CARTESIAN_POINT('Ctrl Pts',(60.0981901461491,249.681324375861,22.6564224785539)) ;
#110708=CARTESIAN_POINT('Ctrl Pts',(60.0925619274017,249.654810566574,22.5528504564865)) ;
#110709=CARTESIAN_POINT('Ctrl Pts',(60.0820908158341,249.588152766786,22.3678828921028)) ;
#110710=CARTESIAN_POINT('Ctrl Pts',(60.0772865967868,249.550897350326,22.2858417433541)) ;
#110711=CARTESIAN_POINT('Ctrl Pts',(60.0717923536121,249.497959749139,22.1904549648953)) ;
#110712=CARTESIAN_POINT('Ctrl Pts',(60.0708420889847,249.48839201615,22.1738892502953)) ;
#110713=CARTESIAN_POINT('Ctrl Pts',(60.0693584318031,249.472745405935,22.1478376371493)) ;
#110714=CARTESIAN_POINT('Ctrl Pts',(60.0688144069575,249.466850910674,22.138243448215)) ;
#110715=CARTESIAN_POINT('Ctrl Pts',(60.0678107402087,249.455667647009,22.1204452314797)) ;
#110716=CARTESIAN_POINT('Ctrl Pts',(60.067349557359,249.45040307088,22.1122267030499)) ;
#110717=CARTESIAN_POINT('Ctrl Pts',(60.0660992080836,249.43579650794,22.0898566062344)) ;
#110718=CARTESIAN_POINT('Ctrl Pts',(60.0653189963652,249.426311010344,22.0757996525973)) ;
#110719=CARTESIAN_POINT('Ctrl Pts',(60.0612969764142,249.375597332534,22.0030485779749)) ;
#110720=CARTESIAN_POINT('Ctrl Pts',(60.0582456609486,249.330846479603,21.94689450141)) ;
#110721=CARTESIAN_POINT('Ctrl Pts',(60.0514267454659,249.221551625529,21.826469589256)) ;
#110722=CARTESIAN_POINT('Ctrl Pts',(60.0476909914728,249.155099031945,21.7642398631361)) ;
#110723=CARTESIAN_POINT('Ctrl Pts',(60.0421934580009,249.054712872913,21.6844831048761)) ;
#110724=CARTESIAN_POINT('Ctrl Pts',(60.0405688634349,249.024724734728,21.6622481865668)) ;
#110725=CARTESIAN_POINT('Ctrl Pts',(60.0375473430975,248.968795796088,21.6236022207869)) ;
#110726=CARTESIAN_POINT('Ctrl Pts',(60.0361621733384,248.943098454237,21.6068674436997)) ;
#110727=CARTESIAN_POINT('Ctrl Pts',(60.0338532450256,248.900319818457,21.5806497499206)) ;
#110728=CARTESIAN_POINT('Ctrl Pts',(60.0329450185226,248.883505578718,21.5707441356093)) ;
#110729=CARTESIAN_POINT('Ctrl Pts',(60.0311460588964,248.850256867152,21.5519300925993)) ;
#110730=CARTESIAN_POINT('Ctrl Pts',(60.0302563369079,248.833838716279,21.542998574357)) ;
#110731=CARTESIAN_POINT('Ctrl Pts',(60.028050875092,248.793225056177,21.5217761721123)) ;
#110732=CARTESIAN_POINT('Ctrl Pts',(60.0267246242141,248.768874532681,21.5097947545086)) ;
#110733=CARTESIAN_POINT('Ctrl Pts',(60.0186859080469,248.621751214475,21.4417856139034)) ;
#110734=CARTESIAN_POINT('Ctrl Pts',(60.011482968448,248.492887076939,21.4001543102271)) ;
#110735=CARTESIAN_POINT('Ctrl Pts',(60.0016864712964,248.311981568598,21.364982871853)) ;
#110736=CARTESIAN_POINT('Ctrl Pts',(59.9990770962117,248.263112652409,21.3577028974612)) ;
#110737=CARTESIAN_POINT('Ctrl Pts',(59.9954044167687,248.192249671143,21.3503255455471)) ;
#110738=CARTESIAN_POINT('Ctrl Pts',(59.9942904565498,248.170464216292,21.3484870637654)) ;
#110739=CARTESIAN_POINT('Ctrl Pts',(59.9923115370205,248.131088056635,21.3459380260121)) ;
#110740=CARTESIAN_POINT('Ctrl Pts',(59.9914405149514,248.113510342178,21.3450775514954)) ;
#110741=CARTESIAN_POINT('Ctrl Pts',(59.9900503235385,248.08497855944,21.3441305347332)) ;
#110742=CARTESIAN_POINT('Ctrl Pts',(59.9895225884216,248.074031676831,21.3438744322677)) ;
#110743=CARTESIAN_POINT('Ctrl Pts',(59.9884554670857,248.051634479983,21.3435698007015)) ;
#110744=CARTESIAN_POINT('Ctrl Pts',(59.987916599857,248.040184750347,21.3435312764594)) ;
#110745=CARTESIAN_POINT('Ctrl Pts',(59.9864503158695,248.008685340553,21.343747752589)) ;
#110746=CARTESIAN_POINT('Ctrl Pts',(59.9855352060764,247.98863877069,21.3442449543637)) ;
#110747=CARTESIAN_POINT('Ctrl Pts',(59.9806245948603,247.879400427121,21.3489149940543)) ;
#110748=CARTESIAN_POINT('Ctrl Pts',(59.9769054622383,247.790634846768,21.3598437692565)) ;
#110749=CARTESIAN_POINT('Ctrl Pts',(59.9685631184884,247.594573335977,21.4000584915383)) ;
#110750=CARTESIAN_POINT('Ctrl Pts',(59.9639454051421,247.488469314128,21.4330349305119)) ;
#110751=CARTESIAN_POINT('Ctrl Pts',(59.9577439875736,247.36081060111,21.4870587354343)) ;
#110752=CARTESIAN_POINT('Ctrl Pts',(59.9564819733251,247.335495780502,21.4985212093475)) ;
#110753=CARTESIAN_POINT('Ctrl Pts',(59.9543217070367,247.293380042413,21.5188662431163)) ;
#110754=CARTESIAN_POINT('Ctrl Pts',(59.9534349594196,247.276423950401,21.5274153010682)) ;
#110755=CARTESIAN_POINT('Ctrl Pts',(59.951621788238,247.242444769981,21.5452769362036)) ;
#110756=CARTESIAN_POINT('Ctrl Pts',(59.9506950603393,247.225430866707,21.5546006863894)) ;
#110757=CARTESIAN_POINT('Ctrl Pts',(59.9483059547366,247.182481433473,21.5791152712235)) ;
#110758=CARTESIAN_POINT('Ctrl Pts',(59.9468292857573,247.156786139901,21.5947114016268)) ;
#110759=CARTESIAN_POINT('Ctrl Pts',(59.93981248876,247.038622908499,21.6708493221273)) ;
#110760=CARTESIAN_POINT('Ctrl Pts',(59.9339711610932,246.95187351876,21.7397364030671)) ;
#110761=CARTESIAN_POINT('Ctrl Pts',(59.9233954851838,246.8093054475,21.8779314600053)) ;
#110762=CARTESIAN_POINT('Ctrl Pts',(59.9187014689674,246.750994377659,21.9441097336536)) ;
#110763=CARTESIAN_POINT('Ctrl Pts',(59.9133556903777,246.687160626746,22.0292072201083)) ;
#110764=CARTESIAN_POINT('Ctrl Pts',(59.9124479787295,246.67641562535,22.0440308138027)) ;
#110765=CARTESIAN_POINT('Ctrl Pts',(59.9110145780852,246.659553728031,22.0681130442463)) ;
#110766=CARTESIAN_POINT('Ctrl Pts',(59.9104793807375,246.65328248386,22.0772614015037)) ;
#110767=CARTESIAN_POINT('Ctrl Pts',(59.9094127799267,246.640821253868,22.0958318092894)) ;
#110768=CARTESIAN_POINT('Ctrl Pts',(59.9088815791073,246.634634615109,22.1052553577)) ;
#110769=CARTESIAN_POINT('Ctrl Pts',(59.9074617601964,246.618175038949,22.1308861397013)) ;
#110770=CARTESIAN_POINT('Ctrl Pts',(59.9065841681356,246.608084167493,22.1472087700735)) ;
#110771=CARTESIAN_POINT('Ctrl Pts',(59.9012046744278,246.547012659867,22.2498936618512)) ;
#110772=CARTESIAN_POINT('Ctrl Pts',(59.8970619082503,246.503576654935,22.3405162958788)) ;
#110773=CARTESIAN_POINT('Ctrl Pts',(59.8886912264801,246.433344702514,22.5286238023864)) ;
#110774=CARTESIAN_POINT('Ctrl Pts',(59.8844750014276,246.406726595847,22.6257282148712)) ;
#110775=CARTESIAN_POINT('Ctrl Pts',(59.8787238383411,246.383969900176,22.7523840366644)) ;
#110776=CARTESIAN_POINT('Ctrl Pts',(59.8774438687043,246.379683156247,22.7802642735121)) ;
#110777=CARTESIAN_POINT('Ctrl Pts',(59.875262120269,246.373680316341,22.8271462900867)) ;
#110778=CARTESIAN_POINT('Ctrl Pts',(59.8743724096161,246.371581807744,22.8460935225829)) ;
#110779=CARTESIAN_POINT('Ctrl Pts',(59.8725609532958,246.368008390957,22.8842970803671)) ;
#110780=CARTESIAN_POINT('Ctrl Pts',(59.871639079679,246.366542217407,22.9035512909055)) ;
#110781=CARTESIAN_POINT('Ctrl Pts',(59.8692794575189,246.363673171748,22.9523382726886)) ;
#110782=CARTESIAN_POINT('Ctrl Pts',(59.8678281126643,246.362718043102,22.9818899504526)) ;
#110783=CARTESIAN_POINT('Ctrl Pts',(59.860554321418,246.361859930396,23.1277536837001)) ;
#110784=CARTESIAN_POINT('Ctrl Pts',(59.8543913300841,246.373271260917,23.2437999833863)) ;
#110785=CARTESIAN_POINT('Ctrl Pts',(59.843729332673,246.413410824383,23.4399273947475)) ;
#110786=CARTESIAN_POINT('Ctrl Pts',(59.8392691218913,246.436381294541,23.5207652839083)) ;
#110787=CARTESIAN_POINT('Ctrl Pts',(59.8341531008635,246.471500740201,23.6164224509797)) ;
#110788=CARTESIAN_POINT('Ctrl Pts',(59.8332625394611,246.47796669936,23.6331960574591)) ;
#110789=CARTESIAN_POINT('Ctrl Pts',(59.8318493654624,246.488831124832,23.6600841379111)) ;
#110790=CARTESIAN_POINT('Ctrl Pts',(59.8313176873039,246.493061830395,23.6702645816247)) ;
#110791=CARTESIAN_POINT('Ctrl Pts',(59.8302510504881,246.501851863298,23.6908415151552)) ;
#110792=CARTESIAN_POINT('Ctrl Pts',(59.8297164379778,246.506416933716,23.7012348250137)) ;
#110793=CARTESIAN_POINT('Ctrl Pts',(59.8282759728107,246.519139132218,23.7294191008815)) ;
#110794=CARTESIAN_POINT('Ctrl Pts',(59.8273817084125,246.527502814997,23.7471153459206)) ;
#110795=CARTESIAN_POINT('Ctrl Pts',(59.8212183621269,246.588219129601,23.8699698340151)) ;
#110796=CARTESIAN_POINT('Ctrl Pts',(59.8164385838963,246.651184154417,23.9695306862723)) ;
#110797=CARTESIAN_POINT('Ctrl Pts',(59.8081486912913,246.774001139679,24.1249108419736)) ;
#110798=CARTESIAN_POINT('Ctrl Pts',(59.8047261055606,246.828447763627,24.1844342050131)) ;
#110799=CARTESIAN_POINT('Ctrl Pts',(59.799832917847,246.908142733688,24.2598658499563)) ;
#110800=CARTESIAN_POINT('Ctrl Pts',(59.7985115037745,246.929847619416,24.2793620469127)) ;
#110801=CARTESIAN_POINT('Ctrl Pts',(59.7962798767943,246.966690635002,24.3107593601767)) ;
#110802=CARTESIAN_POINT('Ctrl Pts',(59.7953830626951,246.981545374015,24.3229837467207)) ;
#110803=CARTESIAN_POINT('Ctrl Pts',(59.793573888811,247.011582311392,24.3468476337114)) ;
#110804=CARTESIAN_POINT('Ctrl Pts',(59.7926617827875,247.026759904857,24.3584882683831)) ;
#110805=CARTESIAN_POINT('Ctrl Pts',(59.7903620554979,247.065092315258,24.3868601660425)) ;
#110806=CARTESIAN_POINT('Ctrl Pts',(59.7889622193492,247.088481093266,24.4032639201617)) ;
#110807=CARTESIAN_POINT('Ctrl Pts',(59.7844636919244,247.163799223822,24.4532691361644)) ;
#110808=CARTESIAN_POINT('Ctrl Pts',(59.7812897935359,247.217131225822,24.4845727667639)) ;
#110809=CARTESIAN_POINT('Ctrl Pts',(59.7780545670443,247.272019328904,24.5128442239351)) ;
#110810=CARTESIAN_POINT('Origin',(61.8645744874958,248.040265107786,23.0213203435596)) ;
#110811=CARTESIAN_POINT('',(59.1778464475999,247.272018857277,24.5128439810119)) ;
#110812=CARTESIAN_POINT('',(59.2757724421406,247.272018954284,24.5128440309779)) ;
#110813=CARTESIAN_POINT('',(61.8645744874958,247.272018954284,24.5128440309778)) ;
#110814=CARTESIAN_POINT('',(59.5173146749147,249.718014940025,23.0220706242834)) ;
#110815=CARTESIAN_POINT('Ctrl Pts',(59.1778464475999,247.272018857277,24.5128439810119)) ;
#110816=CARTESIAN_POINT('Ctrl Pts',(59.1805262364689,247.225785172619,24.4890301747845)) ;
#110817=CARTESIAN_POINT('Ctrl Pts',(59.1832623412498,247.180668289674,24.4630716048173)) ;
#110818=CARTESIAN_POINT('Ctrl Pts',(59.19177069459,247.045554803543,24.3767267360753)) ;
#110819=CARTESIAN_POINT('Ctrl Pts',(59.1976176759093,246.960152553852,24.3097044244426)) ;
#110820=CARTESIAN_POINT('Ctrl Pts',(59.2041114285501,246.867150441261,24.2209275633693)) ;
#110821=CARTESIAN_POINT('Ctrl Pts',(59.205120369381,246.852749898037,24.2066739592982)) ;
#110822=CARTESIAN_POINT('Ctrl Pts',(59.2066732173524,246.830590024083,24.183930915194)) ;
#110823=CARTESIAN_POINT('Ctrl Pts',(59.2072293773417,246.82265411331,24.1756169386283)) ;
#110824=CARTESIAN_POINT('Ctrl Pts',(59.2083011882245,246.807344350987,24.1592442249343)) ;
#110825=CARTESIAN_POINT('Ctrl Pts',(59.2088173564832,246.799962671476,24.1511938866593)) ;
#110826=CARTESIAN_POINT('Ctrl Pts',(59.2101438889143,246.78099308439,24.1300960312892)) ;
#110827=CARTESIAN_POINT('Ctrl Pts',(59.2109456690779,246.769528878101,24.1169384478775)) ;
#110828=CARTESIAN_POINT('Ctrl Pts',(59.2157328882929,246.701322920596,24.0361466951019)) ;
#110829=CARTESIAN_POINT('Ctrl Pts',(59.2194286999149,246.649782071289,23.9642934885275)) ;
#110830=CARTESIAN_POINT('Ctrl Pts',(59.2277907217402,246.546128817064,23.7926758277306)) ;
#110831=CARTESIAN_POINT('Ctrl Pts',(59.232442425993,246.497905741599,23.6910653928879)) ;
#110832=CARTESIAN_POINT('Ctrl Pts',(59.2387690741854,246.450122333068,23.5572187109055)) ;
#110833=CARTESIAN_POINT('Ctrl Pts',(59.2401231303217,246.440814660975,23.5287641811556)) ;
#110834=CARTESIAN_POINT('Ctrl Pts',(59.2423943677765,246.426743149611,23.4815024217254)) ;
#110835=CARTESIAN_POINT('Ctrl Pts',(59.2432970737672,246.421535287482,23.4628340877475)) ;
#110836=CARTESIAN_POINT('Ctrl Pts',(59.2451060969882,246.411861946623,23.4256835330762)) ;
#110837=CARTESIAN_POINT('Ctrl Pts',(59.2460118824369,246.407384934586,23.4072073062803)) ;
#110838=CARTESIAN_POINT('Ctrl Pts',(59.2482717202955,246.397115329551,23.3614409377309)) ;
#110839=CARTESIAN_POINT('Ctrl Pts',(59.2496370844581,246.39168773807,23.3340754454846)) ;
#110840=CARTESIAN_POINT('Ctrl Pts',(59.2563315532777,246.368777798862,23.2012969168908)) ;
#110841=CARTESIAN_POINT('Ctrl Pts',(59.2619476270299,246.36071230708,23.0945231180888)) ;
#110842=CARTESIAN_POINT('Ctrl Pts',(59.2726342336333,246.364732404227,22.8938217066899)) ;
#110843=CARTESIAN_POINT('Ctrl Pts',(59.2776634200091,246.374494562018,22.8002410163271)) ;
#110844=CARTESIAN_POINT('Ctrl Pts',(59.2833860141549,246.39569261367,22.6887405256839)) ;
#110845=CARTESIAN_POINT('Ctrl Pts',(59.2843591536899,246.399683834716,22.6695801420623)) ;
#110846=CARTESIAN_POINT('Ctrl Pts',(59.2858698682483,246.406518612943,22.6394220313487)) ;
#110847=CARTESIAN_POINT('Ctrl Pts',(59.2864186963647,246.409140070377,22.628376255911)) ;
#110848=CARTESIAN_POINT('Ctrl Pts',(59.2874878933858,246.414528584567,22.6066549149141)) ;
#110849=CARTESIAN_POINT('Ctrl Pts',(59.288008540993,246.417289154133,22.5959784552958)) ;
#110850=CARTESIAN_POINT('Ctrl Pts',(59.2893636120749,246.424828210806,22.567963848282)) ;
#110851=CARTESIAN_POINT('Ctrl Pts',(59.2901887187188,246.429780675887,22.5506735339747)) ;
#110852=CARTESIAN_POINT('Ctrl Pts',(59.2948029032425,246.459466541709,22.4529940943306)) ;
#110853=CARTESIAN_POINT('Ctrl Pts',(59.2983337978351,246.489941376754,22.3744683306017)) ;
#110854=CARTESIAN_POINT('Ctrl Pts',(59.3066863236911,246.576165043054,22.1938427726764)) ;
#110855=CARTESIAN_POINT('Ctrl Pts',(59.3114854116076,246.636877313754,22.0946007726532)) ;
#110856=CARTESIAN_POINT('Ctrl Pts',(59.3179725400787,246.72530908657,21.978913810968)) ;
#110857=CARTESIAN_POINT('Ctrl Pts',(59.3193119381519,246.743898108902,21.95588465756)) ;
#110858=CARTESIAN_POINT('Ctrl Pts',(59.3215654172298,246.775611956246,21.9186551166341)) ;
#110859=CARTESIAN_POINT('Ctrl Pts',(59.3224655108632,246.788390810563,21.9041682037294)) ;
#110860=CARTESIAN_POINT('Ctrl Pts',(59.3242746181335,246.814271467177,21.8758300465532)) ;
#110861=CARTESIAN_POINT('Ctrl Pts',(59.3251832237285,246.827364891083,21.8619750735617)) ;
#110862=CARTESIAN_POINT('Ctrl Pts',(59.3274606787177,246.860400006349,21.828190805582)) ;
#110863=CARTESIAN_POINT('Ctrl Pts',(59.3288412345459,246.880612848469,21.8085358320895)) ;
#110864=CARTESIAN_POINT('Ctrl Pts',(59.3351422846897,246.973672327309,21.7224989984122)) ;
#110865=CARTESIAN_POINT('Ctrl Pts',(59.3403006963104,247.051779716983,21.6621111580782)) ;
#110866=CARTESIAN_POINT('Ctrl Pts',(59.3510002120209,247.221185028564,21.5534984433146)) ;
#110867=CARTESIAN_POINT('Ctrl Pts',(59.3565238075376,247.312556380683,21.5061189539152)) ;
#110868=CARTESIAN_POINT('Ctrl Pts',(59.3626484798939,247.42524334896,21.4602462000249)) ;
#110869=CARTESIAN_POINT('Ctrl Pts',(59.363589624051,247.442917261678,21.4533981992962)) ;
#110870=CARTESIAN_POINT('Ctrl Pts',(59.3650625843092,247.471237992364,21.4429733590442)) ;
#110871=CARTESIAN_POINT('Ctrl Pts',(59.3656047862379,247.481810853277,21.4392015363143)) ;
#110872=CARTESIAN_POINT('Ctrl Pts',(59.3666723629663,247.502948963701,21.4318989112463)) ;
#110873=CARTESIAN_POINT('Ctrl Pts',(59.367197791234,247.513513080998,21.4283666588737)) ;
#110874=CARTESIAN_POINT('Ctrl Pts',(59.3685823678694,247.54174593161,21.4192382098166)) ;
#110875=CARTESIAN_POINT('Ctrl Pts',(59.3694314298216,247.559473929841,21.4138289986105)) ;
#110876=CARTESIAN_POINT('Ctrl Pts',(59.3738892527358,247.65444180146,21.3865638739216)) ;
#110877=CARTESIAN_POINT('Ctrl Pts',(59.3772673473169,247.733091853232,21.3699769526928)) ;
#110878=CARTESIAN_POINT('Ctrl Pts',(59.3856151217524,247.931151469249,21.3428539355113)) ;
#110879=CARTESIAN_POINT('Ctrl Pts',(59.3905519373948,248.051065239868,21.3393462045111)) ;
#110880=CARTESIAN_POINT('Ctrl Pts',(59.3971877515056,248.199439791846,21.3508828710565)) ;
#110881=CARTESIAN_POINT('Ctrl Pts',(59.3985105549316,248.228490623729,21.3539064870433)) ;
#110882=CARTESIAN_POINT('Ctrl Pts',(59.400743969436,248.27653020596,21.3601778910361)) ;
#110883=CARTESIAN_POINT('Ctrl Pts',(59.4016411387878,248.295568800932,21.3629972652574)) ;
#110884=CARTESIAN_POINT('Ctrl Pts',(59.4034505947073,248.333422397931,21.3692702081686)) ;
#110885=CARTESIAN_POINT('Ctrl Pts',(59.4043626173041,248.35223520456,21.3727192795222)) ;
#110886=CARTESIAN_POINT('Ctrl Pts',(59.4066612670227,248.39896894871,21.3821158391385)) ;
#110887=CARTESIAN_POINT('Ctrl Pts',(59.408060079665,248.426804104621,21.3884555805986)) ;
#110888=CARTESIAN_POINT('Ctrl Pts',(59.4140854195912,248.544152186667,21.4183514978897)) ;
#110889=CARTESIAN_POINT('Ctrl Pts',(59.4189169681766,248.631787100732,21.4485808066904)) ;
#110890=CARTESIAN_POINT('Ctrl Pts',(59.4296378346349,248.816549827562,21.5299502541684)) ;
#110891=CARTESIAN_POINT('Ctrl Pts',(59.4355369521123,248.912080608784,21.5837034246399)) ;
#110892=CARTESIAN_POINT('Ctrl Pts',(59.4419455224123,249.016621536164,21.6568041053846)) ;
#110893=CARTESIAN_POINT('Ctrl Pts',(59.4428479210382,249.031369659197,21.6674783083586)) ;
#110894=CARTESIAN_POINT('Ctrl Pts',(59.4442751107914,249.054803469309,21.6850271316829)) ;
#110895=CARTESIAN_POINT('Ctrl Pts',(59.4448092716059,249.063599668567,21.6917512299296)) ;
#110896=CARTESIAN_POINT('Ctrl Pts',(59.4458760480371,249.08123729999,21.7055127484445)) ;
#110897=CARTESIAN_POINT('Ctrl Pts',(59.4464084154968,249.090075435629,21.7125533586212)) ;
#110898=CARTESIAN_POINT('Ctrl Pts',(59.4478349886522,249.113824689174,21.7318678081727)) ;
#110899=CARTESIAN_POINT('Ctrl Pts',(59.4487179883856,249.128596437354,21.744310951591)) ;
#110900=CARTESIAN_POINT('Ctrl Pts',(59.4524360961693,249.190846680087,21.7986130577541)) ;
#110901=CARTESIAN_POINT('Ctrl Pts',(59.4551357772857,249.236153651935,21.8428880178773)) ;
#110902=CARTESIAN_POINT('Ctrl Pts',(59.4634328941075,249.369376348737,21.9886933902383)) ;
#110903=CARTESIAN_POINT('Ctrl Pts',(59.4689004280523,249.447681155356,22.0982631211536)) ;
#110904=CARTESIAN_POINT('Ctrl Pts',(59.4761999283544,249.526346155825,22.2420326360001)) ;
#110905=CARTESIAN_POINT('Ctrl Pts',(59.4775432949157,249.539900549804,22.2684460961854)) ;
#110906=CARTESIAN_POINT('Ctrl Pts',(59.4798015786771,249.561114241396,22.3126336904868)) ;
#110907=CARTESIAN_POINT('Ctrl Pts',(59.4807023769587,249.569179638151,22.3302058947182)) ;
#110908=CARTESIAN_POINT('Ctrl Pts',(59.4825114413461,249.584584640663,22.3653591731933)) ;
#110909=CARTESIAN_POINT('Ctrl Pts',(59.4834192655936,249.591932047347,22.3829336669998)) ;
#110910=CARTESIAN_POINT('Ctrl Pts',(59.4856918521451,249.609377443325,22.4267434817076)) ;
#110911=CARTESIAN_POINT('Ctrl Pts',(59.4870682115034,249.619118077597,22.4531140881108)) ;
#110912=CARTESIAN_POINT('Ctrl Pts',(59.4938356197225,249.663067096999,22.5819679337792)) ;
#110913=CARTESIAN_POINT('Ctrl Pts',(59.4995201046604,249.687980812302,22.6873375349047)) ;
#110914=CARTESIAN_POINT('Ctrl Pts',(59.5093266138071,249.712896146806,22.869822058914)) ;
#110915=CARTESIAN_POINT('Ctrl Pts',(59.5133969118513,249.718049001863,22.945902810493)) ;
#110916=CARTESIAN_POINT('Ctrl Pts',(59.5173146749147,249.718014940025,23.0220706242834)) ;
#110917=CARTESIAN_POINT('Ctrl Pts',(59.5173148011493,249.718014938926,23.0220730784946)) ;
#110918=CARTESIAN_POINT('Ctrl Pts',(59.5187308942661,249.718002586838,23.0496043024628)) ;
#110919=CARTESIAN_POINT('Ctrl Pts',(59.520125791784,249.717312569216,23.0771326893012)) ;
#110920=CARTESIAN_POINT('Ctrl Pts',(59.5220396377411,249.715394524352,23.1157105614426)) ;
#110921=CARTESIAN_POINT('Ctrl Pts',(59.5225841699245,249.71473392328,23.1267825312265)) ;
#110922=CARTESIAN_POINT('Ctrl Pts',(59.5235968137477,249.713286273174,23.1475753839361)) ;
#110923=CARTESIAN_POINT('Ctrl Pts',(59.5240661907489,249.712524163427,23.1572976206492)) ;
#110924=CARTESIAN_POINT('Ctrl Pts',(59.5250769350779,249.710681659853,23.1784351450741)) ;
#110925=CARTESIAN_POINT('Ctrl Pts',(59.5256165125746,249.709568940235,23.1898470380258)) ;
#110926=CARTESIAN_POINT('Ctrl Pts',(59.5270868280488,249.706181119012,23.2212550563819)) ;
#110927=CARTESIAN_POINT('Ctrl Pts',(59.528005147852,249.703663047617,23.2412235046442)) ;
#110928=CARTESIAN_POINT('Ctrl Pts',(59.5328093928304,249.688369264406,23.3471171650295)) ;
#110929=CARTESIAN_POINT('Ctrl Pts',(59.536434848772,249.669292901835,23.4320048008461)) ;
#110930=CARTESIAN_POINT('Ctrl Pts',(59.5412198095171,249.635516970733,23.5416998057986)) ;
#110931=CARTESIAN_POINT('Ctrl Pts',(59.5423811561681,249.626644012976,23.5681523582366)) ;
#110932=CARTESIAN_POINT('Ctrl Pts',(59.5469722036763,249.589158223124,23.6713011119839)) ;
#110933=CARTESIAN_POINT('Ctrl Pts',(59.5504450930294,249.555610087597,23.7460776470531)) ;
#110934=CARTESIAN_POINT('Ctrl Pts',(59.5554015745482,249.502801234747,23.8439349139661)) ;
#110935=CARTESIAN_POINT('Ctrl Pts',(59.5567307583138,249.488186245953,23.8693951717872)) ;
#110936=CARTESIAN_POINT('Ctrl Pts',(59.558971881816,249.462881488672,23.9109152687918)) ;
#110937=CARTESIAN_POINT('Ctrl Pts',(59.5598701708822,249.452569012188,23.9271978977621)) ;
#110938=CARTESIAN_POINT('Ctrl Pts',(59.5616794590218,249.431482197501,23.9592568566776)) ;
#110939=CARTESIAN_POINT('Ctrl Pts',(59.5625901382069,249.42071435872,23.9750339914206)) ;
#110940=CARTESIAN_POINT('Ctrl Pts',(59.5648804736064,249.393268714089,24.0138087225754)) ;
#110941=CARTESIAN_POINT('Ctrl Pts',(59.5662721268453,249.376272168342,24.0365725065368)) ;
#110942=CARTESIAN_POINT('Ctrl Pts',(59.5739523041733,249.280784807041,24.1579080939915)) ;
#110943=CARTESIAN_POINT('Ctrl Pts',(59.5806549468218,249.191965734632,24.2478187763718)) ;
#110944=CARTESIAN_POINT('Ctrl Pts',(59.5901990676382,249.052410741105,24.3604447505936)) ;
#110945=CARTESIAN_POINT('Ctrl Pts',(59.5930275059842,249.009305029107,24.3919607088536)) ;
#110946=CARTESIAN_POINT('Ctrl Pts',(59.596965985669,248.945689939851,24.4339680981686)) ;
#110947=CARTESIAN_POINT('Ctrl Pts',(59.5981335850957,248.926354496423,24.4461759417771)) ;
#110948=CARTESIAN_POINT('Ctrl Pts',(59.6001963531454,248.891194019983,24.4673826262163)) ;
#110949=CARTESIAN_POINT('Ctrl Pts',(59.6010983245476,248.875460697278,24.4765263478056)) ;
#110950=CARTESIAN_POINT('Ctrl Pts',(59.6025250103263,248.849921290618,24.490818374756)) ;
#110951=CARTESIAN_POINT('Ctrl Pts',(59.6030590833381,248.840207818122,24.4961285597051)) ;
#110952=CARTESIAN_POINT('Ctrl Pts',(59.6041258592792,248.820472999704,24.5066648899307)) ;
#110953=CARTESIAN_POINT('Ctrl Pts',(59.6046583105073,248.81045004299,24.5118866636684)) ;
#110954=CARTESIAN_POINT('Ctrl Pts',(59.6060853906529,248.783150120489,24.5257605175601)) ;
#110955=CARTESIAN_POINT('Ctrl Pts',(59.6069687998426,248.765774841195,24.534216262099)) ;
#110956=CARTESIAN_POINT('Ctrl Pts',(59.6122757365485,248.658878232088,24.5839726213769)) ;
#110957=CARTESIAN_POINT('Ctrl Pts',(59.6163536363015,248.565998675546,24.6176197964051)) ;
#110958=CARTESIAN_POINT('Ctrl Pts',(59.6246698344004,248.373169096507,24.6688037265239)) ;
#110959=CARTESIAN_POINT('Ctrl Pts',(59.6288983498874,248.273510653106,24.6858386676765)) ;
#110960=CARTESIAN_POINT('Ctrl Pts',(59.6346832530808,248.144329734024,24.6960856601306)) ;
#110961=CARTESIAN_POINT('Ctrl Pts',(59.6359841411847,248.11567482639,24.697620309563)) ;
#110962=CARTESIAN_POINT('Ctrl Pts',(59.6381911332643,248.067850840389,24.6989528702247)) ;
#110963=CARTESIAN_POINT('Ctrl Pts',(59.6390845053475,248.04869889806,24.6991584473113)) ;
#110964=CARTESIAN_POINT('Ctrl Pts',(59.6408948820142,248.010331445425,24.6989133611145)) ;
#110965=CARTESIAN_POINT('Ctrl Pts',(59.6418118200348,247.991118858991,24.6984604585725)) ;
#110966=CARTESIAN_POINT('Ctrl Pts',(59.6441407199324,247.942893465726,24.6964942729807)) ;
#110967=CARTESIAN_POINT('Ctrl Pts',(59.6455655594682,247.913905025383,24.6945573055447)) ;
#110968=CARTESIAN_POINT('Ctrl Pts',(59.6530372784655,247.764548728882,24.6806741818089)) ;
#110969=CARTESIAN_POINT('Ctrl Pts',(59.6594587820107,247.645692176022,24.6564899854684)) ;
#110970=CARTESIAN_POINT('Ctrl Pts',(59.6701882789886,247.453705534772,24.5952605478754)) ;
#110971=CARTESIAN_POINT('Ctrl Pts',(59.6744624274261,247.378784043383,24.5652712557968)) ;
#110972=CARTESIAN_POINT('Ctrl Pts',(59.6791490969792,247.294811225893,24.5244194538945)) ;
#110973=CARTESIAN_POINT('Ctrl Pts',(59.6797845335315,247.283381906269,24.5186968003499)) ;
#110974=CARTESIAN_POINT('Ctrl Pts',(59.6804129742801,247.272018954245,24.5128440309576)) ;
#110975=CARTESIAN_POINT('Ctrl Pts',(59.7780545670443,247.272019328904,24.5128442239351)) ;
#110976=CARTESIAN_POINT('Ctrl Pts',(59.774761794154,247.327883750854,24.5416185579683)) ;
#110977=CARTESIAN_POINT('Ctrl Pts',(59.7714055505668,247.385360102237,24.5672519396114)) ;
#110978=CARTESIAN_POINT('Ctrl Pts',(59.7651852062337,247.494600491515,24.6087724922865)) ;
#110979=CARTESIAN_POINT('Ctrl Pts',(59.762325360688,247.545914614006,24.6254937168973)) ;
#110980=CARTESIAN_POINT('Ctrl Pts',(59.7583490811463,247.620134709861,24.6457785904628)) ;
#110981=CARTESIAN_POINT('Ctrl Pts',(59.7571740831682,247.642445978209,24.6513860366435)) ;
#110982=CARTESIAN_POINT('Ctrl Pts',(59.7550998233612,247.682679481403,24.6606225172389)) ;
#110983=CARTESIAN_POINT('Ctrl Pts',(59.7541936532009,247.700559010831,24.6644207402717)) ;
#110984=CARTESIAN_POINT('Ctrl Pts',(59.7527620710491,247.729376717799,24.6700520818001)) ;
#110985=CARTESIAN_POINT('Ctrl Pts',(59.7522271907319,247.740276916286,24.6720701841887)) ;
#110986=CARTESIAN_POINT('Ctrl Pts',(59.7511605958433,247.762307184996,24.6759235213669)) ;
#110987=CARTESIAN_POINT('Ctrl Pts',(59.7506290965651,247.773437306327,24.6777548337123)) ;
#110988=CARTESIAN_POINT('Ctrl Pts',(59.7492074792761,247.803581987803,24.6824030074996)) ;
#110989=CARTESIAN_POINT('Ctrl Pts',(59.7483284357257,247.822628278194,24.685005644251)) ;
#110990=CARTESIAN_POINT('Ctrl Pts',(59.7429653475135,247.940912304063,24.6991027499984)) ;
#110991=CARTESIAN_POINT('Ctrl Pts',(59.7388373156994,248.040975550861,24.7020427459108)) ;
#110992=CARTESIAN_POINT('Ctrl Pts',(59.7304696760117,248.241339005617,24.6900253734806)) ;
#110993=CARTESIAN_POINT('Ctrl Pts',(59.7262411098734,248.34121223189,24.6749334012655)) ;
#110994=CARTESIAN_POINT('Ctrl Pts',(59.7204756214179,248.466519057224,24.644264668261)) ;
#110995=CARTESIAN_POINT('Ctrl Pts',(59.7191955308437,248.493743133007,24.6368692551899)) ;
#110996=CARTESIAN_POINT('Ctrl Pts',(59.7170136347423,248.539031252983,24.6233318240841)) ;
#110997=CARTESIAN_POINT('Ctrl Pts',(59.7161239010689,248.557200644494,24.6175615743021)) ;
#110998=CARTESIAN_POINT('Ctrl Pts',(59.7143124464029,248.593567907158,24.6053259923635)) ;
#110999=CARTESIAN_POINT('Ctrl Pts',(59.7133905985666,248.611760312604,24.5988535685712)) ;
#111000=CARTESIAN_POINT('Ctrl Pts',(59.7110311466097,248.657511589341,24.5816810893695)) ;
#111001=CARTESIAN_POINT('Ctrl Pts',(59.7095799503321,248.684906112866,24.5705642606709)) ;
#111002=CARTESIAN_POINT('Ctrl Pts',(59.7023049196112,248.818594572278,24.5121529646731)) ;
#111003=CARTESIAN_POINT('Ctrl Pts',(59.696140338342,248.920052083842,24.4546197581295)) ;
#111004=CARTESIAN_POINT('Ctrl Pts',(59.6854779745309,249.083021796893,24.3383403192104)) ;
#111005=CARTESIAN_POINT('Ctrl Pts',(59.6810189661873,249.14756740238,24.284556888648)) ;
#111006=CARTESIAN_POINT('Ctrl Pts',(59.6759040712347,249.220729409296,24.2136592905779)) ;
#111007=CARTESIAN_POINT('Ctrl Pts',(59.6750135496421,249.233435858065,24.200943901888)) ;
#111008=CARTESIAN_POINT('Ctrl Pts',(59.6736004212274,249.253601868926,24.1801044001107)) ;
#111009=CARTESIAN_POINT('Ctrl Pts',(59.6730687499222,249.261189781961,24.1721068323961)) ;
#111010=CARTESIAN_POINT('Ctrl Pts',(59.6720021109092,249.276429952263,24.155723442942)) ;
#111011=CARTESIAN_POINT('Ctrl Pts',(59.6714674896903,249.284076967901,24.1473336580495)) ;
#111012=CARTESIAN_POINT('Ctrl Pts',(59.6700269700435,249.30467527621,24.1242686875443)) ;
#111013=CARTESIAN_POINT('Ctrl Pts',(59.6691326614019,249.317456159265,24.109443129741)) ;
#111014=CARTESIAN_POINT('Ctrl Pts',(59.6640307037729,249.390011486994,24.0222402705537)) ;
#111015=CARTESIAN_POINT('Ctrl Pts',(59.6601335143789,249.443891693565,23.9451663070665)) ;
#111016=CARTESIAN_POINT('Ctrl Pts',(59.6517667254847,249.544720537382,23.771573505906)) ;
#111017=CARTESIAN_POINT('Ctrl Pts',(59.6473018333757,249.589441737181,23.6742489334558)) ;
#111018=CARTESIAN_POINT('Ctrl Pts',(59.6412747623058,249.633780750475,23.546992653337)) ;
#111019=CARTESIAN_POINT('Ctrl Pts',(59.6400078404709,249.642301593623,23.5204220132433)) ;
#111020=CARTESIAN_POINT('Ctrl Pts',(59.6378417115146,249.655507120173,23.475412433816)) ;
#111021=CARTESIAN_POINT('Ctrl Pts',(59.6369541621637,249.660548018405,23.4570836271768)) ;
#111022=CARTESIAN_POINT('Ctrl Pts',(59.6351415088113,249.670095850163,23.4199080815493)) ;
#111023=CARTESIAN_POINT('Ctrl Pts',(59.634216149424,249.674589859489,23.4010610460801)) ;
#111024=CARTESIAN_POINT('Ctrl Pts',(59.6318353408483,249.685190146919,23.3529249872554)) ;
#111025=CARTESIAN_POINT('Ctrl Pts',(59.6303657969879,249.690841079606,23.3235435136852)) ;
#111026=CARTESIAN_POINT('Ctrl Pts',(59.623263615938,249.713974244059,23.1831163693322)) ;
#111027=CARTESIAN_POINT('Ctrl Pts',(59.6173173192074,249.721050621605,23.0706617828455)) ;
#111028=CARTESIAN_POINT('Ctrl Pts',(59.6066511748029,249.713535852349,22.8705510765495)) ;
#111029=CARTESIAN_POINT('Ctrl Pts',(59.6019716717976,249.703344836954,22.783131050542)) ;
#111030=CARTESIAN_POINT('Ctrl Pts',(59.5966832838548,249.682953897403,22.6796664194113)) ;
#111031=CARTESIAN_POINT('Ctrl Pts',(59.5958135164287,249.679285212283,22.6624791466082)) ;
#111032=CARTESIAN_POINT('Ctrl Pts',(59.5944248058086,249.672894524959,22.6346861150518)) ;
#111033=CARTESIAN_POINT('Ctrl Pts',(59.5938973284434,249.670337607899,22.6240439865378)) ;
#111034=CARTESIAN_POINT('Ctrl Pts',(59.5928301761248,249.664891550901,22.602315315598)) ;
#111035=CARTESIAN_POINT('Ctrl Pts',(59.5922910315064,249.661992671096,22.5912319607847)) ;
#111036=CARTESIAN_POINT('Ctrl Pts',(59.5908230508129,249.653700155936,22.5608035776308)) ;
#111037=CARTESIAN_POINT('Ctrl Pts',(59.5899065697292,249.648072241925,22.5415239012834)) ;
#111038=CARTESIAN_POINT('Ctrl Pts',(59.5849910277009,249.615518922208,22.4370188126257)) ;
#111039=CARTESIAN_POINT('Ctrl Pts',(59.5812686711442,249.582160356368,22.3539415299896)) ;
#111040=CARTESIAN_POINT('Ctrl Pts',(59.5729218036873,249.492950912579,22.1746562990521)) ;
#111041=CARTESIAN_POINT('Ctrl Pts',(59.5683025964055,249.433847722074,22.0805432491439)) ;
#111042=CARTESIAN_POINT('Ctrl Pts',(59.5621024417683,249.348914668885,21.9710588354632)) ;
#111043=CARTESIAN_POINT('Ctrl Pts',(59.5608436740857,249.331390763142,21.9495893367198)) ;
#111044=CARTESIAN_POINT('Ctrl Pts',(59.5586872849192,249.300984759523,21.914165845468)) ;
#111045=CARTESIAN_POINT('Ctrl Pts',(59.5578010668375,249.28838269399,21.8999784782596)) ;
#111046=CARTESIAN_POINT('Ctrl Pts',(59.5559875399162,249.262403415081,21.8717116882523)) ;
#111047=CARTESIAN_POINT('Ctrl Pts',(59.5550598940995,249.249016987054,21.8576447194599)) ;
#111048=CARTESIAN_POINT('Ctrl Pts',(59.5526652158698,249.214231694936,21.8223389683243)) ;
#111049=CARTESIAN_POINT('Ctrl Pts',(59.5511837595219,249.192499602197,21.801439442893)) ;
#111050=CARTESIAN_POINT('Ctrl Pts',(59.5453676721818,249.106389150695,21.722982725395)) ;
#111051=CARTESIAN_POINT('Ctrl Pts',(59.5408631118082,249.038173399908,21.6698480468623)) ;
#111052=CARTESIAN_POINT('Ctrl Pts',(59.5321061176216,248.900542143154,21.5787658566816)) ;
#111053=CARTESIAN_POINT('Ctrl Pts',(59.527879502502,248.831929939601,21.5400009696296)) ;
#111054=CARTESIAN_POINT('Ctrl Pts',(59.5223074232035,248.735466302676,21.4941234324246)) ;
#111055=CARTESIAN_POINT('Ctrl Pts',(59.5208580733492,248.709782671801,21.4826906083421)) ;
#111056=CARTESIAN_POINT('Ctrl Pts',(59.5183634155121,248.664267267667,21.4637855062765)) ;
#111057=CARTESIAN_POINT('Ctrl Pts',(59.5173068652299,248.644558704881,21.4560335369966)) ;
#111058=CARTESIAN_POINT('Ctrl Pts',(59.515698250874,248.613762793008,21.4445889754111)) ;
#111059=CARTESIAN_POINT('Ctrl Pts',(59.5151325552097,248.602775230741,21.4406357519086)) ;
#111060=CARTESIAN_POINT('Ctrl Pts',(59.5140626043835,248.581663938695,21.4332881171425)) ;
#111061=CARTESIAN_POINT('Ctrl Pts',(59.5135573903211,248.571547621024,21.4298751074472)) ;
#111062=CARTESIAN_POINT('Ctrl Pts',(59.5122748658985,248.545512104935,21.4213672535861)) ;
#111063=CARTESIAN_POINT('Ctrl Pts',(59.511505263184,248.529547687484,21.4164131773161)) ;
#111064=CARTESIAN_POINT('Ctrl Pts',(59.5079262555667,248.453902052813,21.3941725424164)) ;
#111065=CARTESIAN_POINT('Ctrl Pts',(59.5052581977839,248.393360519861,21.3799702131822)) ;
#111066=CARTESIAN_POINT('Ctrl Pts',(59.4996340259662,248.26199503237,21.3567607345253)) ;
#111067=CARTESIAN_POINT('Ctrl Pts',(59.4966972215952,248.191104367986,21.3488459574273)) ;
#111068=CARTESIAN_POINT('Ctrl Pts',(59.4915022641246,248.067678804981,21.3429790930685)) ;
#111069=CARTESIAN_POINT('Ctrl Pts',(59.4892750213532,248.015347367843,21.3429402932568)) ;
#111070=CARTESIAN_POINT('Ctrl Pts',(59.4852852154806,247.924292856095,21.3471325413208)) ;
#111071=CARTESIAN_POINT('Ctrl Pts',(59.4835520019177,247.88555993595,21.3502666584703)) ;
#111072=CARTESIAN_POINT('Ctrl Pts',(59.4808168830331,247.826069783601,21.3571664407301)) ;
#111073=CARTESIAN_POINT('Ctrl Pts',(59.4798442104066,247.805215456688,21.3599836937173)) ;
#111074=CARTESIAN_POINT('Ctrl Pts',(59.4779985574567,247.766250544468,21.3659958810795)) ;
#111075=CARTESIAN_POINT('Ctrl Pts',(59.4771286314416,247.748128710412,21.3690977950707)) ;
#111076=CARTESIAN_POINT('Ctrl Pts',(59.4751231416628,247.706926102166,21.3768494918451)) ;
#111077=CARTESIAN_POINT('Ctrl Pts',(59.4739817338708,247.683885235584,21.3816884970079)) ;
#111078=CARTESIAN_POINT('Ctrl Pts',(59.4703541573072,247.611954166381,21.3983831395589)) ;
#111079=CARTESIAN_POINT('Ctrl Pts',(59.4678153528255,247.563493579279,21.4119528557484)) ;
#111080=CARTESIAN_POINT('Ctrl Pts',(59.4590396175844,247.401795136794,21.4651758203841)) ;
#111081=CARTESIAN_POINT('Ctrl Pts',(59.4525458340495,247.292224243684,21.5147810328645)) ;
#111082=CARTESIAN_POINT('Ctrl Pts',(59.4436696934603,247.146681567672,21.6004920259415)) ;
#111083=CARTESIAN_POINT('Ctrl Pts',(59.4411363442711,247.105577499193,21.6271882236737)) ;
#111084=CARTESIAN_POINT('Ctrl Pts',(59.4379188436745,247.05302158639,21.6646929711772)) ;
#111085=CARTESIAN_POINT('Ctrl Pts',(59.4371522566458,247.04047100183,21.6739156621638)) ;
#111086=CARTESIAN_POINT('Ctrl Pts',(59.4358831307604,247.019601499764,21.689703621198)) ;
#111087=CARTESIAN_POINT('Ctrl Pts',(59.4353746242082,247.011213237778,21.6961752323037)) ;
#111088=CARTESIAN_POINT('Ctrl Pts',(59.434293753018,246.993314485507,21.7102567356795)) ;
#111089=CARTESIAN_POINT('Ctrl Pts',(59.4337230629041,246.983824705338,21.7178913730078)) ;
#111090=CARTESIAN_POINT('Ctrl Pts',(59.4320583899658,246.956071291668,21.7407215592049)) ;
#111091=CARTESIAN_POINT('Ctrl Pts',(59.4309828465802,246.938045794223,21.7562028957448)) ;
#111092=CARTESIAN_POINT('Ctrl Pts',(59.4252547384642,246.842143437684,21.8421755941424)) ;
#111093=CARTESIAN_POINT('Ctrl Pts',(59.4209532032415,246.770683440108,21.9194838239143)) ;
#111094=CARTESIAN_POINT('Ctrl Pts',(59.4130581662455,246.656002026043,22.0696388219923)) ;
#111095=CARTESIAN_POINT('Ctrl Pts',(59.4095090047085,246.610159526125,22.1400265909284)) ;
#111096=CARTESIAN_POINT('Ctrl Pts',(59.4044355855961,246.555262773169,22.2399614866442)) ;
#111097=CARTESIAN_POINT('Ctrl Pts',(59.4030726362694,246.541465644329,22.2667650844466)) ;
#111098=CARTESIAN_POINT('Ctrl Pts',(59.400790718495,246.519980244556,22.311421757387)) ;
#111099=CARTESIAN_POINT('Ctrl Pts',(59.3998865266387,246.51186667889,22.3290629685585)) ;
#111100=CARTESIAN_POINT('Ctrl Pts',(59.3980777747049,246.496432704842,22.3642155880455)) ;
#111101=CARTESIAN_POINT('Ctrl Pts',(59.3971738218356,246.489099638532,22.3817182805544)) ;
#111102=CARTESIAN_POINT('Ctrl Pts',(59.3949249176763,246.471791036399,22.4250802825795)) ;
#111103=CARTESIAN_POINT('Ctrl Pts',(59.3935688931329,246.462156620707,22.4510689835856)) ;
#111104=CARTESIAN_POINT('Ctrl Pts',(59.386686291932,246.417218527503,22.5821648795098)) ;
#111105=CARTESIAN_POINT('Ctrl Pts',(59.3808470178179,246.391755600703,22.6903393598047)) ;
#111106=CARTESIAN_POINT('Ctrl Pts',(59.3701828656917,246.365365456292,22.8888452760489)) ;
#111107=CARTESIAN_POINT('Ctrl Pts',(59.3654052785317,246.360685573072,22.9782762457737)) ;
#111108=CARTESIAN_POINT('Ctrl Pts',(59.3598786003915,246.363709196641,23.087711662349)) ;
#111109=CARTESIAN_POINT('Ctrl Pts',(59.3588799218448,246.364622942463,23.1077548711933)) ;
#111110=CARTESIAN_POINT('Ctrl Pts',(59.3573391963446,246.366622621998,23.1392060002222)) ;
#111111=CARTESIAN_POINT('Ctrl Pts',(59.3567851852818,246.3674662508,23.1506269406852)) ;
#111112=CARTESIAN_POINT('Ctrl Pts',(59.3557143794269,246.36934498136,23.1729476611568)) ;
#111113=CARTESIAN_POINT('Ctrl Pts',(59.3551971330036,246.370369951855,23.1838475282997)) ;
#111114=CARTESIAN_POINT('Ctrl Pts',(59.3538632957894,246.373319480054,23.2122304594866)) ;
#111115=CARTESIAN_POINT('Ctrl Pts',(59.3530554784209,246.37541244506,23.2296951304503)) ;
#111116=CARTESIAN_POINT('Ctrl Pts',(59.3484464973521,246.389119258351,23.330611797653)) ;
#111117=CARTESIAN_POINT('Ctrl Pts',(59.3449073114498,246.406732676285,23.4131341028129)) ;
#111118=CARTESIAN_POINT('Ctrl Pts',(59.3365146431292,246.463384127568,23.6060747644031)) ;
#111119=CARTESIAN_POINT('Ctrl Pts',(59.3316853673595,246.507910793797,23.7144148222799)) ;
#111120=CARTESIAN_POINT('Ctrl Pts',(59.3251656518772,246.57732484112,23.8432215865148)) ;
#111121=CARTESIAN_POINT('Ctrl Pts',(59.3238297635604,246.592006557289,23.8688242837909)) ;
#111122=CARTESIAN_POINT('Ctrl Pts',(59.3215806421183,246.61739407242,23.9105084778274)) ;
#111123=CARTESIAN_POINT('Ctrl Pts',(59.320681282857,246.627716210268,23.9268163937017)) ;
#111124=CARTESIAN_POINT('Ctrl Pts',(59.3188724490701,246.648793108471,23.9588780397437)) ;
#111125=CARTESIAN_POINT('Ctrl Pts',(59.3179633544818,246.659539758871,23.9746336355874)) ;
#111126=CARTESIAN_POINT('Ctrl Pts',(59.3156822821868,246.686867914198,24.013267572458)) ;
#111127=CARTESIAN_POINT('Ctrl Pts',(59.3142985116661,246.703762781768,24.0359161656126)) ;
#111128=CARTESIAN_POINT('Ctrl Pts',(59.3112348031537,246.741838498622,24.084356803264)) ;
#111129=CARTESIAN_POINT('Ctrl Pts',(59.3095472147758,246.763233071231,24.1099649922655)) ;
#111130=CARTESIAN_POINT('Ctrl Pts',(59.3041223612164,246.833398297222,24.1890327113843)) ;
#111131=CARTESIAN_POINT('Ctrl Pts',(59.3002965380526,246.884867880334,24.2399817859792)) ;
#111132=CARTESIAN_POINT('Ctrl Pts',(59.2914262774161,247.010615316636,24.3493099009446)) ;
#111133=CARTESIAN_POINT('Ctrl Pts',(59.2863765328242,247.086860945118,24.4050679017676)) ;
#111134=CARTESIAN_POINT('Ctrl Pts',(59.2806379440077,247.184068925345,24.4642876270644)) ;
#111135=CARTESIAN_POINT('Ctrl Pts',(59.2796668443651,247.200924459311,24.4741568170896)) ;
#111136=CARTESIAN_POINT('Ctrl Pts',(59.278158591979,247.227835958453,24.4892892113407)) ;
#111137=CARTESIAN_POINT('Ctrl Pts',(59.2776102411725,247.237779201986,24.4947483546354)) ;
#111138=CARTESIAN_POINT('Ctrl Pts',(59.276632254559,247.255822990797,24.5044180988372)) ;
#111139=CARTESIAN_POINT('Ctrl Pts',(59.2762004036355,247.263903808271,24.5086641243746)) ;
#111140=CARTESIAN_POINT('Ctrl Pts',(59.2757724421406,247.272018954284,24.5128440309779)) ;
#111141=CARTESIAN_POINT('Origin',(61.8645744874958,248.040265107786,23.0213203435596)) ;
#111142=CARTESIAN_POINT('',(58.6780583779715,247.272018809212,24.512843956255)) ;
#111143=CARTESIAN_POINT('',(58.7781769759756,247.272019165218,24.5128441396244)) ;
#111144=CARTESIAN_POINT('',(61.8645744874958,247.272018954284,24.5128440309778)) ;
#111145=CARTESIAN_POINT('Ctrl Pts',(58.6780583779715,247.272018809212,24.512843956255)) ;
#111146=CARTESIAN_POINT('Ctrl Pts',(58.6800068924602,247.231512300371,24.4919800723578)) ;
#111147=CARTESIAN_POINT('Ctrl Pts',(58.6819912802419,247.191850795628,24.469463559986)) ;
#111148=CARTESIAN_POINT('Ctrl Pts',(58.6852925950531,247.129145477612,24.4303998213336)) ;
#111149=CARTESIAN_POINT('Ctrl Pts',(58.6865751585715,247.105537624819,24.4148512480985)) ;
#111150=CARTESIAN_POINT('Ctrl Pts',(58.6887601557558,247.06667367633,24.3878226944819)) ;
#111151=CARTESIAN_POINT('Ctrl Pts',(58.6896504429267,247.051200149417,24.3766651052517)) ;
#111152=CARTESIAN_POINT('Ctrl Pts',(58.6914621087527,247.020459040762,24.3536916206181)) ;
#111153=CARTESIAN_POINT('Ctrl Pts',(58.6923835933263,247.005198464231,24.341871228463)) ;
#111154=CARTESIAN_POINT('Ctrl Pts',(58.6947401655318,246.96713070797,24.3113197523509)) ;
#111155=CARTESIAN_POINT('Ctrl Pts',(58.6961887716055,246.944608137751,24.2922458266315)) ;
#111156=CARTESIAN_POINT('Ctrl Pts',(58.7034865319802,246.835449869319,24.1947429378636)) ;
#111157=CARTESIAN_POINT('Ctrl Pts',(58.7096801360837,246.756679787355,24.1080137953495)) ;
#111158=CARTESIAN_POINT('Ctrl Pts',(58.7203497328208,246.638165635079,23.9464885838306)) ;
#111159=CARTESIAN_POINT('Ctrl Pts',(58.7247873478086,246.593856025307,23.8755578817659)) ;
#111160=CARTESIAN_POINT('Ctrl Pts',(58.7298822590129,246.546657306,23.7857177662923)) ;
#111161=CARTESIAN_POINT('Ctrl Pts',(58.7307721363177,246.538559141151,23.7696831713953)) ;
#111162=CARTESIAN_POINT('Ctrl Pts',(58.7321845691273,246.525909293868,23.7436035490382)) ;
#111163=CARTESIAN_POINT('Ctrl Pts',(58.7327161714001,246.521196516751,23.7336385260547)) ;
#111164=CARTESIAN_POINT('Ctrl Pts',(58.7337830046694,246.51182804092,23.7133132471223)) ;
#111165=CARTESIAN_POINT('Ctrl Pts',(58.7343178820646,246.507178687058,23.7029508048126)) ;
#111166=CARTESIAN_POINT('Ctrl Pts',(58.7357597144667,246.494795213463,23.674582808946)) ;
#111167=CARTESIAN_POINT('Ctrl Pts',(58.7366550452951,246.487270567014,23.656487294631)) ;
#111168=CARTESIAN_POINT('Ctrl Pts',(58.7417491617437,246.445617614282,23.551150247605)) ;
#111169=CARTESIAN_POINT('Ctrl Pts',(58.7456389575049,246.418524230147,23.4612974253404)) ;
#111170=CARTESIAN_POINT('Ctrl Pts',(58.7540021755883,246.376862887085,23.2650036127155)) ;
#111171=CARTESIAN_POINT('Ctrl Pts',(58.7584709205864,246.36471336984,23.1584804108466)) ;
#111172=CARTESIAN_POINT('Ctrl Pts',(58.7645033374796,246.362284364243,23.0236165178458)) ;
#111173=CARTESIAN_POINT('Ctrl Pts',(58.7657711570691,246.362478537671,22.9956928014189)) ;
#111174=CARTESIAN_POINT('Ctrl Pts',(58.7679384458552,246.36397605214,22.9487834829235)) ;
#111175=CARTESIAN_POINT('Ctrl Pts',(58.7688262306036,246.364905742131,22.9297913596818)) ;
#111176=CARTESIAN_POINT('Ctrl Pts',(58.7706390536231,246.367433967197,22.8914882791098)) ;
#111177=CARTESIAN_POINT('Ctrl Pts',(58.771564340197,246.369044648063,22.8721810583319)) ;
#111178=CARTESIAN_POINT('Ctrl Pts',(58.773944291295,246.373990673928,22.823157279201)) ;
#111179=CARTESIAN_POINT('Ctrl Pts',(58.7754130269918,246.377786686637,22.793494867268)) ;
#111180=CARTESIAN_POINT('Ctrl Pts',(58.7825252867883,246.399650464576,22.6526554152987)) ;
#111181=CARTESIAN_POINT('Ctrl Pts',(58.7884839693428,246.428089011615,22.5433948972293)) ;
#111182=CARTESIAN_POINT('Ctrl Pts',(58.7991001305919,246.497407177365,22.3565249039626)) ;
#111183=CARTESIAN_POINT('Ctrl Pts',(58.8037172290047,246.533822426037,22.2776834042871)) ;
#111184=CARTESIAN_POINT('Ctrl Pts',(58.8089802150941,246.584999227896,22.1862316864812)) ;
#111185=CARTESIAN_POINT('Ctrl Pts',(58.8098760663716,246.59408175224,22.1705997100946)) ;
#111186=CARTESIAN_POINT('Ctrl Pts',(58.8112955195643,246.609118067985,22.1456576155755)) ;
#111187=CARTESIAN_POINT('Ctrl Pts',(58.8118283227689,246.614914135414,22.1362544222591)) ;
#111188=CARTESIAN_POINT('Ctrl Pts',(58.8128950891015,246.626842337563,22.1173239494713)) ;
#111189=CARTESIAN_POINT('Ctrl Pts',(58.8134287493444,246.632978910035,22.1078002405373)) ;
#111190=CARTESIAN_POINT('Ctrl Pts',(58.8148631424279,246.649915568187,22.0820909794099)) ;
#111191=CARTESIAN_POINT('Ctrl Pts',(58.8157524563631,246.660901737458,22.0660296083724)) ;
#111192=CARTESIAN_POINT('Ctrl Pts',(58.8219431047456,246.740550424521,21.9538260651249)) ;
#111193=CARTESIAN_POINT('Ctrl Pts',(58.8267480939625,246.818926087262,21.8649732255836)) ;
#111194=CARTESIAN_POINT('Ctrl Pts',(58.8350524953649,246.965094437661,21.7308605477397)) ;
#111195=CARTESIAN_POINT('Ctrl Pts',(58.8384609251298,247.028004390372,21.6809452436266)) ;
#111196=CARTESIAN_POINT('Ctrl Pts',(58.8433364277247,247.118290947778,21.6193014914828)) ;
#111197=CARTESIAN_POINT('Ctrl Pts',(58.8446557688708,247.142765264961,21.6035096613941)) ;
#111198=CARTESIAN_POINT('Ctrl Pts',(58.8468850118474,247.184062219823,21.5783610591849)) ;
#111199=CARTESIAN_POINT('Ctrl Pts',(58.8477815852708,247.200657365204,21.5686422360755)) ;
#111200=CARTESIAN_POINT('Ctrl Pts',(58.84959117711,247.23409518255,21.5498240160585)) ;
#111201=CARTESIAN_POINT('Ctrl Pts',(58.8505039623618,247.250933810155,21.5407233505481)) ;
#111202=CARTESIAN_POINT('Ctrl Pts',(58.8528072779376,247.293333256262,21.5187368650762)) ;
#111203=CARTESIAN_POINT('Ctrl Pts',(58.8542100993148,247.319074435748,21.5062136834201)) ;
#111204=CARTESIAN_POINT('Ctrl Pts',(58.8618230108034,247.458302993651,21.4428306180321)) ;
#111205=CARTESIAN_POINT('Ctrl Pts',(58.8684340781813,247.576848577834,21.4040550390575)) ;
#111206=CARTESIAN_POINT('Ctrl Pts',(58.8791490750161,247.773930296575,21.3630573987211)) ;
#111207=CARTESIAN_POINT('Ctrl Pts',(58.8832253930222,247.850286809356,21.3525842887454)) ;
#111208=CARTESIAN_POINT('Ctrl Pts',(58.8880217651646,247.94548325457,21.3461483892609)) ;
#111209=CARTESIAN_POINT('Ctrl Pts',(58.8889357985629,247.963889822747,21.3452083120157)) ;
#111210=CARTESIAN_POINT('Ctrl Pts',(58.8903767283326,247.993419333748,21.344187633411)) ;
#111211=CARTESIAN_POINT('Ctrl Pts',(58.8909132960796,248.004533747088,21.3439140306238)) ;
#111212=CARTESIAN_POINT('Ctrl Pts',(58.8919801750569,248.026897197378,21.3435858951377)) ;
#111213=CARTESIAN_POINT('Ctrl Pts',(58.8925103329082,248.038145668024,21.3435339741781)) ;
#111214=CARTESIAN_POINT('Ctrl Pts',(58.8939235311602,248.068457642554,21.3436989103481)) ;
#111215=CARTESIAN_POINT('Ctrl Pts',(58.8947957265094,248.087518735271,21.3441275581854)) ;
#111216=CARTESIAN_POINT('Ctrl Pts',(58.9002313698804,248.208099244399,21.3488965723468)) ;
#111217=CARTESIAN_POINT('Ctrl Pts',(58.9044247550774,248.309064077088,21.3621276568549)) ;
#111218=CARTESIAN_POINT('Ctrl Pts',(58.9128581300875,248.506412010373,21.4064886287213)) ;
#111219=CARTESIAN_POINT('Ctrl Pts',(58.9170850366825,248.602416382107,21.4373511458664)) ;
#111220=CARTESIAN_POINT('Ctrl Pts',(58.922825496935,248.720511232688,21.4874123225659)) ;
#111221=CARTESIAN_POINT('Ctrl Pts',(58.9240809350991,248.745680878951,21.4988233492552)) ;
#111222=CARTESIAN_POINT('Ctrl Pts',(58.926233468294,248.787629872405,21.5191051086089)) ;
#111223=CARTESIAN_POINT('Ctrl Pts',(58.9271192659513,248.804561618889,21.5276485216295)) ;
#111224=CARTESIAN_POINT('Ctrl Pts',(58.9289335319453,248.838549624449,21.5455273973439)) ;
#111225=CARTESIAN_POINT('Ctrl Pts',(58.9298623735548,248.855595657085,21.554875988622)) ;
#111226=CARTESIAN_POINT('Ctrl Pts',(58.9322637473162,248.898746729296,21.5795263875509)) ;
#111227=CARTESIAN_POINT('Ctrl Pts',(58.9337508581201,248.924606547087,21.5952416012535)) ;
#111228=CARTESIAN_POINT('Ctrl Pts',(58.9405909841939,249.039693264303,21.6695151362722)) ;
#111229=CARTESIAN_POINT('Ctrl Pts',(58.946221265251,249.123624540158,21.7358004508164)) ;
#111230=CARTESIAN_POINT('Ctrl Pts',(58.9566921257936,249.265621064996,21.8717847574258)) ;
#111231=CARTESIAN_POINT('Ctrl Pts',(58.9614940015473,249.325458123753,21.9390957679159)) ;
#111232=CARTESIAN_POINT('Ctrl Pts',(58.9669862199653,249.391135525068,22.0261519612688)) ;
#111233=CARTESIAN_POINT('Ctrl Pts',(58.967936545685,249.40239475477,22.0416194331383)) ;
#111234=CARTESIAN_POINT('Ctrl Pts',(58.9694203489835,249.419858301762,22.0664933944996)) ;
#111235=CARTESIAN_POINT('Ctrl Pts',(58.9699644587535,249.426236415168,22.0757752987595)) ;
#111236=CARTESIAN_POINT('Ctrl Pts',(58.9710324195051,249.438717222206,22.0943359539026)) ;
#111237=CARTESIAN_POINT('Ctrl Pts',(58.9715563898702,249.444822179253,22.1036124282152)) ;
#111238=CARTESIAN_POINT('Ctrl Pts',(58.9729320575894,249.460779244435,22.1283914479827)) ;
#111239=CARTESIAN_POINT('Ctrl Pts',(58.9737739021991,249.470469876354,22.1439966904043)) ;
#111240=CARTESIAN_POINT('Ctrl Pts',(58.9794742523339,249.535316435537,22.2523528520838)) ;
#111241=CARTESIAN_POINT('Ctrl Pts',(58.9839071642455,249.58167315091,22.3500863143635)) ;
#111242=CARTESIAN_POINT('Ctrl Pts',(58.9924770014192,249.651419951054,22.5432776526206)) ;
#111243=CARTESIAN_POINT('Ctrl Pts',(58.9965868135225,249.676463579344,22.6376572512019)) ;
#111244=CARTESIAN_POINT('Ctrl Pts',(59.0021600130385,249.697771279016,22.7600966090702)) ;
#111245=CARTESIAN_POINT('Ctrl Pts',(59.0033807261859,249.701735556985,22.786628200569)) ;
#111246=CARTESIAN_POINT('Ctrl Pts',(59.0054920409605,249.70739697299,22.8319242948974)) ;
#111247=CARTESIAN_POINT('Ctrl Pts',(59.0063724087197,249.709417253397,22.8506434567142)) ;
#111248=CARTESIAN_POINT('Ctrl Pts',(59.008191851812,249.712901249862,22.8889593358785)) ;
#111249=CARTESIAN_POINT('Ctrl Pts',(59.0091316703644,249.71433654715,22.908555651142)) ;
#111250=CARTESIAN_POINT('Ctrl Pts',(59.0115994151221,249.717168420724,22.9594836213597)) ;
#111251=CARTESIAN_POINT('Ctrl Pts',(59.0131435349899,249.718031200923,22.9908363139679)) ;
#111252=CARTESIAN_POINT('Ctrl Pts',(59.0196052657794,249.717964004018,23.1199459778461)) ;
#111253=CARTESIAN_POINT('Ctrl Pts',(59.024745600192,249.709370144375,23.2174968252151)) ;
#111254=CARTESIAN_POINT('Ctrl Pts',(59.0350639591994,249.675580179381,23.408402413195)) ;
#111255=CARTESIAN_POINT('Ctrl Pts',(59.040217835334,249.65071716102,23.5014598733502)) ;
#111256=CARTESIAN_POINT('Ctrl Pts',(59.0460433831368,249.611411359966,23.610151451488)) ;
#111257=CARTESIAN_POINT('Ctrl Pts',(59.04700933739,249.604486250839,23.6283087232919)) ;
#111258=CARTESIAN_POINT('Ctrl Pts',(59.0485115797545,249.593028602881,23.6568506833149)) ;
#111259=CARTESIAN_POINT('Ctrl Pts',(59.0490589241114,249.588703800771,23.6673164053325)) ;
#111260=CARTESIAN_POINT('Ctrl Pts',(59.0501276907253,249.579949729371,23.6879075053629)) ;
#111261=CARTESIAN_POINT('Ctrl Pts',(59.050649342149,249.57552575876,23.6980344042429)) ;
#111262=CARTESIAN_POINT('Ctrl Pts',(59.0520106772798,249.563592389382,23.7246315747849)) ;
#111263=CARTESIAN_POINT('Ctrl Pts',(59.0528408818623,249.555915767636,23.7410257122566)) ;
#111264=CARTESIAN_POINT('Ctrl Pts',(59.0546844514362,249.538015911516,23.7776952715522)) ;
#111265=CARTESIAN_POINT('Ctrl Pts',(59.055690540886,249.527643300369,23.7978940250859)) ;
#111266=CARTESIAN_POINT('Ctrl Pts',(59.0589846081115,249.49183639373,23.8642702780622)) ;
#111267=CARTESIAN_POINT('Ctrl Pts',(59.0612080670382,249.464635510417,23.9094606537765)) ;
#111268=CARTESIAN_POINT('Ctrl Pts',(59.0687421837228,249.364582981845,24.0592303900436)) ;
#111269=CARTESIAN_POINT('Ctrl Pts',(59.0739747414648,249.281985627891,24.1567514518126)) ;
#111270=CARTESIAN_POINT('Ctrl Pts',(59.0809289571639,249.168587520957,24.2633065079118)) ;
#111271=CARTESIAN_POINT('Ctrl Pts',(59.0822093487065,249.14754304456,24.2821044511304)) ;
#111272=CARTESIAN_POINT('Ctrl Pts',(59.0843038949953,249.112950355457,24.3114699540109)) ;
#111273=CARTESIAN_POINT('Ctrl Pts',(59.0851041141105,249.099696076997,24.3223759355834)) ;
#111274=CARTESIAN_POINT('Ctrl Pts',(59.0868052296141,249.071460111801,24.3448916749606)) ;
#111275=CARTESIAN_POINT('Ctrl Pts',(59.0877078081271,249.056444406092,24.3564547200788)) ;
#111276=CARTESIAN_POINT('Ctrl Pts',(59.0899474364691,249.019121589641,24.3842012663169)) ;
#111277=CARTESIAN_POINT('Ctrl Pts',(59.0912953489291,248.996605959164,24.4000938881119)) ;
#111278=CARTESIAN_POINT('Ctrl Pts',(59.0975763310836,248.89147858849,24.4704836188712)) ;
#111279=CARTESIAN_POINT('Ctrl Pts',(59.102751724479,248.804546483278,24.5181531354213)) ;
#111280=CARTESIAN_POINT('Ctrl Pts',(59.113535694934,248.618754302963,24.5996090550592)) ;
#111281=CARTESIAN_POINT('Ctrl Pts',(59.1191279591078,248.519902044397,24.6324054936291)) ;
#111282=CARTESIAN_POINT('Ctrl Pts',(59.1253051408544,248.400312364848,24.6600897694251)) ;
#111283=CARTESIAN_POINT('Ctrl Pts',(59.1262394457633,248.381906318736,24.6640256107041)) ;
#111284=CARTESIAN_POINT('Ctrl Pts',(59.1277043253735,248.352449302477,24.6698079774404)) ;
#111285=CARTESIAN_POINT('Ctrl Pts',(59.1282451036836,248.341439720121,24.6718548982652)) ;
#111286=CARTESIAN_POINT('Ctrl Pts',(59.1293124388825,248.319413677259,24.675722286849)) ;
#111287=CARTESIAN_POINT('Ctrl Pts',(59.1298389994593,248.308397897902,24.677543315478)) ;
#111288=CARTESIAN_POINT('Ctrl Pts',(59.1312304569059,248.278924256982,24.6821138564977)) ;
#111289=CARTESIAN_POINT('Ctrl Pts',(59.1320850859488,248.260436928664,24.6846656777916)) ;
#111290=CARTESIAN_POINT('Ctrl Pts',(59.1339935648034,248.218426788412,24.6897516526688)) ;
#111291=CARTESIAN_POINT('Ctrl Pts',(59.1350393274011,248.194885019713,24.6920978202689)) ;
#111292=CARTESIAN_POINT('Ctrl Pts',(59.1385387753894,248.114803847398,24.6983714843983)) ;
#111293=CARTESIAN_POINT('Ctrl Pts',(59.1409191793168,248.058116498361,24.6999323936584)) ;
#111294=CARTESIAN_POINT('Ctrl Pts',(59.1482633569917,247.882275219614,24.6958639063609)) ;
#111295=CARTESIAN_POINT('Ctrl Pts',(59.1531844219596,247.76372828289,24.680411270846)) ;
#111296=CARTESIAN_POINT('Ctrl Pts',(59.1598032730574,247.6193888287,24.6456860174553)) ;
#111297=CARTESIAN_POINT('Ctrl Pts',(59.1611280950841,247.591134131045,24.6381016937144)) ;
#111298=CARTESIAN_POINT('Ctrl Pts',(59.1633639478416,247.544634214823,24.6243068672195)) ;
#111299=CARTESIAN_POINT('Ctrl Pts',(59.164261470855,247.526271530763,24.6185136140823)) ;
#111300=CARTESIAN_POINT('Ctrl Pts',(59.1660708691775,247.489883050916,24.6063408902297)) ;
#111301=CARTESIAN_POINT('Ctrl Pts',(59.166982462753,247.471858531281,24.599966747521)) ;
#111302=CARTESIAN_POINT('Ctrl Pts',(59.1692784594062,247.427244067947,24.5833262747688)) ;
#111303=CARTESIAN_POINT('Ctrl Pts',(59.1706749877738,247.400800053489,24.5726880132938)) ;
#111304=CARTESIAN_POINT('Ctrl Pts',(59.1739768072608,247.339880550374,24.5463582163533)) ;
#111305=CARTESIAN_POINT('Ctrl Pts',(59.1758968835936,247.305654166584,24.5301686814799)) ;
#111306=CARTESIAN_POINT('Ctrl Pts',(59.1778464475999,247.272018857277,24.5128439810119)) ;
#111307=CARTESIAN_POINT('Ctrl Pts',(59.2757724421406,247.272018954284,24.5128440309779)) ;
#111308=CARTESIAN_POINT('Ctrl Pts',(59.2756832338205,247.273710551664,24.5137153300333)) ;
#111309=CARTESIAN_POINT('Ctrl Pts',(59.2755941944142,247.275403640655,24.5145837561406)) ;
#111310=CARTESIAN_POINT('Ctrl Pts',(59.274664186804,247.293136301171,24.5236411934761)) ;
#111311=CARTESIAN_POINT('Ctrl Pts',(59.2738379793636,247.309305809266,24.5315746064805)) ;
#111312=CARTESIAN_POINT('Ctrl Pts',(59.2691900068813,247.40235556953,24.5753839694454)) ;
#111313=CARTESIAN_POINT('Ctrl Pts',(59.2656309187946,247.481747968796,24.6056509131867)) ;
#111314=CARTESIAN_POINT('Ctrl Pts',(59.2572898826209,247.673398463464,24.6625063832365)) ;
#111315=CARTESIAN_POINT('Ctrl Pts',(59.2525282212603,247.786773605299,24.6837953462717)) ;
#111316=CARTESIAN_POINT('Ctrl Pts',(59.2460817644186,247.93100929316,24.6957723084332)) ;
#111317=CARTESIAN_POINT('Ctrl Pts',(59.2447383994796,247.960650548587,24.6974431363461)) ;
#111318=CARTESIAN_POINT('Ctrl Pts',(59.2424802275104,248.009642506877,24.6989022418924)) ;
#111319=CARTESIAN_POINT('Ctrl Pts',(59.2415795418324,248.028973428159,24.6991437044648)) ;
#111320=CARTESIAN_POINT('Ctrl Pts',(59.239770799108,248.067346942264,24.6989598424482)) ;
#111321=CARTESIAN_POINT('Ctrl Pts',(59.2388631858678,248.086386687892,24.6985443826624)) ;
#111322=CARTESIAN_POINT('Ctrl Pts',(59.2365913380461,248.133491807594,24.6967138361549)) ;
#111323=CARTESIAN_POINT('Ctrl Pts',(59.2352155180496,248.161535854383,24.6949176253331)) ;
#111324=CARTESIAN_POINT('Ctrl Pts',(59.2286621040817,248.292853503695,24.6831888805836)) ;
#111325=CARTESIAN_POINT('Ctrl Pts',(59.2232167922381,248.395095754938,24.6643962503533)) ;
#111326=CARTESIAN_POINT('Ctrl Pts',(59.2125418273794,248.588182566326,24.6100354308629)) ;
#111327=CARTESIAN_POINT('Ctrl Pts',(59.2073467257661,248.678984786095,24.5757553602442)) ;
#111328=CARTESIAN_POINT('Ctrl Pts',(59.2014859311529,248.783818635691,24.5254313073959)) ;
#111329=CARTESIAN_POINT('Ctrl Pts',(59.2005212819831,248.801166668533,24.5167301580052)) ;
#111330=CARTESIAN_POINT('Ctrl Pts',(59.1990206350808,248.828386947691,24.5024810728117)) ;
#111331=CARTESIAN_POINT('Ctrl Pts',(59.1984736158019,248.838360323534,24.4971310293533)) ;
#111332=CARTESIAN_POINT('Ctrl Pts',(59.1974051062263,248.85796506062,24.4863575446352)) ;
#111333=CARTESIAN_POINT('Ctrl Pts',(59.1968833943735,248.867598392539,24.4809390806193)) ;
#111334=CARTESIAN_POINT('Ctrl Pts',(59.1955213675278,248.892877620234,24.4663895831641)) ;
#111335=CARTESIAN_POINT('Ctrl Pts',(59.1946905523746,248.908430773549,24.4570994443033)) ;
#111336=CARTESIAN_POINT('Ctrl Pts',(59.1928453212638,248.943151769816,24.4355895184086)) ;
#111337=CARTESIAN_POINT('Ctrl Pts',(59.1918382021674,248.962228043646,24.4232283424403)) ;
#111338=CARTESIAN_POINT('Ctrl Pts',(59.1885387492599,249.024780274094,24.3808660889052)) ;
#111339=CARTESIAN_POINT('Ctrl Pts',(59.1863111621762,249.067091650836,24.3491992774067)) ;
#111340=CARTESIAN_POINT('Ctrl Pts',(59.1787824063012,249.205946775922,24.2346648135798)) ;
#111341=CARTESIAN_POINT('Ctrl Pts',(59.1735582698871,249.294527689775,24.1428561113039)) ;
#111342=CARTESIAN_POINT('Ctrl Pts',(59.1666132026627,249.389067246547,24.0195064469067)) ;
#111343=CARTESIAN_POINT('Ctrl Pts',(59.1653315961221,249.405678283071,23.9966610335597)) ;
#111344=CARTESIAN_POINT('Ctrl Pts',(59.1632357144701,249.431445739271,23.9592735358202)) ;
#111345=CARTESIAN_POINT('Ctrl Pts',(59.1624354163397,249.440969454907,23.944990764425)) ;
#111346=CARTESIAN_POINT('Ctrl Pts',(59.1607346766371,249.460537674307,23.9146454260799)) ;
#111347=CARTESIAN_POINT('Ctrl Pts',(59.1598325646368,249.470532608402,23.8985538968733)) ;
#111348=CARTESIAN_POINT('Ctrl Pts',(59.1575952925211,249.494374606878,23.8586780385084)) ;
#111349=CARTESIAN_POINT('Ctrl Pts',(59.1562493168796,249.507912701337,23.8347161732236)) ;
#111350=CARTESIAN_POINT('Ctrl Pts',(59.150008424147,249.56704370909,23.7237703359854)) ;
#111351=CARTESIAN_POINT('Ctrl Pts',(59.1448752581481,249.605529245702,23.6332296458638)) ;
#111352=CARTESIAN_POINT('Ctrl Pts',(59.1340771840239,249.668321215754,23.4400090897544)) ;
#111353=CARTESIAN_POINT('Ctrl Pts',(59.1284249762466,249.69132651387,23.3373348111415)) ;
#111354=CARTESIAN_POINT('Ctrl Pts',(59.1222023406101,249.706946259922,23.2146301974013)) ;
#111355=CARTESIAN_POINT('Ctrl Pts',(59.1212742391056,249.70899744145,23.1960407298871)) ;
#111356=CARTESIAN_POINT('Ctrl Pts',(59.1198167510851,249.711776892762,23.1662969678575)) ;
#111357=CARTESIAN_POINT('Ctrl Pts',(59.119277323937,249.712705220842,23.1551633495173)) ;
#111358=CARTESIAN_POINT('Ctrl Pts',(59.1182103668189,249.714340401072,23.132864552665)) ;
#111359=CARTESIAN_POINT('Ctrl Pts',(59.1176828777974,249.715046930052,23.1216999164919)) ;
#111360=CARTESIAN_POINT('Ctrl Pts',(59.1162855029825,249.716639866945,23.0917838042115)) ;
#111361=CARTESIAN_POINT('Ctrl Pts',(59.1154260441635,249.717323349405,23.0730227318097)) ;
#111362=CARTESIAN_POINT('Ctrl Pts',(59.1106028756525,249.719423330873,22.9660616467604)) ;
#111363=CARTESIAN_POINT('Ctrl Pts',(59.1069180968881,249.714197124594,22.877862799474)) ;
#111364=CARTESIAN_POINT('Ctrl Pts',(59.0986812719752,249.687015575204,22.6821873776594)) ;
#111365=CARTESIAN_POINT('Ctrl Pts',(59.0941397554922,249.661423920133,22.5756291101106)) ;
#111366=CARTESIAN_POINT('Ctrl Pts',(59.0879345999278,249.615792645264,22.4438554301119)) ;
#111367=CARTESIAN_POINT('Ctrl Pts',(59.0865722535898,249.60516951322,22.4156580422304)) ;
#111368=CARTESIAN_POINT('Ctrl Pts',(59.0842910679346,249.586462163637,22.369786284481)) ;
#111369=CARTESIAN_POINT('Ctrl Pts',(59.0833869848968,249.578819712629,22.3519387959534)) ;
#111370=CARTESIAN_POINT('Ctrl Pts',(59.0815782390122,249.563097403902,22.3169149055017)) ;
#111371=CARTESIAN_POINT('Ctrl Pts',(59.0806741784275,249.555032355823,22.2997350253682)) ;
#111372=CARTESIAN_POINT('Ctrl Pts',(59.0784245944884,249.534471831554,22.2578021567064)) ;
#111373=CARTESIAN_POINT('Ctrl Pts',(59.0770679827655,249.521651151157,22.2332156341506)) ;
#111374=CARTESIAN_POINT('Ctrl Pts',(59.0701848029926,249.454545247717,22.1119531686992)) ;
#111375=CARTESIAN_POINT('Ctrl Pts',(59.0643456032795,249.391385998898,22.0205188670627)) ;
#111376=CARTESIAN_POINT('Ctrl Pts',(59.0536820571112,249.26185125817,21.8678194649851)) ;
#111377=CARTESIAN_POINT('Ctrl Pts',(59.0489049680732,249.198660974826,21.8043742735574)) ;
#111378=CARTESIAN_POINT('Ctrl Pts',(59.0433791905355,249.115472558587,21.733230219853)) ;
#111379=CARTESIAN_POINT('Ctrl Pts',(59.0423809018738,249.099998770894,21.7204699080264)) ;
#111380=CARTESIAN_POINT('Ctrl Pts',(59.0408406350502,249.075336421302,21.7008645362373)) ;
#111381=CARTESIAN_POINT('Ctrl Pts',(59.0402867037317,249.066300565406,21.6938312036526)) ;
#111382=CARTESIAN_POINT('Ctrl Pts',(59.0392159284342,249.048484937863,21.6802544575572)) ;
#111383=CARTESIAN_POINT('Ctrl Pts',(59.0386986353898,249.039711863784,21.6737035124262)) ;
#111384=CARTESIAN_POINT('Ctrl Pts',(59.0373644982815,249.016675734297,21.6568508919402)) ;
#111385=CARTESIAN_POINT('Ctrl Pts',(59.0365564353191,249.002313280192,21.6466865915394)) ;
#111386=CARTESIAN_POINT('Ctrl Pts',(59.0347711755006,248.969757747503,21.6244072801883)) ;
#111387=CARTESIAN_POINT('Ctrl Pts',(59.0338005635506,248.951482329002,21.6124179650065)) ;
#111388=CARTESIAN_POINT('Ctrl Pts',(59.0306825977539,248.891184782886,21.5745248579657)) ;
#111389=CARTESIAN_POINT('Ctrl Pts',(59.0285926323636,248.848251720638,21.5501169208241)) ;
#111390=CARTESIAN_POINT('Ctrl Pts',(59.0208652754726,248.684121063009,21.4661619896179)) ;
#111391=CARTESIAN_POINT('Ctrl Pts',(59.0153460338213,248.556968156538,21.4194199658274)) ;
#111392=CARTESIAN_POINT('Ctrl Pts',(59.0080817135993,248.39918600657,21.3821874172139)) ;
#111393=CARTESIAN_POINT('Ctrl Pts',(59.0068479444681,248.372637394238,21.376598625297)) ;
#111394=CARTESIAN_POINT('Ctrl Pts',(59.0047299598419,248.327590647772,21.3682509753661)) ;
#111395=CARTESIAN_POINT('Ctrl Pts',(59.0038565676469,248.309160398292,21.3651532048937)) ;
#111396=CARTESIAN_POINT('Ctrl Pts',(59.0020510631478,248.27138542847,21.359451116319)) ;
#111397=CARTESIAN_POINT('Ctrl Pts',(59.0011182035658,248.252039363202,21.3568752238686)) ;
#111398=CARTESIAN_POINT('Ctrl Pts',(58.9986919659079,248.202183982957,21.3511203296651)) ;
#111399=CARTESIAN_POINT('Ctrl Pts',(58.9971834057496,248.171625359811,21.3484395524482)) ;
#111400=CARTESIAN_POINT('Ctrl Pts',(58.9937842867575,248.103738671579,21.3443556846649)) ;
#111401=CARTESIAN_POINT('Ctrl Pts',(58.9918828540747,248.066403104802,21.3433585082654)) ;
#111402=CARTESIAN_POINT('Ctrl Pts',(58.9852501600673,247.938082526444,21.3442150068167)) ;
#111403=CARTESIAN_POINT('Ctrl Pts',(58.9803795988204,247.847302454304,21.3522226315655)) ;
#111404=CARTESIAN_POINT('Ctrl Pts',(58.9717395520393,247.687052260192,21.3796102814224)) ;
#111405=CARTESIAN_POINT('Ctrl Pts',(58.9679687205315,247.617317290485,21.3961779373445)) ;
#111406=CARTESIAN_POINT('Ctrl Pts',(58.9635355362364,247.532637767708,21.4221183368638)) ;
#111407=CARTESIAN_POINT('Ctrl Pts',(58.9626976219862,247.516500882964,21.4273304905638)) ;
#111408=CARTESIAN_POINT('Ctrl Pts',(58.9613981210444,247.491204560043,21.4359267556684)) ;
#111409=CARTESIAN_POINT('Ctrl Pts',(58.9609277845549,247.481991193062,21.4391476095167)) ;
#111410=CARTESIAN_POINT('Ctrl Pts',(58.9599251710927,247.462209461428,21.4462573199981)) ;
#111411=CARTESIAN_POINT('Ctrl Pts',(58.9593944861244,247.451651061834,21.450172554115)) ;
#111412=CARTESIAN_POINT('Ctrl Pts',(58.9579777970654,247.423264218973,21.4610252073203)) ;
#111413=CARTESIAN_POINT('Ctrl Pts',(58.9571027345452,247.405513312165,21.4681618777725)) ;
#111414=CARTESIAN_POINT('Ctrl Pts',(58.955139455352,247.365349113441,21.4851133457979)) ;
#111415=CARTESIAN_POINT('Ctrl Pts',(58.9540600469222,247.343020455939,21.4951180248594)) ;
#111416=CARTESIAN_POINT('Ctrl Pts',(58.9503786464123,247.266519163842,21.5314250365684)) ;
#111417=CARTESIAN_POINT('Ctrl Pts',(58.9478580874344,247.21354743314,21.5601532427633)) ;
#111418=CARTESIAN_POINT('Ctrl Pts',(58.9406477027788,247.066241987889,21.6506220243604)) ;
#111419=CARTESIAN_POINT('Ctrl Pts',(58.9359784797362,246.976434506998,21.7190923748397)) ;
#111420=CARTESIAN_POINT('Ctrl Pts',(58.9296327427801,246.872337684337,21.8164617003937)) ;
#111421=CARTESIAN_POINT('Ctrl Pts',(58.9282803263903,246.851055079706,21.8374630033313)) ;
#111422=CARTESIAN_POINT('Ctrl Pts',(58.9260111853406,246.816926029838,21.8729903431372)) ;
#111423=CARTESIAN_POINT('Ctrl Pts',(58.9251088835541,246.803749775198,21.887190683996)) ;
#111424=CARTESIAN_POINT('Ctrl Pts',(58.9233001766887,246.778134663553,21.9157737630462)) ;
#111425=CARTESIAN_POINT('Ctrl Pts',(58.9223942915969,246.765688580717,21.9301461410217)) ;
#111426=CARTESIAN_POINT('Ctrl Pts',(58.9201332532231,246.735575535026,21.9661381066379)) ;
#111427=CARTESIAN_POINT('Ctrl Pts',(58.9187667565292,246.718199287022,21.9879925712087)) ;
#111428=CARTESIAN_POINT('Ctrl Pts',(58.9120650556819,246.63691815688,22.0956294463276)) ;
#111429=CARTESIAN_POINT('Ctrl Pts',(58.9064422590297,246.5807775837,22.1869479321452)) ;
#111430=CARTESIAN_POINT('Ctrl Pts',(58.8957605556408,246.492477302808,22.3671194538856)) ;
#111431=CARTESIAN_POINT('Ctrl Pts',(58.8907432286155,246.458358890063,22.4545748597694)) ;
#111432=CARTESIAN_POINT('Ctrl Pts',(58.8850297653321,246.426151035413,22.5632103880907)) ;
#111433=CARTESIAN_POINT('Ctrl Pts',(58.8840553706572,246.420910909986,22.5820925991769)) ;
#111434=CARTESIAN_POINT('Ctrl Pts',(58.8825432344746,246.413158080223,22.6120566921717)) ;
#111435=CARTESIAN_POINT('Ctrl Pts',(58.8819942043579,246.410425208202,22.6230792976749)) ;
#111436=CARTESIAN_POINT('Ctrl Pts',(58.8809251145403,246.405261114147,22.6448519498689)) ;
#111437=CARTESIAN_POINT('Ctrl Pts',(58.8804047660875,246.402823512767,22.6555997660341)) ;
#111438=CARTESIAN_POINT('Ctrl Pts',(58.8790512412998,246.396693094635,22.6839206939715)) ;
#111439=CARTESIAN_POINT('Ctrl Pts',(58.8782273446952,246.393176093099,22.7015308686017)) ;
#111440=CARTESIAN_POINT('Ctrl Pts',(58.8736452966569,246.374921429963,22.8012446361361)) ;
#111441=CARTESIAN_POINT('Ctrl Pts',(58.8701411218086,246.36603908736,22.8843078139307)) ;
#111442=CARTESIAN_POINT('Ctrl Pts',(58.8617767426315,246.359633400343,23.0846081531142)) ;
#111443=CARTESIAN_POINT('Ctrl Pts',(58.8569414150446,246.368132146755,23.201592323637)) ;
#111444=CARTESIAN_POINT('Ctrl Pts',(58.8504151549209,246.393920590317,23.3457654695649)) ;
#111445=CARTESIAN_POINT('Ctrl Pts',(58.8490799687286,246.399878087681,23.3746547676323)) ;
#111446=CARTESIAN_POINT('Ctrl Pts',(58.8468316993007,246.410987738129,23.4221602807902)) ;
#111447=CARTESIAN_POINT('Ctrl Pts',(58.8459324668906,246.415705477713,23.4408717399387)) ;
#111448=CARTESIAN_POINT('Ctrl Pts',(58.8441236294452,246.42572615438,23.4779085854282)) ;
#111449=CARTESIAN_POINT('Ctrl Pts',(58.8432143983577,246.431020989747,23.4962331635209)) ;
#111450=CARTESIAN_POINT('Ctrl Pts',(58.8409324641281,246.444935497676,23.5414813961833)) ;
#111451=CARTESIAN_POINT('Ctrl Pts',(58.8395479485843,246.453925187186,23.5682843485361)) ;
#111452=CARTESIAN_POINT('Ctrl Pts',(58.8328216666303,246.500165118509,23.695402307595)) ;
#111453=CARTESIAN_POINT('Ctrl Pts',(58.8271933792132,246.546274434922,23.7922167174662)) ;
#111454=CARTESIAN_POINT('Ctrl Pts',(58.8165664935499,246.648902277645,23.963410117423)) ;
#111455=CARTESIAN_POINT('Ctrl Pts',(58.8116095845956,246.703024063899,24.0387739582984)) ;
#111456=CARTESIAN_POINT('Ctrl Pts',(58.8059404796308,246.775901722118,24.1243255587703)) ;
#111457=CARTESIAN_POINT('Ctrl Pts',(58.8049577719186,246.788976536466,24.1391361816344)) ;
#111458=CARTESIAN_POINT('Ctrl Pts',(58.8034358438087,246.809997031716,24.1621162160562)) ;
#111459=CARTESIAN_POINT('Ctrl Pts',(58.8028851051076,246.817769270327,24.1704411825542)) ;
#111460=CARTESIAN_POINT('Ctrl Pts',(58.8018154691542,246.833210207075,24.1866462238561)) ;
#111461=CARTESIAN_POINT('Ctrl Pts',(58.8012962267056,246.840872689327,24.1945312255709)) ;
#111462=CARTESIAN_POINT('Ctrl Pts',(58.7999496706984,246.861160494751,24.2150016827531)) ;
#111463=CARTESIAN_POINT('Ctrl Pts',(58.7991314570207,246.873910179236,24.2274625625539)) ;
#111464=CARTESIAN_POINT('Ctrl Pts',(58.7947027895651,246.945032188495,24.2947909260585)) ;
#111465=CARTESIAN_POINT('Ctrl Pts',(58.7913266365165,247.007082701722,24.3456309901094)) ;
#111466=CARTESIAN_POINT('Ctrl Pts',(58.7847244126569,247.136185351128,24.4367907842065)) ;
#111467=CARTESIAN_POINT('Ctrl Pts',(58.7815055650463,247.202845155603,24.4772143680056)) ;
#111468=CARTESIAN_POINT('Ctrl Pts',(58.7781769759756,247.272019165218,24.5128441396244)) ;
#111469=CARTESIAN_POINT('Origin',(61.8645744874958,248.040265107786,23.0213203435596)) ;
#111470=CARTESIAN_POINT('',(58.1788076829103,247.272018954284,24.5128440309778)) ;
#111471=CARTESIAN_POINT('',(58.2783798877068,247.272019130299,24.5128441216388)) ;
#111472=CARTESIAN_POINT('',(61.8645744874958,247.272018954284,24.5128440309778)) ;
#111473=CARTESIAN_POINT('',(58.5159557280534,249.718014455466,23.019840864003)) ;
#111474=CARTESIAN_POINT('Ctrl Pts',(58.5159557280534,249.718014455466,23.019840864003)) ;
#111475=CARTESIAN_POINT('Ctrl Pts',(58.512319144992,249.717946765379,22.9430794117974)) ;
#111476=CARTESIAN_POINT('Ctrl Pts',(58.5086825619307,249.712607036384,22.8665495704283)) ;
#111477=CARTESIAN_POINT('Ctrl Pts',(58.5050459788693,249.702113747406,22.7908769416287)) ;
#111478=CARTESIAN_POINT('Ctrl Pts',(58.501409395808,249.691620458428,22.7152043128292)) ;
#111479=CARTESIAN_POINT('Ctrl Pts',(58.4977728127466,249.675973792176,22.6403886898807)) ;
#111480=CARTESIAN_POINT('Ctrl Pts',(58.4941362296853,249.655340419636,22.5670332101811)) ;
#111481=CARTESIAN_POINT('Ctrl Pts',(58.4912273357581,249.638835835232,22.5083563407627)) ;
#111482=CARTESIAN_POINT('Ctrl Pts',(58.488318441831,249.619095809122,22.4504605153754)) ;
#111483=CARTESIAN_POINT('Ctrl Pts',(58.4854095479039,249.596212549723,22.3937276249675)) ;
#111484=CARTESIAN_POINT('Ctrl Pts',(58.4824763077287,249.573137766837,22.3365199035561)) ;
#111485=CARTESIAN_POINT('Ctrl Pts',(58.4795430675535,249.54686695187,22.2804952007317)) ;
#111486=CARTESIAN_POINT('Ctrl Pts',(58.4766098273783,249.517546749281,22.2260317077794)) ;
#111487=CARTESIAN_POINT('Ctrl Pts',(58.4737088759363,249.488549299736,22.1721677419993)) ;
#111488=CARTESIAN_POINT('Ctrl Pts',(58.4708079244942,249.456569502694,22.1198312496985)) ;
#111489=CARTESIAN_POINT('Ctrl Pts',(58.4679069730521,249.421797367442,22.0693677827505)) ;
#111490=CARTESIAN_POINT('Ctrl Pts',(58.4650077825223,249.387046339292,22.0189349477316)) ;
#111491=CARTESIAN_POINT('Ctrl Pts',(58.4621085919926,249.349506622877,21.9703733030639)) ;
#111492=CARTESIAN_POINT('Ctrl Pts',(58.4592094014628,249.309412361891,21.9240007411198)) ;
#111493=CARTESIAN_POINT('Ctrl Pts',(58.4563109008991,249.269327642768,21.8776392151865)) ;
#111494=CARTESIAN_POINT('Ctrl Pts',(58.4534124003355,249.226689919712,21.8334661235975)) ;
#111495=CARTESIAN_POINT('Ctrl Pts',(58.4505138997719,249.18177324594,21.7917658579719)) ;
#111496=CARTESIAN_POINT('Ctrl Pts',(58.4475553900992,249.135926639771,21.749202250859)) ;
#111497=CARTESIAN_POINT('Ctrl Pts',(58.4445968804265,249.087706025917,21.7092154260372)) ;
#111498=CARTESIAN_POINT('Ctrl Pts',(58.4416383707538,249.037440157736,21.6720661116754)) ;
#111499=CARTESIAN_POINT('Ctrl Pts',(58.4387362096991,248.988131667599,21.6356243537374)) ;
#111500=CARTESIAN_POINT('Ctrl Pts',(58.4358340486445,248.936855629865,21.6019131867214)) ;
#111501=CARTESIAN_POINT('Ctrl Pts',(58.4329318875898,248.88395137375,21.5711346495455)) ;
#111502=CARTESIAN_POINT('Ctrl Pts',(58.4299452036081,248.829506327,21.5394597141334)) ;
#111503=CARTESIAN_POINT('Ctrl Pts',(58.4269585196264,248.773337245491,21.5108911838589)) ;
#111504=CARTESIAN_POINT('Ctrl Pts',(58.4239718356447,248.715838132977,21.4855970123135)) ;
#111505=CARTESIAN_POINT('Ctrl Pts',(58.4209851516631,248.658339020463,21.460302840768)) ;
#111506=CARTESIAN_POINT('Ctrl Pts',(58.4179984676814,248.599510445876,21.4382831667924)) ;
#111507=CARTESIAN_POINT('Ctrl Pts',(58.4150117836997,248.539762635379,21.4196501894927)) ;
#111508=CARTESIAN_POINT('Ctrl Pts',(58.4121032756731,248.481578713856,21.401504927266)) ;
#111509=CARTESIAN_POINT('Ctrl Pts',(58.4091947676465,248.422286197173,21.3864972799856)) ;
#111510=CARTESIAN_POINT('Ctrl Pts',(58.4062862596199,248.36225544961,21.3747580816722)) ;
#111511=CARTESIAN_POINT('Ctrl Pts',(58.4033529712071,248.301713242189,21.3629188658018)) ;
#111512=CARTESIAN_POINT('Ctrl Pts',(58.4004196827944,248.240420639795,21.3544042929628)) ;
#111513=CARTESIAN_POINT('Ctrl Pts',(58.3974863943817,248.178774750602,21.3492975741731)) ;
#111514=CARTESIAN_POINT('Ctrl Pts',(58.3945858116232,248.117816202324,21.3442477944074)) ;
#111515=CARTESIAN_POINT('Ctrl Pts',(58.3916852288648,248.056512725529,21.3425303093672)) ;
#111516=CARTESIAN_POINT('Ctrl Pts',(58.3887846461064,247.99525752739,21.3441741423574)) ;
#111517=CARTESIAN_POINT('Ctrl Pts',(58.3858858168575,247.934039360282,21.3458169815898)) ;
#111518=CARTESIAN_POINT('Ctrl Pts',(58.3829869876085,247.872869923269,21.3508170959372)) ;
#111519=CARTESIAN_POINT('Ctrl Pts',(58.3800881583596,247.812143285866,21.3591514301023)) ;
#111520=CARTESIAN_POINT('Ctrl Pts',(58.3771900111413,247.7514309361,21.3674838033825)) ;
#111521=CARTESIAN_POINT('Ctrl Pts',(58.3742918639229,247.69116168467,21.3791487696651)) ;
#111522=CARTESIAN_POINT('Ctrl Pts',(58.3713937167045,247.63172326158,21.3940715542227)) ;
#111523=CARTESIAN_POINT('Ctrl Pts',(58.3684348517887,247.57103957249,21.4093069789088)) ;
#111524=CARTESIAN_POINT('Ctrl Pts',(58.3654759868728,247.511222467808,21.4279381960708)) ;
#111525=CARTESIAN_POINT('Ctrl Pts',(58.3625171219569,247.452669923237,21.4498315712183)) ;
#111526=CARTESIAN_POINT('Ctrl Pts',(58.3596152908466,247.395246012293,21.4713029390971)) ;
#111527=CARTESIAN_POINT('Ctrl Pts',(58.3567134597363,247.339038791254,21.4959115382701)) ;
#111528=CARTESIAN_POINT('Ctrl Pts',(58.3538116286261,247.284402505327,21.5234829729803)) ;
#111529=CARTESIAN_POINT('Ctrl Pts',(58.3508242468074,247.228155452686,21.551867258501)) ;
#111530=CARTESIAN_POINT('Ctrl Pts',(58.3478368649888,247.173573943315,21.58339157008)) ;
#111531=CARTESIAN_POINT('Ctrl Pts',(58.3448494831701,247.121013786214,21.6178168450647)) ;
#111532=CARTESIAN_POINT('Ctrl Pts',(58.3418621013515,247.068453629112,21.6522421200494)) ;
#111533=CARTESIAN_POINT('Ctrl Pts',(58.3388747195328,247.017915251416,21.6895679561089)) ;
#111534=CARTESIAN_POINT('Ctrl Pts',(58.3358873377142,246.969716489903,21.7295112557881)) ;
#111535=CARTESIAN_POINT('Ctrl Pts',(58.3329808840848,246.922823433095,21.7683724912673)) ;
#111536=CARTESIAN_POINT('Ctrl Pts',(58.3300744304555,246.877952616534,21.8098703856135)) ;
#111537=CARTESIAN_POINT('Ctrl Pts',(58.3271679768261,246.835415446672,21.8537663376942)) ;
#111538=CARTESIAN_POINT('Ctrl Pts',(58.3242344316138,246.79248178011,21.8980714519302)) ;
#111539=CARTESIAN_POINT('Ctrl Pts',(58.3213008864014,246.751925950203,21.9448192926936)) ;
#111540=CARTESIAN_POINT('Ctrl Pts',(58.318367341189,246.714034725236,21.9937221560853)) ;
#111541=CARTESIAN_POINT('Ctrl Pts',(58.3154688347601,246.676596079769,22.0420409150172)) ;
#111542=CARTESIAN_POINT('Ctrl Pts',(58.3125703283311,246.641759057408,22.0924630850673)) ;
#111543=CARTESIAN_POINT('Ctrl Pts',(58.3096718219022,246.60976219787,22.1446753257664)) ;
#111544=CARTESIAN_POINT('Ctrl Pts',(58.3067750713524,246.577784721631,22.1968559369408)) ;
#111545=CARTESIAN_POINT('Ctrl Pts',(58.3038783208025,246.548644263484,22.25082403357)) ;
#111546=CARTESIAN_POINT('Ctrl Pts',(58.3009815702527,246.522536186484,22.3062371428449)) ;
#111547=CARTESIAN_POINT('Ctrl Pts',(58.298085500658,246.496434246855,22.3616372258537)) ;
#111548=CARTESIAN_POINT('Ctrl Pts',(58.2951894310634,246.473363491077,22.4184811847766)) ;
#111549=CARTESIAN_POINT('Ctrl Pts',(58.2922933614687,246.453472472819,22.4764036562443)) ;
#111550=CARTESIAN_POINT('Ctrl Pts',(58.2893324889904,246.433136370181,22.5356222095421)) ;
#111551=CARTESIAN_POINT('Ctrl Pts',(58.286371616512,246.41612425942,22.5959676176771)) ;
#111552=CARTESIAN_POINT('Ctrl Pts',(58.2834107440337,246.402541327335,22.6570321589531)) ;
#111553=CARTESIAN_POINT('Ctrl Pts',(58.2805109638258,246.389238654587,22.7168367434091)) ;
#111554=CARTESIAN_POINT('Ctrl Pts',(58.277611183618,246.379225004203,22.777330536764)) ;
#111555=CARTESIAN_POINT('Ctrl Pts',(58.2747114034101,246.372547084093,22.8381219375916)) ;
#111556=CARTESIAN_POINT('Ctrl Pts',(58.2717199847966,246.365658129384,22.9008344588676)) ;
#111557=CARTESIAN_POINT('Ctrl Pts',(58.268728566183,246.36231935317,22.9638631286378)) ;
#111558=CARTESIAN_POINT('Ctrl Pts',(58.2657371475694,246.362523982039,23.0267772177427)) ;
#111559=CARTESIAN_POINT('Ctrl Pts',(58.2627457289558,246.362728610907,23.0896913068475)) ;
#111560=CARTESIAN_POINT('Ctrl Pts',(58.2597543103423,246.366476538335,23.1524902311482)) ;
#111561=CARTESIAN_POINT('Ctrl Pts',(58.2567628917287,246.373702911042,23.2147512275519)) ;
#111562=CARTESIAN_POINT('Ctrl Pts',(58.2538499587604,246.380739685902,23.2753786864564)) ;
#111563=CARTESIAN_POINT('Ctrl Pts',(58.2509370257922,246.391103214285,23.3357435029581)) ;
#111564=CARTESIAN_POINT('Ctrl Pts',(58.2480240928239,246.404762219472,23.3954531606417)) ;
#111565=CARTESIAN_POINT('Ctrl Pts',(58.2451162792155,246.418397219521,23.4550578810588)) ;
#111566=CARTESIAN_POINT('Ctrl Pts',(58.2422084656071,246.435316083139,23.5140092369757)) ;
#111567=CARTESIAN_POINT('Ctrl Pts',(58.2393006519987,246.455436000457,23.5719216176783)) ;
#111568=CARTESIAN_POINT('Ctrl Pts',(58.2363957088068,246.475536056617,23.6297768308042)) ;
#111569=CARTESIAN_POINT('Ctrl Pts',(58.233490765615,246.49883073656,23.6865946235036)) ;
#111570=CARTESIAN_POINT('Ctrl Pts',(58.2305858224232,246.525186974954,23.742002876936)) ;
#111571=CARTESIAN_POINT('Ctrl Pts',(58.2276826827665,246.551526850066,23.7973767301316)) ;
#111572=CARTESIAN_POINT('Ctrl Pts',(58.2247795431098,246.580924295902,23.8513423210356)) ;
#111573=CARTESIAN_POINT('Ctrl Pts',(58.2218764034532,246.613198284203,23.9035478332288)) ;
#111574=CARTESIAN_POINT('Ctrl Pts',(58.2189740028974,246.645464055975,23.9557400545912)) ;
#111575=CARTESIAN_POINT('Ctrl Pts',(58.2160716023415,246.680604648608,24.0061726544247)) ;
#111576=CARTESIAN_POINT('Ctrl Pts',(58.2131692017857,246.718394304614,24.0545205382078)) ;
#111577=CARTESIAN_POINT('Ctrl Pts',(58.2102644853581,246.75621411359,24.1029069995403)) ;
#111578=CARTESIAN_POINT('Ctrl Pts',(58.2073597689305,246.796686898043,24.1492050171797)) ;
#111579=CARTESIAN_POINT('Ctrl Pts',(58.2044550525028,246.839545718577,24.1931215258754)) ;
#111580=CARTESIAN_POINT('Ctrl Pts',(58.2015492914808,246.882419952002,24.2370538278295)) ;
#111581=CARTESIAN_POINT('Ctrl Pts',(58.1986435304589,246.927681558917,24.2786025660187)) ;
#111582=CARTESIAN_POINT('Ctrl Pts',(58.1957377694369,246.975027895082,24.3175127456246)) ;
#111583=CARTESIAN_POINT('Ctrl Pts',(58.1928267896766,247.022459265128,24.3564928077992)) ;
#111584=CARTESIAN_POINT('Ctrl Pts',(58.1899158099164,247.071982436888,24.3928245366809)) ;
#111585=CARTESIAN_POINT('Ctrl Pts',(58.1870048301561,247.123263613894,24.426294835392)) ;
#111586=CARTESIAN_POINT('Ctrl Pts',(58.1842724477408,247.17139853678,24.4577116308227)) ;
#111587=CARTESIAN_POINT('Ctrl Pts',(58.1815400653256,247.221081789228,24.4866075846815)) ;
#111588=CARTESIAN_POINT('Ctrl Pts',(58.1788076829103,247.272018954284,24.5128440309778)) ;
#111589=CARTESIAN_POINT('Ctrl Pts',(58.515643070046,249.718014466972,23.01985397027)) ;
#111590=CARTESIAN_POINT('Ctrl Pts',(58.5179320301945,249.718062191968,23.0744584714563)) ;
#111591=CARTESIAN_POINT('Ctrl Pts',(58.5202465310105,249.715444140582,23.1290318143707)) ;
#111592=CARTESIAN_POINT('Ctrl Pts',(58.5240382880717,249.707042313032,23.2156066858572)) ;
#111593=CARTESIAN_POINT('Ctrl Pts',(58.5254717260617,249.702982624228,23.247735351128)) ;
#111594=CARTESIAN_POINT('Ctrl Pts',(58.5278030221993,249.695024000041,23.2987918396245)) ;
#111595=CARTESIAN_POINT('Ctrl Pts',(58.528683075632,249.691723312647,23.3178050577416)) ;
#111596=CARTESIAN_POINT('Ctrl Pts',(58.5304557462619,249.684499348991,23.3555428350881)) ;
#111597=CARTESIAN_POINT('Ctrl Pts',(58.5313480524487,249.680582307546,23.3742656114643)) ;
#111598=CARTESIAN_POINT('Ctrl Pts',(58.5331578527914,249.672087840024,23.4116654128546)) ;
#111599=CARTESIAN_POINT('Ctrl Pts',(58.5340753167885,249.667507723484,23.4303388451223)) ;
#111600=CARTESIAN_POINT('Ctrl Pts',(58.5364088090204,249.6551834298,23.4770970861105)) ;
#111601=CARTESIAN_POINT('Ctrl Pts',(58.5378378385315,249.647026999209,23.5050658550262)) ;
#111602=CARTESIAN_POINT('Ctrl Pts',(58.5453499516503,249.60105925046,23.6486688460366)) ;
#111603=CARTESIAN_POINT('Ctrl Pts',(58.5518124162021,249.551484034298,23.7601400907936)) ;
#111604=CARTESIAN_POINT('Ctrl Pts',(58.5612304916895,249.462507892651,23.9130178303199)) ;
#111605=CARTESIAN_POINT('Ctrl Pts',(58.5641635121313,249.432366386356,23.9593786641421)) ;
#111606=CARTESIAN_POINT('Ctrl Pts',(58.5682276679555,249.386329564592,24.0230685030165)) ;
#111607=CARTESIAN_POINT('Ctrl Pts',(58.5694197585455,249.372275163203,24.0416821363769)) ;
#111608=CARTESIAN_POINT('Ctrl Pts',(58.5715205452099,249.346406410939,24.074496895347)) ;
#111609=CARTESIAN_POINT('Ctrl Pts',(58.5724363990657,249.334737027622,24.0888073235102)) ;
#111610=CARTESIAN_POINT('Ctrl Pts',(58.5738793039246,249.315664163357,24.111423999665)) ;
#111611=CARTESIAN_POINT('Ctrl Pts',(58.5744160817446,249.308410384526,24.1198540498652)) ;
#111612=CARTESIAN_POINT('Ctrl Pts',(58.5754826946989,249.293659286898,24.1366563344218)) ;
#111613=CARTESIAN_POINT('Ctrl Pts',(58.5760123921181,249.286160623736,24.145026584935)) ;
#111614=CARTESIAN_POINT('Ctrl Pts',(58.5774227989656,249.26575057283,24.1673534557708)) ;
#111615=CARTESIAN_POINT('Ctrl Pts',(58.5782927381509,249.252684846015,24.1811672945508)) ;
#111616=CARTESIAN_POINT('Ctrl Pts',(58.583750004731,249.167961298428,24.2677453579383)) ;
#111617=CARTESIAN_POINT('Ctrl Pts',(58.5879629602787,249.09001440943,24.3340671440252)) ;
#111618=CARTESIAN_POINT('Ctrl Pts',(58.5963099657129,248.92635643896,24.4493613893714)) ;
#111619=CARTESIAN_POINT('Ctrl Pts',(58.6004280223336,248.841406858024,24.4986927361666)) ;
#111620=CARTESIAN_POINT('Ctrl Pts',(58.6060840722861,248.726708687347,24.55248353038)) ;
#111621=CARTESIAN_POINT('Ctrl Pts',(58.6073828591067,248.700469523681,24.5639789292531)) ;
#111622=CARTESIAN_POINT('Ctrl Pts',(58.6095873956141,248.656223033881,24.5820276899201)) ;
#111623=CARTESIAN_POINT('Ctrl Pts',(58.6104804836726,248.638374270672,24.5889545423018)) ;
#111624=CARTESIAN_POINT('Ctrl Pts',(58.6122912009387,248.602368152751,24.6022235655979)) ;
#111625=CARTESIAN_POINT('Ctrl Pts',(58.6132087845088,248.584212516365,24.6085619791354)) ;
#111626=CARTESIAN_POINT('Ctrl Pts',(58.6155412829522,248.538309720398,24.6237072903177)) ;
#111627=CARTESIAN_POINT('Ctrl Pts',(58.6169691536816,248.510435543522,24.6321064854137)) ;
#111628=CARTESIAN_POINT('Ctrl Pts',(58.6244183518366,248.36618946995,24.6715083441976)) ;
#111629=CARTESIAN_POINT('Ctrl Pts',(58.6308102685836,248.24695511078,24.6906373721208)) ;
#111630=CARTESIAN_POINT('Ctrl Pts',(58.6415295244695,248.045900337825,24.7010115267353)) ;
#111631=CARTESIAN_POINT('Ctrl Pts',(58.6458223555456,247.964879534078,24.6993289756702)) ;
#111632=CARTESIAN_POINT('Ctrl Pts',(58.6507810093612,247.866507964071,24.6901440500868)) ;
#111633=CARTESIAN_POINT('Ctrl Pts',(58.6516657097671,247.848750453958,24.6881995509372)) ;
#111634=CARTESIAN_POINT('Ctrl Pts',(58.6530721019866,247.820108830985,24.684599442471)) ;
#111635=CARTESIAN_POINT('Ctrl Pts',(58.6536027052168,247.809204271112,24.6831196860291)) ;
#111636=CARTESIAN_POINT('Ctrl Pts',(58.6546697822737,247.78704903131,24.6798909000274)) ;
#111637=CARTESIAN_POINT('Ctrl Pts',(58.6552058562418,247.775800125529,24.678134442542)) ;
#111638=CARTESIAN_POINT('Ctrl Pts',(58.6566547762021,247.745111478052,24.6730220498855)) ;
#111639=CARTESIAN_POINT('Ctrl Pts',(58.6575558051197,247.725711225189,24.6694374826725)) ;
#111640=CARTESIAN_POINT('Ctrl Pts',(58.6626130507342,247.615465082727,24.6470497176586)) ;
#111641=CARTESIAN_POINT('Ctrl Pts',(58.6664675055547,247.526232084007,24.6210778177386)) ;
#111642=CARTESIAN_POINT('Ctrl Pts',(58.672888695377,247.382377997139,24.5659190495331)) ;
#111643=CARTESIAN_POINT('Ctrl Pts',(58.6754407143328,247.326435861763,24.5408728113435)) ;
#111644=CARTESIAN_POINT('Ctrl Pts',(58.6780583779715,247.272018809212,24.512843956255)) ;
#111645=CARTESIAN_POINT('Ctrl Pts',(58.7781769759756,247.272019165218,24.5128441396244)) ;
#111646=CARTESIAN_POINT('Ctrl Pts',(58.7763091666173,247.310835570535,24.5328374819825)) ;
#111647=CARTESIAN_POINT('Ctrl Pts',(58.774407975385,247.350443695255,24.5513213682175)) ;
#111648=CARTESIAN_POINT('Ctrl Pts',(58.7711652789816,247.417460655586,24.5794597720553)) ;
#111649=CARTESIAN_POINT('Ctrl Pts',(58.7698528371765,247.444449249757,24.58997811835)) ;
#111650=CARTESIAN_POINT('Ctrl Pts',(58.7676320365219,247.489758419209,24.6062985897986)) ;
#111651=CARTESIAN_POINT('Ctrl Pts',(58.7667367847226,247.507931004924,24.6124941310397)) ;
#111652=CARTESIAN_POINT('Ctrl Pts',(58.7649272881695,247.544447029362,24.6242478918723)) ;
#111653=CARTESIAN_POINT('Ctrl Pts',(58.7640132172179,247.562787341133,24.6298063513237)) ;
#111654=CARTESIAN_POINT('Ctrl Pts',(58.761701374617,247.608887281234,24.642920093752)) ;
#111655=CARTESIAN_POINT('Ctrl Pts',(58.7602911119702,247.636752865747,24.6500776379853)) ;
#111656=CARTESIAN_POINT('Ctrl Pts',(58.7536240153106,247.767284446877,24.6800506204373)) ;
#111657=CARTESIAN_POINT('Ctrl Pts',(58.7480935357987,247.871755414129,24.6938944737568)) ;
#111658=CARTESIAN_POINT('Ctrl Pts',(58.7375092745268,248.070428162307,24.7014126090336)) ;
#111659=CARTESIAN_POINT('Ctrl Pts',(58.7324937558047,248.164171910562,24.6971093414747)) ;
#111660=CARTESIAN_POINT('Ctrl Pts',(58.7267816618943,248.276503243161,24.6824707501298)) ;
#111661=CARTESIAN_POINT('Ctrl Pts',(58.72580705598,248.295891470333,24.6795978692146)) ;
#111662=CARTESIAN_POINT('Ctrl Pts',(58.7242946691828,248.326428696776,24.674524636937)) ;
#111663=CARTESIAN_POINT('Ctrl Pts',(58.7237455939469,248.337612874061,24.6725496900193)) ;
#111664=CARTESIAN_POINT('Ctrl Pts',(58.7226764739928,248.359608509145,24.6684348796372)) ;
#111665=CARTESIAN_POINT('Ctrl Pts',(58.7221561392753,248.370420520988,24.6663017760783)) ;
#111666=CARTESIAN_POINT('Ctrl Pts',(58.7208027443307,248.398789837314,24.6604138158854)) ;
#111667=CARTESIAN_POINT('Ctrl Pts',(58.719978959852,248.416309692928,24.6564833040354)) ;
#111668=CARTESIAN_POINT('Ctrl Pts',(58.7154002734769,248.514779735428,24.6327255086645)) ;
#111669=CARTESIAN_POINT('Ctrl Pts',(58.7118988982531,248.5942339226,24.6071676261343)) ;
#111670=CARTESIAN_POINT('Ctrl Pts',(58.7035334161776,248.779933585828,24.5317643156487)) ;
#111671=CARTESIAN_POINT('Ctrl Pts',(58.6986944345953,248.883493050375,24.4764888669701)) ;
#111672=CARTESIAN_POINT('Ctrl Pts',(58.6921642461824,249.004867232207,24.3943669735868)) ;
#111673=CARTESIAN_POINT('Ctrl Pts',(58.6908294958231,249.028845313321,24.3772050602596)) ;
#111674=CARTESIAN_POINT('Ctrl Pts',(58.6885817424774,249.067746451667,24.3477815857167)) ;
#111675=CARTESIAN_POINT('Ctrl Pts',(58.687682575334,249.082932548257,24.3358780299583)) ;
#111676=CARTESIAN_POINT('Ctrl Pts',(58.6858736959232,249.112717399393,24.3116904520405)) ;
#111677=CARTESIAN_POINT('Ctrl Pts',(58.6849643536074,249.127318621607,24.299414063143)) ;
#111678=CARTESIAN_POINT('Ctrl Pts',(58.6826817887202,249.163037362025,24.268327615606)) ;
#111679=CARTESIAN_POINT('Ctrl Pts',(58.681296740239,249.183894114938,24.249228013608)) ;
#111680=CARTESIAN_POINT('Ctrl Pts',(58.674558673086,249.281479774344,24.155220042489)) ;
#111681=CARTESIAN_POINT('Ctrl Pts',(58.6689178165271,249.351383794338,24.0736059583046)) ;
#111682=CARTESIAN_POINT('Ctrl Pts',(58.6582977029097,249.466061233093,23.9104003964724)) ;
#111683=CARTESIAN_POINT('Ctrl Pts',(58.6533605397259,249.512791377416,23.8306571743344)) ;
#111684=CARTESIAN_POINT('Ctrl Pts',(58.6477053890401,249.561305607179,23.7296094913164)) ;
#111685=CARTESIAN_POINT('Ctrl Pts',(58.6467194803946,249.569565230345,23.7115948643374)) ;
#111686=CARTESIAN_POINT('Ctrl Pts',(58.6451937806029,249.582071479195,23.6829910801999)) ;
#111687=CARTESIAN_POINT('Ctrl Pts',(58.6446423824,249.586532403169,23.6724981345098)) ;
#111688=CARTESIAN_POINT('Ctrl Pts',(58.6435725463192,249.595080412569,23.6518083168824)) ;
#111689=CARTESIAN_POINT('Ctrl Pts',(58.6430537413628,249.599174943509,23.6416153111299)) ;
#111690=CARTESIAN_POINT('Ctrl Pts',(58.6417098750084,249.609632840876,23.6148234755993)) ;
#111691=CARTESIAN_POINT('Ctrl Pts',(58.6408938454047,249.615833190677,23.5981620107676)) ;
#111692=CARTESIAN_POINT('Ctrl Pts',(58.6361593568661,249.65077928568,23.499485173232)) ;
#111693=CARTESIAN_POINT('Ctrl Pts',(58.6325187981103,249.673384600467,23.4154279840847)) ;
#111694=CARTESIAN_POINT('Ctrl Pts',(58.624176308611,249.710180687893,23.2188409489268)) ;
#111695=CARTESIAN_POINT('Ctrl Pts',(58.6194905188775,249.719694018365,23.1058737582084)) ;
#111696=CARTESIAN_POINT('Ctrl Pts',(58.613126656964,249.717265645328,22.9629602650058)) ;
#111697=CARTESIAN_POINT('Ctrl Pts',(58.6117757601395,249.715961390043,22.9331242656587)) ;
#111698=CARTESIAN_POINT('Ctrl Pts',(58.6095084885204,249.712500076772,22.8840242382705)) ;
#111699=CARTESIAN_POINT('Ctrl Pts',(58.6086064872593,249.710804158887,22.864734093427)) ;
#111700=CARTESIAN_POINT('Ctrl Pts',(58.6067978621239,249.706781787383,22.8265671273519)) ;
#111701=CARTESIAN_POINT('Ctrl Pts',(58.6058917460839,249.704467476912,22.807691935192)) ;
#111702=CARTESIAN_POINT('Ctrl Pts',(58.6036291117501,249.697961078725,22.7611857229054)) ;
#111703=CARTESIAN_POINT('Ctrl Pts',(58.6022612126478,249.693398594909,22.7336130070024)) ;
#111704=CARTESIAN_POINT('Ctrl Pts',(58.5955505633836,249.668030433951,22.6009666465405)) ;
#111705=CARTESIAN_POINT('Ctrl Pts',(58.5899194324147,249.637885583593,22.4979458718017)) ;
#111706=CARTESIAN_POINT('Ctrl Pts',(58.5792439998436,249.563448488295,22.3117512918139)) ;
#111707=CARTESIAN_POINT('Ctrl Pts',(58.5742415628301,249.521573424786,22.2280339232889)) ;
#111708=CARTESIAN_POINT('Ctrl Pts',(58.568539314449,249.462729399463,22.1314744743989)) ;
#111709=CARTESIAN_POINT('Ctrl Pts',(58.5675631160725,249.452221275872,22.1148931975161)) ;
#111710=CARTESIAN_POINT('Ctrl Pts',(58.5660488664004,249.435174366666,22.0890101317272)) ;
#111711=CARTESIAN_POINT('Ctrl Pts',(58.565499476295,249.42882812751,22.0795842206011)) ;
#111712=CARTESIAN_POINT('Ctrl Pts',(58.5644302806529,249.416142369524,22.0611494494127)) ;
#111713=CARTESIAN_POINT('Ctrl Pts',(58.5639101741161,249.409808993762,22.0521372149261)) ;
#111714=CARTESIAN_POINT('Ctrl Pts',(58.5625581970151,249.392935666634,22.0286226032031)) ;
#111715=CARTESIAN_POINT('Ctrl Pts',(58.561735565789,249.382250961371,22.0142252846363)) ;
#111716=CARTESIAN_POINT('Ctrl Pts',(58.5571890944492,249.321027141696,21.9344330456867)) ;
#111717=CARTESIAN_POINT('Ctrl Pts',(58.5537145890524,249.26593654388,21.8726658335845)) ;
#111718=CARTESIAN_POINT('Ctrl Pts',(58.5453362716452,249.121656529711,21.7331545956064)) ;
#111719=CARTESIAN_POINT('Ctrl Pts',(58.540460143388,249.028378067632,21.6602878179039)) ;
#111720=CARTESIAN_POINT('Ctrl Pts',(58.5338897740087,248.903303594657,21.582267572326)) ;
#111721=CARTESIAN_POINT('Ctrl Pts',(58.5325593846841,248.877971752257,21.5673754449325)) ;
#111722=CARTESIAN_POINT('Ctrl Pts',(58.5303168920002,248.835394780419,21.5438273895886)) ;
#111723=CARTESIAN_POINT('Ctrl Pts',(58.5294184804517,248.818367709945,21.5347898429423)) ;
#111724=CARTESIAN_POINT('Ctrl Pts',(58.5276094787576,248.784173224159,21.5173887300536)) ;
#111725=CARTESIAN_POINT('Ctrl Pts',(58.5266992206044,248.767011231781,21.5090208962999)) ;
#111726=CARTESIAN_POINT('Ctrl Pts',(58.524411039067,248.724000826396,21.4889511171973)) ;
#111727=CARTESIAN_POINT('Ctrl Pts',(58.5230211639088,248.697991953697,21.4776088243472)) ;
#111728=CARTESIAN_POINT('Ctrl Pts',(58.5167073842392,248.580383650691,21.4298324576466)) ;
#111729=CARTESIAN_POINT('Ctrl Pts',(58.5115460560139,248.485976780048,21.4008578236516)) ;
#111730=CARTESIAN_POINT('Ctrl Pts',(58.5008720152831,248.289637497897,21.359062711305)) ;
#111731=CARTESIAN_POINT('Ctrl Pts',(58.4953776921804,248.187952045253,21.3469615037871)) ;
#111732=CARTESIAN_POINT('Ctrl Pts',(58.4892756047735,248.066795757564,21.3436724668466)) ;
#111733=CARTESIAN_POINT('Ctrl Pts',(58.4883316948739,248.047789072863,21.3434795530609)) ;
#111734=CARTESIAN_POINT('Ctrl Pts',(58.4868555039266,248.017547584194,21.343686531784)) ;
#111735=CARTESIAN_POINT('Ctrl Pts',(58.4863127629332,248.006313406644,21.343876279719)) ;
#111736=CARTESIAN_POINT('Ctrl Pts',(58.4852451213693,247.983957828478,21.3444785552276)) ;
#111737=CARTESIAN_POINT('Ctrl Pts',(58.4847201473515,247.972836973909,21.3448889103273)) ;
#111738=CARTESIAN_POINT('Ctrl Pts',(58.4833383540921,247.943259950205,21.3462750865881)) ;
#111739=CARTESIAN_POINT('Ctrl Pts',(58.482491545943,247.924814012191,21.3474452866173)) ;
#111740=CARTESIAN_POINT('Ctrl Pts',(58.4783241605687,247.832757650797,21.3548143390947)) ;
#111741=CARTESIAN_POINT('Ctrl Pts',(58.4751973989511,247.759588383597,21.3655655741958)) ;
#111742=CARTESIAN_POINT('Ctrl Pts',(58.4667268005291,247.561682982708,21.408146299191)) ;
#111743=CARTESIAN_POINT('Ctrl Pts',(58.4614501685449,247.439537945236,21.4495389279885)) ;
#111744=CARTESIAN_POINT('Ctrl Pts',(58.4544488059768,247.297959053896,21.5164570714694)) ;
#111745=CARTESIAN_POINT('Ctrl Pts',(58.4531755358376,247.272906528287,21.5290762441629)) ;
#111746=CARTESIAN_POINT('Ctrl Pts',(58.4510894463472,247.233076424013,21.5504073115548)) ;
#111747=CARTESIAN_POINT('Ctrl Pts',(58.4502903316322,247.218095189481,21.5587283571787)) ;
#111748=CARTESIAN_POINT('Ctrl Pts',(58.4485889186806,247.186797123065,21.5767451072029)) ;
#111749=CARTESIAN_POINT('Ctrl Pts',(58.447684884219,247.170512153954,21.5864910932166)) ;
#111750=CARTESIAN_POINT('Ctrl Pts',(58.4454358629747,247.130860041733,21.6111446128651)) ;
#111751=CARTESIAN_POINT('Ctrl Pts',(58.4440798047152,247.107690837377,21.626358593766)) ;
#111752=CARTESIAN_POINT('Ctrl Pts',(58.437197109501,246.99376686969,21.7052734168937)) ;
#111753=CARTESIAN_POINT('Ctrl Pts',(58.4313577839772,246.909117391874,21.7772796676543)) ;
#111754=CARTESIAN_POINT('Ctrl Pts',(58.4206935283578,246.770156731069,21.9214734008873)) ;
#111755=CARTESIAN_POINT('Ctrl Pts',(58.4159159000148,246.71335763094,21.9907104003349)) ;
#111756=CARTESIAN_POINT('Ctrl Pts',(58.4103889491236,246.650897267652,22.0806266151527)) ;
#111757=CARTESIAN_POINT('Ctrl Pts',(58.4093900699783,246.639745807282,22.0973109073648)) ;
#111758=CARTESIAN_POINT('Ctrl Pts',(58.4078491050382,246.622703866114,22.1238258622081)) ;
#111759=CARTESIAN_POINT('Ctrl Pts',(58.4072950496932,246.616610453297,22.1335232629072)) ;
#111760=CARTESIAN_POINT('Ctrl Pts',(58.4062244929914,246.604890547417,22.1526059781332)) ;
#111761=CARTESIAN_POINT('Ctrl Pts',(58.4057075349024,246.599255729897,22.1619852778634)) ;
#111762=CARTESIAN_POINT('Ctrl Pts',(58.404374683682,246.584811067766,22.1865704374236)) ;
#111763=CARTESIAN_POINT('Ctrl Pts',(58.403567550519,246.576147427895,22.201861174364)) ;
#111764=CARTESIAN_POINT('Ctrl Pts',(58.4017846317166,246.557267414991,22.2364387520759)) ;
#111765=CARTESIAN_POINT('Ctrl Pts',(58.4008154108517,246.547183818055,22.2557946456414)) ;
#111766=CARTESIAN_POINT('Ctrl Pts',(58.397703865375,246.51558548612,22.3194499960749)) ;
#111767=CARTESIAN_POINT('Ctrl Pts',(58.3956187279498,246.495642111868,22.3645021501016)) ;
#111768=CARTESIAN_POINT('Ctrl Pts',(58.3878816574461,246.428423412721,22.5364189890206)) ;
#111769=CARTESIAN_POINT('Ctrl Pts',(58.3823497885551,246.394574102488,22.6679607977833)) ;
#111770=CARTESIAN_POINT('Ctrl Pts',(58.3750713163291,246.373355750385,22.8289883848575)) ;
#111771=CARTESIAN_POINT('Ctrl Pts',(58.3738396310956,246.370468698972,22.8559170571086)) ;
#111772=CARTESIAN_POINT('Ctrl Pts',(58.3717243950754,246.366694048073,22.9015134445233)) ;
#111773=CARTESIAN_POINT('Ctrl Pts',(58.370851616067,246.365464260998,22.9201478419344)) ;
#111774=CARTESIAN_POINT('Ctrl Pts',(58.3690466900847,246.363585878384,22.9582909590887)) ;
#111775=CARTESIAN_POINT('Ctrl Pts',(58.3681137805869,246.362966170763,22.977798187214)) ;
#111776=CARTESIAN_POINT('Ctrl Pts',(58.3656858914236,246.36224753231,23.0280114505093)) ;
#111777=CARTESIAN_POINT('Ctrl Pts',(58.3641756709277,246.362650989571,23.0587165050758)) ;
#111778=CARTESIAN_POINT('Ctrl Pts',(58.3607717902728,246.365413982445,23.1267593839296)) ;
#111779=CARTESIAN_POINT('Ctrl Pts',(58.3588671967442,246.368180251952,23.1640637223062)) ;
#111780=CARTESIAN_POINT('Ctrl Pts',(58.3522136656842,246.381983242826,23.292032202533)) ;
#111781=CARTESIAN_POINT('Ctrl Pts',(58.3473243659794,246.399171449346,23.3818663382931)) ;
#111782=CARTESIAN_POINT('Ctrl Pts',(58.3386915740641,246.442600760751,23.5384037208412)) ;
#111783=CARTESIAN_POINT('Ctrl Pts',(58.3349455946988,246.465963221582,23.6056846059942)) ;
#111784=CARTESIAN_POINT('Ctrl Pts',(58.3305352836636,246.50009545241,23.6869101854176)) ;
#111785=CARTESIAN_POINT('Ctrl Pts',(58.3296976069603,246.5068990544,23.7024378013214)) ;
#111786=CARTESIAN_POINT('Ctrl Pts',(58.3283984476285,246.517987934605,23.7267368703102)) ;
#111787=CARTESIAN_POINT('Ctrl Pts',(58.3279282180068,246.522116296513,23.7355783262644)) ;
#111788=CARTESIAN_POINT('Ctrl Pts',(58.3269255457853,246.531176009976,23.7545474762277)) ;
#111789=CARTESIAN_POINT('Ctrl Pts',(58.3263946983799,246.536132699469,23.7646625557054)) ;
#111790=CARTESIAN_POINT('Ctrl Pts',(58.3249775885554,246.549783758182,23.7918244381563)) ;
#111791=CARTESIAN_POINT('Ctrl Pts',(58.3241022699391,246.558668692689,23.8087740431688)) ;
#111792=CARTESIAN_POINT('Ctrl Pts',(58.3221384058258,246.579572301457,23.8470445146311)) ;
#111793=CARTESIAN_POINT('Ctrl Pts',(58.3210586706229,246.591771508122,23.8682620509178)) ;
#111794=CARTESIAN_POINT('Ctrl Pts',(58.3173760155993,246.635589618798,23.9407549596521)) ;
#111795=CARTESIAN_POINT('Ctrl Pts',(58.3148545498496,246.669503147108,23.9905909396671)) ;
#111796=CARTESIAN_POINT('Ctrl Pts',(58.3076432850708,246.7743178802,24.1280774838715)) ;
#111797=CARTESIAN_POINT('Ctrl Pts',(58.3029740208238,246.85145768565,24.2105507553264)) ;
#111798=CARTESIAN_POINT('Ctrl Pts',(58.2966279008363,246.958792838534,24.3043469209137)) ;
#111799=CARTESIAN_POINT('Ctrl Pts',(58.2952749658863,246.981833823012,24.3234196328338)) ;
#111800=CARTESIAN_POINT('Ctrl Pts',(58.2930048943598,247.020624717965,24.353819533697)) ;
#111801=CARTESIAN_POINT('Ctrl Pts',(58.2921021837853,247.036083521804,24.3655078012965)) ;
#111802=CARTESIAN_POINT('Ctrl Pts',(58.2902925822343,247.067110057282,24.3881327388936)) ;
#111803=CARTESIAN_POINT('Ctrl Pts',(58.289386209874,247.082668229832,24.3990776006084)) ;
#111804=CARTESIAN_POINT('Ctrl Pts',(58.2871237393485,247.121527625192,24.4254381932065)) ;
#111805=CARTESIAN_POINT('Ctrl Pts',(58.2857562855252,247.145033661721,24.440540566286)) ;
#111806=CARTESIAN_POINT('Ctrl Pts',(58.2824087606323,247.20260611765,24.4755307017307)) ;
#111807=CARTESIAN_POINT('Ctrl Pts',(58.2804101508806,247.236999629262,24.4948064669926)) ;
#111808=CARTESIAN_POINT('Ctrl Pts',(58.2783798877068,247.272019130299,24.5128441216388)) ;
#111809=CARTESIAN_POINT('Origin',(59.9402651077866,248.040265107786,23.0213203435596)) ;
#111810=CARTESIAN_POINT('',(67.9402651077866,250.003765107786,23.0213203435596)) ;
#111811=CARTESIAN_POINT('Origin',(67.9402651077866,248.040265107786,23.0213203435596)) ;
#111812=CARTESIAN_POINT('',(64.9402651077866,248.926035539849,24.773673901402)) ;
#111813=CARTESIAN_POINT('',(64.9402651077866,247.188367839728,24.7903888257486)) ;
#111814=CARTESIAN_POINT('Origin',(64.9402651077866,248.040265107786,23.0213203435596)) ;
#111815=CARTESIAN_POINT('',(65.2795522049911,250.003149224854,23.0202913881658)) ;
#111816=CARTESIAN_POINT('Ctrl Pts',(64.9402651077866,247.188367839728,24.7903888257487)) ;
#111817=CARTESIAN_POINT('Ctrl Pts',(64.966038653494,246.615402068142,24.5144764004132)) ;
#111818=CARTESIAN_POINT('Ctrl Pts',(65.0175857449088,245.767082084754,23.3666879407905)) ;
#111819=CARTESIAN_POINT('Ctrl Pts',(65.094906382031,246.471954521124,21.3360833564102)) ;
#111820=CARTESIAN_POINT('Ctrl Pts',(65.1722270191531,248.547505040093,20.777031256302)) ;
#111821=CARTESIAN_POINT('Ctrl Pts',(65.2337755287617,249.846624333595,21.8890188139763)) ;
#111822=CARTESIAN_POINT('Ctrl Pts',(65.2695504926629,250.002831124184,22.772803931472)) ;
#111823=CARTESIAN_POINT('Ctrl Pts',(65.2795519108567,250.001664111351,23.0202848861717)) ;
#111824=CARTESIAN_POINT('',(65.7795523268879,250.003764688188,23.0226039947667)) ;
#111825=CARTESIAN_POINT('Ctrl Pts',(65.2795523269168,250.003764839589,23.0202940833964)) ;
#111826=CARTESIAN_POINT('Ctrl Pts',(65.2823744169042,250.003801377307,23.0902001376797)) ;
#111827=CARTESIAN_POINT('Ctrl Pts',(65.2851965068916,250.00010029984,23.1601117387701)) ;
#111828=CARTESIAN_POINT('Ctrl Pts',(65.288018596879,249.992686234058,23.2296085949989)) ;
#111829=CARTESIAN_POINT('Ctrl Pts',(65.2908413713362,249.985270370068,23.2991223069976)) ;
#111830=CARTESIAN_POINT('Ctrl Pts',(65.2936641457934,249.974139780495,23.3682206035034)) ;
#111831=CARTESIAN_POINT('Ctrl Pts',(65.2964869202507,249.959370802772,23.4364896842759)) ;
#111832=CARTESIAN_POINT('Ctrl Pts',(65.2993133109198,249.944582904746,23.5048462234925)) ;
#111833=CARTESIAN_POINT('Ctrl Pts',(65.3021397015889,249.926147414425,23.5723709624915)) ;
#111834=CARTESIAN_POINT('Ctrl Pts',(65.304966092258,249.90419138201,23.6386623024912)) ;
#111835=CARTESIAN_POINT('Ctrl Pts',(65.3077944426461,249.882220126061,23.7049996065549)) ;
#111836=CARTESIAN_POINT('Ctrl Pts',(65.3106227930343,249.856723639135,23.7701013671339)) ;
#111837=CARTESIAN_POINT('Ctrl Pts',(65.3134511434225,249.827877287848,23.8335856596324)) ;
#111838=CARTESIAN_POINT('Ctrl Pts',(65.3162847933004,249.798976887053,23.8971889028677)) ;
#111839=CARTESIAN_POINT('Ctrl Pts',(65.3191184431784,249.766714305099,23.9591682047407)) ;
#111840=CARTESIAN_POINT('Ctrl Pts',(65.3219520930564,249.731310792157,24.0191663954992)) ;
#111841=CARTESIAN_POINT('Ctrl Pts',(65.3235908265034,249.710836519294,24.0538640632389)) ;
#111842=CARTESIAN_POINT('Ctrl Pts',(65.3252295599505,249.689312593963,24.0878996918042)) ;
#111843=CARTESIAN_POINT('Ctrl Pts',(65.3268682933975,249.666788097151,24.1212090720539)) ;
#111844=CARTESIAN_POINT('Ctrl Pts',(65.3296726910431,249.628241470824,24.17821208723)) ;
#111845=CARTESIAN_POINT('Ctrl Pts',(65.3324770886888,249.586624367975,24.2332903131143)) ;
#111846=CARTESIAN_POINT('Ctrl Pts',(65.3352814863345,249.542155517383,24.2860959946378)) ;
#111847=CARTESIAN_POINT('Ctrl Pts',(65.3381526298422,249.496628289149,24.3401584739413)) ;
#111848=CARTESIAN_POINT('Ctrl Pts',(65.3410237733499,249.448112038248,24.3918383687241)) ;
#111849=CARTESIAN_POINT('Ctrl Pts',(65.3438949168576,249.396889058754,24.4407933815775)) ;
#111850=CARTESIAN_POINT('Ctrl Pts',(65.346692200189,249.346983790579,24.4884890265612)) ;
#111851=CARTESIAN_POINT('Ctrl Pts',(65.3494894835203,249.294509759058,24.5335979427487)) ;
#111852=CARTESIAN_POINT('Ctrl Pts',(65.3522867668517,249.239767702999,24.5758382026002)) ;
#111853=CARTESIAN_POINT('Ctrl Pts',(65.3550824698301,249.185056574007,24.6180545983987)) ;
#111854=CARTESIAN_POINT('Ctrl Pts',(65.3578781728086,249.128080348433,24.6574052568979)) ;
#111855=CARTESIAN_POINT('Ctrl Pts',(65.360673875787,249.069173262012,24.6936481404244)) ;
#111856=CARTESIAN_POINT('Ctrl Pts',(65.3634689366283,249.010279705794,24.729882699425)) ;
#111857=CARTESIAN_POINT('Ctrl Pts',(65.3662639974696,248.949456584652,24.7630106461511)) ;
#111858=CARTESIAN_POINT('Ctrl Pts',(65.3690590583109,248.887066087755,24.7928339196646)) ;
#111859=CARTESIAN_POINT('Ctrl Pts',(65.3719865476616,248.821719562,24.8240702041577)) ;
#111860=CARTESIAN_POINT('Ctrl Pts',(65.3749140370124,248.754653949304,24.8516805938501)) ;
#111861=CARTESIAN_POINT('Ctrl Pts',(65.3778415263631,248.686310907772,24.8754932250139)) ;
#111862=CARTESIAN_POINT('Ctrl Pts',(65.3806398236742,248.620983889827,24.898254989028)) ;
#111863=CARTESIAN_POINT('Ctrl Pts',(65.3834381209853,248.554490323935,24.9175470485588)) ;
#111864=CARTESIAN_POINT('Ctrl Pts',(65.3862364182963,248.487231047264,24.933270577992)) ;
#111865=CARTESIAN_POINT('Ctrl Pts',(65.3890365162122,248.419928491641,24.9490042249572)) ;
#111866=CARTESIAN_POINT('Ctrl Pts',(65.3918366141281,248.351859724051,24.9611646863053)) ;
#111867=CARTESIAN_POINT('Ctrl Pts',(65.3946367120439,248.283433860123,24.9697045992665)) ;
#111868=CARTESIAN_POINT('Ctrl Pts',(65.3974411055399,248.214903025304,24.9782576131553)) ;
#111869=CARTESIAN_POINT('Ctrl Pts',(65.4002454990358,248.146014486428,24.9831789665619)) ;
#111870=CARTESIAN_POINT('Ctrl Pts',(65.4030498925317,248.077179448845,24.9844733130004)) ;
#111871=CARTESIAN_POINT('Ctrl Pts',(65.403429571861,248.067860057347,24.9846485511003)) ;
#111872=CARTESIAN_POINT('Ctrl Pts',(65.4038092511904,248.058541640326,24.9847573850822)) ;
#111873=CARTESIAN_POINT('Ctrl Pts',(65.4041889305197,248.049225210902,24.9847998994889)) ;
#111874=CARTESIAN_POINT('Ctrl Pts',(65.4069935126991,247.980407421991,24.9851139412027)) ;
#111875=CARTESIAN_POINT('Ctrl Pts',(65.4097980948786,247.911447888344,24.9818062564764)) ;
#111876=CARTESIAN_POINT('Ctrl Pts',(65.412602677058,247.842757201115,24.9748614556948)) ;
#111877=CARTESIAN_POINT('Ctrl Pts',(65.415473797499,247.772436838369,24.9677518906306)) ;
#111878=CARTESIAN_POINT('Ctrl Pts',(65.41834491794,247.702398755633,24.9568303285523)) ;
#111879=CARTESIAN_POINT('Ctrl Pts',(65.421216038381,247.63308477106,24.942136946826)) ;
#111880=CARTESIAN_POINT('Ctrl Pts',(65.4240135270963,247.565548388091,24.9278203863007)) ;
#111881=CARTESIAN_POINT('Ctrl Pts',(65.4268110158116,247.498699915975,24.9099232606698)) ;
#111882=CARTESIAN_POINT('Ctrl Pts',(65.4296085045269,247.432941807806,24.8885350230492)) ;
#111883=CARTESIAN_POINT('Ctrl Pts',(65.4324044200699,247.367220678815,24.8671588131385)) ;
#111884=CARTESIAN_POINT('Ctrl Pts',(65.4352003356129,247.302589159481,24.8422955377268)) ;
#111885=CARTESIAN_POINT('Ctrl Pts',(65.437996251156,247.239435639966,24.8140848047957)) ;
#111886=CARTESIAN_POINT('Ctrl Pts',(65.4407915314058,247.176296470313,24.7858804819607)) ;
#111887=CARTESIAN_POINT('Ctrl Pts',(65.4435868116556,247.114635078082,24.7543304112435)) ;
#111888=CARTESIAN_POINT('Ctrl Pts',(65.4463820919054,247.054819290828,24.7196220811314)) ;
#111889=CARTESIAN_POINT('Ctrl Pts',(65.4493093815501,246.992178654122,24.6832746217562)) ;
#111890=CARTESIAN_POINT('Ctrl Pts',(65.4522366711948,246.931562785623,24.6434634606412)) ;
#111891=CARTESIAN_POINT('Ctrl Pts',(65.4551639608395,246.873362514501,24.6004563692978)) ;
#111892=CARTESIAN_POINT('Ctrl Pts',(65.4579624923183,246.817722208763,24.559340964419)) ;
#111893=CARTESIAN_POINT('Ctrl Pts',(65.4607610237972,246.764289811874,24.5153052505619)) ;
#111894=CARTESIAN_POINT('Ctrl Pts',(65.4635595552761,246.71337298715,24.4686245790936)) ;
#111895=CARTESIAN_POINT('Ctrl Pts',(65.4663598922761,246.662423312553,24.4219137907796)) ;
#111896=CARTESIAN_POINT('Ctrl Pts',(65.4691602292762,246.613992781093,24.3725549962916)) ;
#111897=CARTESIAN_POINT('Ctrl Pts',(65.4719605662762,246.568351221111,24.3208594003846)) ;
#111898=CARTESIAN_POINT('Ctrl Pts',(65.4747652041905,246.522639562269,24.2690844074901)) ;
#111899=CARTESIAN_POINT('Ctrl Pts',(65.4775698421047,246.479725719894,24.2149658360299)) ;
#111900=CARTESIAN_POINT('Ctrl Pts',(65.480374480019,246.439837741792,24.1588459459873)) ;
#111901=CARTESIAN_POINT('Ctrl Pts',(65.4807528425599,246.434456613387,24.1512750349309)) ;
#111902=CARTESIAN_POINT('Ctrl Pts',(65.4811312051008,246.429130487227,24.1436677391668)) ;
#111903=CARTESIAN_POINT('Ctrl Pts',(65.4815095676418,246.423859859516,24.1360249337381)) ;
#111904=CARTESIAN_POINT('Ctrl Pts',(65.4843136713075,246.384798417421,24.0793829134542)) ;
#111905=CARTESIAN_POINT('Ctrl Pts',(65.4871177749731,246.34864643985,24.0205817797099)) ;
#111906=CARTESIAN_POINT('Ctrl Pts',(65.4899218786388,246.315648228617,23.959951724925)) ;
#111907=CARTESIAN_POINT('Ctrl Pts',(65.492793058894,246.281860671577,23.8978713466918)) ;
#111908=CARTESIAN_POINT('Ctrl Pts',(65.4956642391493,246.251380075197,23.8338737921426)) ;
#111909=CARTESIAN_POINT('Ctrl Pts',(65.4985354194045,246.22442260256,23.7683466123185)) ;
#111910=CARTESIAN_POINT('Ctrl Pts',(65.501332407077,246.198161723081,23.7045126841452)) ;
#111911=CARTESIAN_POINT('Ctrl Pts',(65.5041293947495,246.175244283028,23.6392277106462)) ;
#111912=CARTESIAN_POINT('Ctrl Pts',(65.5069263824221,246.155823425945,23.5728743279883)) ;
#111913=CARTESIAN_POINT('Ctrl Pts',(65.5097217900188,246.136413540102,23.5065584297199)) ;
#111914=CARTESIAN_POINT('Ctrl Pts',(65.5125171976155,246.120496453996,23.4391757870567)) ;
#111915=CARTESIAN_POINT('Ctrl Pts',(65.5153126052122,246.10817596721,23.3711257221154)) ;
#111916=CARTESIAN_POINT('Ctrl Pts',(65.5181073714904,246.095858306972,23.3030912691264)) ;
#111917=CARTESIAN_POINT('Ctrl Pts',(65.5209021377685,246.087135693778,23.2343901775297)) ;
#111918=CARTESIAN_POINT('Ctrl Pts',(65.5236969040467,246.082060793314,23.1654318031459)) ;
#111919=CARTESIAN_POINT('Ctrl Pts',(65.5266246791064,246.076744367707,23.0931915552718)) ;
#111920=CARTESIAN_POINT('Ctrl Pts',(65.5295524541662,246.075431614551,23.020669499252)) ;
#111921=CARTESIAN_POINT('Ctrl Pts',(65.532480229226,246.078121870574,22.9483397525469)) ;
#111922=CARTESIAN_POINT('Ctrl Pts',(65.5352782376675,246.080692887442,22.8792158486533)) ;
#111923=CARTESIAN_POINT('Ctrl Pts',(65.538076246109,246.086919464182,22.8102680703954)) ;
#111924=CARTESIAN_POINT('Ctrl Pts',(65.5408742545506,246.096747759992,22.74190565385)) ;
#111925=CARTESIAN_POINT('Ctrl Pts',(65.5436740658715,246.106582388604,22.6734991884048)) ;
#111926=CARTESIAN_POINT('Ctrl Pts',(65.5464738771925,246.120023260211,22.6056793131083)) ;
#111927=CARTESIAN_POINT('Ctrl Pts',(65.5492736885134,246.136965588452,22.5388442408341)) ;
#111928=CARTESIAN_POINT('Ctrl Pts',(65.5520778006902,246.1539339422,22.4719065016373)) ;
#111929=CARTESIAN_POINT('Ctrl Pts',(65.554881912867,246.174414335663,22.4059570469023)) ;
#111930=CARTESIAN_POINT('Ctrl Pts',(65.5576860250438,246.198252774597,22.3413771000614)) ;
#111931=CARTESIAN_POINT('Ctrl Pts',(65.5580674182839,246.201495091198,22.332593444624)) ;
#111932=CARTESIAN_POINT('Ctrl Pts',(65.5584488115239,246.20479945831,22.3238350896746)) ;
#111933=CARTESIAN_POINT('Ctrl Pts',(65.558830204764,246.208165422206,22.3151029605269)) ;
#111934=CARTESIAN_POINT('Ctrl Pts',(65.5616345176778,246.232914723003,22.2508972537607)) ;
#111935=CARTESIAN_POINT('Ctrl Pts',(65.5644388305917,246.261088319541,22.1878769827904)) ;
#111936=CARTESIAN_POINT('Ctrl Pts',(65.5672431435055,246.292551236391,22.126430141505)) ;
#111937=CARTESIAN_POINT('Ctrl Pts',(65.5701142976047,246.324764076207,22.0635187062759)) ;
#111938=CARTESIAN_POINT('Ctrl Pts',(65.5729854517039,246.36042495406,22.002257183029)) ;
#111939=CARTESIAN_POINT('Ctrl Pts',(65.5758566058031,246.39933570864,21.9430425699689)) ;
#111940=CARTESIAN_POINT('Ctrl Pts',(65.578653809421,246.437244263782,21.8853531098551)) ;
#111941=CARTESIAN_POINT('Ctrl Pts',(65.5814510130389,246.478237012326,21.8296068198098)) ;
#111942=CARTESIAN_POINT('Ctrl Pts',(65.5842482166568,246.522084271727,21.7761459786521)) ;
#111943=CARTESIAN_POINT('Ctrl Pts',(65.5870438420561,246.565906791934,21.7227153007958)) ;
#111944=CARTESIAN_POINT('Ctrl Pts',(65.5898394674554,246.612580318353,21.6715678890376)) ;
#111945=CARTESIAN_POINT('Ctrl Pts',(65.5926350928547,246.661833564721,21.6230146791631)) ;
#111946=CARTESIAN_POINT('Ctrl Pts',(65.595430078416,246.711075538442,21.5744725817173)) ;
#111947=CARTESIAN_POINT('Ctrl Pts',(65.5982250639774,246.762895712278,21.5285238487395)) ;
#111948=CARTESIAN_POINT('Ctrl Pts',(65.6010200495387,246.816985680048,21.4854428446451)) ;
#111949=CARTESIAN_POINT('Ctrl Pts',(65.6039476155676,246.873641411777,21.4403182880727)) ;
#111950=CARTESIAN_POINT('Ctrl Pts',(65.6068751815966,246.932787206431,21.3983406889682)) ;
#111951=CARTESIAN_POINT('Ctrl Pts',(65.6098027476256,246.994031275681,21.3597767785098)) ;
#111952=CARTESIAN_POINT('Ctrl Pts',(65.6126009764781,247.052569638242,21.3229165861707)) ;
#111953=CARTESIAN_POINT('Ctrl Pts',(65.6153992053307,247.113024308223,21.2891750086416)) ;
#111954=CARTESIAN_POINT('Ctrl Pts',(65.6181974341833,247.175026921842,21.2587383932423)) ;
#111955=CARTESIAN_POINT('Ctrl Pts',(65.620997466096,247.237069487318,21.2282821657777)) ;
#111956=CARTESIAN_POINT('Ctrl Pts',(65.6237974980087,247.300661533568,21.2011353298438)) ;
#111957=CARTESIAN_POINT('Ctrl Pts',(65.6265975299214,247.365415068727,21.1774359451272)) ;
#111958=CARTESIAN_POINT('Ctrl Pts',(65.6294018614015,247.430268035678,21.1537001690032)) ;
#111959=CARTESIAN_POINT('Ctrl Pts',(65.6322061928816,247.496285583913,21.1334225446893)) ;
#111960=CARTESIAN_POINT('Ctrl Pts',(65.6350105243617,247.563065999685,21.1166909147133)) ;
#111961=CARTESIAN_POINT('Ctrl Pts',(65.6353906302032,247.572117578043,21.1144230692974)) ;
#111962=CARTESIAN_POINT('Ctrl Pts',(65.6357707360447,247.581183160105,21.11222029248)) ;
#111963=CARTESIAN_POINT('Ctrl Pts',(65.6361508418862,247.590261736264,21.1100827299649)) ;
#111964=CARTESIAN_POINT('Ctrl Pts',(65.6389551462454,247.657240687697,21.0943124491003)) ;
#111965=CARTESIAN_POINT('Ctrl Pts',(65.6417594506045,247.725171800938,21.0820385006581)) ;
#111966=CARTESIAN_POINT('Ctrl Pts',(65.6445637549637,247.793658548226,21.0733682253641)) ;
#111967=CARTESIAN_POINT('Ctrl Pts',(65.6474349101322,247.863777926606,21.0644912624762)) ;
#111968=CARTESIAN_POINT('Ctrl Pts',(65.6503060653008,247.934479290863,21.0593922007207)) ;
#111969=CARTESIAN_POINT('Ctrl Pts',(65.6531772204693,248.005323040076,21.0581312793317)) ;
#111970=CARTESIAN_POINT('Ctrl Pts',(65.6559744166489,248.074341902875,21.0569028384132)) ;
#111971=CARTESIAN_POINT('Ctrl Pts',(65.6587716128286,248.143495383548,21.0593171883109)) ;
#111972=CARTESIAN_POINT('Ctrl Pts',(65.6615688090083,248.212371297335,21.0653776783675)) ;
#111973=CARTESIAN_POINT('Ctrl Pts',(65.6643644274066,248.281208361103,21.0714347499553)) ;
#111974=CARTESIAN_POINT('Ctrl Pts',(65.667160045805,248.349767684046,21.0811338376912)) ;
#111975=CARTESIAN_POINT('Ctrl Pts',(65.6699556642034,248.417639503082,21.0944262583087)) ;
#111976=CARTESIAN_POINT('Ctrl Pts',(65.6727506432144,248.485495799118,21.1077156388094)) ;
#111977=CARTESIAN_POINT('Ctrl Pts',(65.6755456222253,248.552664425469,21.1245966259919)) ;
#111978=CARTESIAN_POINT('Ctrl Pts',(65.6783406012363,248.618744887007,21.1449692583328)) ;
#111979=CARTESIAN_POINT('Ctrl Pts',(65.681268174384,248.687960213501,21.166308370775)) ;
#111980=CARTESIAN_POINT('Ctrl Pts',(65.6841957475316,248.755980993142,21.1914785334642)) ;
#111981=CARTESIAN_POINT('Ctrl Pts',(65.6871233206793,248.822366006382,21.2203066194546)) ;
#111982=CARTESIAN_POINT('Ctrl Pts',(65.6899215441968,248.885817915484,21.2478609875651)) ;
#111983=CARTESIAN_POINT('Ctrl Pts',(65.6927197677142,248.947775128316,21.2787565729496)) ;
#111984=CARTESIAN_POINT('Ctrl Pts',(65.6955179912317,249.007876023601,21.3127942636895)) ;
#111985=CARTESIAN_POINT('Ctrl Pts',(65.6983180182362,249.0680156546,21.3468538921104)) ;
#111986=CARTESIAN_POINT('Ctrl Pts',(65.7011180452407,249.126296176496,21.3840593941392)) ;
#111987=CARTESIAN_POINT('Ctrl Pts',(65.7039180722452,249.182384775927,21.4241682175409)) ;
#111988=CARTESIAN_POINT('Ctrl Pts',(65.7067223994572,249.238559514747,21.4643386390141)) ;
#111989=CARTESIAN_POINT('Ctrl Pts',(65.7095267266692,249.292535237366,21.5074209713915)) ;
#111990=CARTESIAN_POINT('Ctrl Pts',(65.7123310538812,249.344012862449,21.5531330114348)) ;
#111991=CARTESIAN_POINT('Ctrl Pts',(65.7127111955903,249.35099093273,21.5593295255051)) ;
#111992=CARTESIAN_POINT('Ctrl Pts',(65.7130913372993,249.357923157329,21.5655743079424)) ;
#111993=CARTESIAN_POINT('Ctrl Pts',(65.7134714790084,249.364808846371,21.5718666069489)) ;
#111994=CARTESIAN_POINT('Ctrl Pts',(65.7162356678715,249.414877924591,21.61762086759)) ;
#111995=CARTESIAN_POINT('Ctrl Pts',(65.7189998567346,249.462677693738,21.6660680056072)) ;
#111996=CARTESIAN_POINT('Ctrl Pts',(65.7217640455977,249.50790051215,21.7169513122429)) ;
#111997=CARTESIAN_POINT('Ctrl Pts',(65.7245247450279,249.553066242569,21.7677703852476)) ;
#111998=CARTESIAN_POINT('Ctrl Pts',(65.727285444458,249.595661137275,21.8210191605267)) ;
#111999=CARTESIAN_POINT('Ctrl Pts',(65.7300461438882,249.635412551539,21.8764024938038)) ;
#112000=CARTESIAN_POINT('Ctrl Pts',(65.7328043528181,249.675128104997,21.9317358643068)) ;
#112001=CARTESIAN_POINT('Ctrl Pts',(65.7355625617481,249.7120049712,21.9891995688869)) ;
#112002=CARTESIAN_POINT('Ctrl Pts',(65.738320770678,249.745810455506,22.0484651041374)) ;
#112003=CARTESIAN_POINT('Ctrl Pts',(65.7410774846502,249.779597617135,22.1076985172849)) ;
#112004=CARTESIAN_POINT('Ctrl Pts',(65.7438341986225,249.81031645043,22.1687313877624)) ;
#112005=CARTESIAN_POINT('Ctrl Pts',(65.7465909125947,249.837778407826,22.2312075755451)) ;
#112006=CARTESIAN_POINT('Ctrl Pts',(65.749348553021,249.865249594414,22.2937047598186)) ;
#112007=CARTESIAN_POINT('Ctrl Pts',(65.7521061934473,249.889461502537,22.3576457753752)) ;
#112008=CARTESIAN_POINT('Ctrl Pts',(65.7548638338736,249.910272881316,22.4226525083319)) ;
#112009=CARTESIAN_POINT('Ctrl Pts',(65.7576217613921,249.931086426725,22.487666009006)) ;
#112010=CARTESIAN_POINT('Ctrl Pts',(65.7603796889107,249.948498597497,22.5537449641857)) ;
#112011=CARTESIAN_POINT('Ctrl Pts',(65.7631376164293,249.962418217271,22.6204965996326)) ;
#112012=CARTESIAN_POINT('Ctrl Pts',(65.765899358522,249.976357089699,22.6873405613132)) ;
#112013=CARTESIAN_POINT('Ctrl Pts',(65.7686611006147,249.986793672311,22.754858565243)) ;
#112014=CARTESIAN_POINT('Ctrl Pts',(65.7714228427074,249.993688246243,22.8226490267054)) ;
#112015=CARTESIAN_POINT('Ctrl Pts',(65.7741326707675,250.000453218959,22.8891651924147)) ;
#112016=CARTESIAN_POINT('Ctrl Pts',(65.7768424988277,250.003808268137,22.9559431984112)) ;
#112017=CARTESIAN_POINT('Ctrl Pts',(65.7795523268879,250.003764688188,23.0226039947667)) ;
#112018=CARTESIAN_POINT('',(66.2795523268944,250.003764624032,23.019942046258)) ;
#112019=CARTESIAN_POINT('Ctrl Pts',(65.7795523269168,250.003764688188,23.0226039954774)) ;
#112020=CARTESIAN_POINT('Ctrl Pts',(65.7832989233214,250.003704434708,23.1147689204846)) ;
#112021=CARTESIAN_POINT('Ctrl Pts',(65.787045519726,249.997153658522,23.2067142655956)) ;
#112022=CARTESIAN_POINT('Ctrl Pts',(65.7907921161306,249.984212027855,23.2977305856885)) ;
#112023=CARTESIAN_POINT('Ctrl Pts',(65.7935964027768,249.974525358105,23.3658553110284)) ;
#112024=CARTESIAN_POINT('Ctrl Pts',(65.796400689423,249.961235643221,23.43359451641)) ;
#112025=CARTESIAN_POINT('Ctrl Pts',(65.7992049760692,249.94438720405,23.5005398053073)) ;
#112026=CARTESIAN_POINT('Ctrl Pts',(65.8020761334518,249.927136998699,23.5690814648099)) ;
#112027=CARTESIAN_POINT('Ctrl Pts',(65.8049472908345,249.906156147452,23.6367903357438)) ;
#112028=CARTESIAN_POINT('Ctrl Pts',(65.8078184482171,249.881548520379,23.7032350336118)) ;
#112029=CARTESIAN_POINT('Ctrl Pts',(65.8106156254977,249.857574949375,23.7679676743284)) ;
#112030=CARTESIAN_POINT('Ctrl Pts',(65.8134128027783,249.830159435462,23.8315000181063)) ;
#112031=CARTESIAN_POINT('Ctrl Pts',(65.8162099800589,249.79944885858,23.8934469289492)) ;
#112032=CARTESIAN_POINT('Ctrl Pts',(65.8190055791721,249.768755608605,23.9553588893453)) ;
#112033=CARTESIAN_POINT('Ctrl Pts',(65.8218011782852,249.734771201065,24.0156867560399)) ;
#112034=CARTESIAN_POINT('Ctrl Pts',(65.8245967773984,249.697690099425,24.0740665841562)) ;
#112035=CARTESIAN_POINT('Ctrl Pts',(65.8273917367707,249.660617483372,24.1324330527153)) ;
#112036=CARTESIAN_POINT('Ctrl Pts',(65.8301866961429,249.620449842153,24.188851956971)) ;
#112037=CARTESIAN_POINT('Ctrl Pts',(65.8329816555152,249.577426028614,24.242986645575)) ;
#112038=CARTESIAN_POINT('Ctrl Pts',(65.8359092469933,249.532360561428,24.2996902437033)) ;
#112039=CARTESIAN_POINT('Ctrl Pts',(65.8388368384714,249.484161425465,24.353886957013)) ;
#112040=CARTESIAN_POINT('Ctrl Pts',(65.8417644299495,249.43315045536,24.4052288154293)) ;
#112041=CARTESIAN_POINT('Ctrl Pts',(65.8445626331684,249.384393973519,24.4543015615948)) ;
#112042=CARTESIAN_POINT('Ctrl Pts',(65.8473608363873,249.333069380292,24.5007661813769)) ;
#112043=CARTESIAN_POINT('Ctrl Pts',(65.8501590396061,249.279493733614,24.5443583151576)) ;
#112044=CARTESIAN_POINT('Ctrl Pts',(65.8529590461022,249.225883560586,24.5879785415018)) ;
#112045=CARTESIAN_POINT('Ctrl Pts',(65.8557590525983,249.170019840529,24.6287223107889)) ;
#112046=CARTESIAN_POINT('Ctrl Pts',(65.8585590590943,249.112249609004,24.666367904923)) ;
#112047=CARTESIAN_POINT('Ctrl Pts',(65.8613633656434,249.054390658023,24.7040713125116)) ;
#112048=CARTESIAN_POINT('Ctrl Pts',(65.8641676721924,248.994619776891,24.7386668120721)) ;
#112049=CARTESIAN_POINT('Ctrl Pts',(65.8669719787414,248.933308657236,24.7699785345121)) ;
#112050=CARTESIAN_POINT('Ctrl Pts',(65.8673522369118,248.924994996166,24.7742243393411)) ;
#112051=CARTESIAN_POINT('Ctrl Pts',(65.8677324950823,248.916653043686,24.7784098390137)) ;
#112052=CARTESIAN_POINT('Ctrl Pts',(65.8681127532527,248.908283751993,24.7825346642227)) ;
#112053=CARTESIAN_POINT('Ctrl Pts',(65.8709170369376,248.846562873984,24.8129539449544)) ;
#112054=CARTESIAN_POINT('Ctrl Pts',(65.8737213206225,248.783128441438,24.8401803846571)) ;
#112055=CARTESIAN_POINT('Ctrl Pts',(65.8765256043074,248.718342706596,24.8640202702952)) ;
#112056=CARTESIAN_POINT('Ctrl Pts',(65.8793967620602,248.652012019061,24.888428668363)) ;
#112057=CARTESIAN_POINT('Ctrl Pts',(65.882267919813,248.584265172412,24.9092866076984)) ;
#112058=CARTESIAN_POINT('Ctrl Pts',(65.8851390775658,248.515516986662,24.9264365871587)) ;
#112059=CARTESIAN_POINT('Ctrl Pts',(65.8879362518848,248.448540290772,24.9431446492884)) ;
#112060=CARTESIAN_POINT('Ctrl Pts',(65.8907334262039,248.380613744292,24.9563334198147)) ;
#112061=CARTESIAN_POINT('Ctrl Pts',(65.8935306005229,248.312138228577,24.9659069978878)) ;
#112062=CARTESIAN_POINT('Ctrl Pts',(65.8963261966832,248.243701346575,24.9754751745723)) ;
#112063=CARTESIAN_POINT('Ctrl Pts',(65.8991217928436,248.174716591821,24.9814321391608)) ;
#112064=CARTESIAN_POINT('Ctrl Pts',(65.9019173890039,248.105594180368,24.9837332364737)) ;
#112065=CARTESIAN_POINT('Ctrl Pts',(65.9047123454372,248.036487586461,24.9860338072178)) ;
#112066=CARTESIAN_POINT('Ctrl Pts',(65.9075073018706,247.967243885384,24.9846801563403)) ;
#112067=CARTESIAN_POINT('Ctrl Pts',(65.910302258304,247.898275787108,24.979679678006)) ;
#112068=CARTESIAN_POINT('Ctrl Pts',(65.9132298526432,247.826034727573,24.9744418961608)) ;
#112069=CARTESIAN_POINT('Ctrl Pts',(65.9161574469824,247.754096661642,24.9652025381079)) ;
#112070=CARTESIAN_POINT('Ctrl Pts',(65.9190850413217,247.682930446395,24.9520311426614)) ;
#112071=CARTESIAN_POINT('Ctrl Pts',(65.9218832416723,247.61490963976,24.9394418973338)) ;
#112072=CARTESIAN_POINT('Ctrl Pts',(65.9246814420229,247.547594376103,24.9232610403567)) ;
#112073=CARTESIAN_POINT('Ctrl Pts',(65.9274796423735,247.481381769452,24.9036013173074)) ;
#112074=CARTESIAN_POINT('Ctrl Pts',(65.9302796460286,247.415126491985,24.8839289245192)) ;
#112075=CARTESIAN_POINT('Ctrl Pts',(65.9330796496838,247.349975744644,24.8607733669104)) ;
#112076=CARTESIAN_POINT('Ctrl Pts',(65.9358796533389,247.286308333306,24.8342961934308)) ;
#112077=CARTESIAN_POINT('Ctrl Pts',(65.9386839571058,247.222543144603,24.8077783575741)) ;
#112078=CARTESIAN_POINT('Ctrl Pts',(65.9414882608727,247.160266273636,24.7779289420924)) ;
#112079=CARTESIAN_POINT('Ctrl Pts',(65.9442925646396,247.099832568283,24.7449557135392)) ;
#112080=CARTESIAN_POINT('Ctrl Pts',(65.9446728398847,247.091637506683,24.7404844067148)) ;
#112081=CARTESIAN_POINT('Ctrl Pts',(65.9450531151298,247.083476293981,24.7359557225224)) ;
#112082=CARTESIAN_POINT('Ctrl Pts',(65.9454333903749,247.075349772257,24.7313702391066)) ;
#112083=CARTESIAN_POINT('Ctrl Pts',(65.9482376714969,247.015421991652,24.6975552991565)) ;
#112084=CARTESIAN_POINT('Ctrl Pts',(65.951041952619,246.957164536995,24.6605247010187)) ;
#112085=CARTESIAN_POINT('Ctrl Pts',(65.953846233741,246.900941669287,24.6204683518713)) ;
#112086=CARTESIAN_POINT('Ctrl Pts',(65.9567173918141,246.843377989508,24.5794567324105)) ;
#112087=CARTESIAN_POINT('Ctrl Pts',(65.9595885498873,246.787947679348,24.5352733627102)) ;
#112088=CARTESIAN_POINT('Ctrl Pts',(65.9624597079605,246.73501474225,24.4881719833885)) ;
#112089=CARTESIAN_POINT('Ctrl Pts',(65.9652568795533,246.683445826781,24.4422843530792)) ;
#112090=CARTESIAN_POINT('Ctrl Pts',(65.9680540511461,246.634247511617,24.3936276378542)) ;
#112091=CARTESIAN_POINT('Ctrl Pts',(65.970851222739,246.587725068246,24.3424788062479)) ;
#112092=CARTESIAN_POINT('Ctrl Pts',(65.9736468161203,246.541228873624,24.2913588336764)) ;
#112093=CARTESIAN_POINT('Ctrl Pts',(65.9764424095017,246.497405882032,24.2377498950117)) ;
#112094=CARTESIAN_POINT('Ctrl Pts',(65.979238002883,246.456524310034,24.1819655673617)) ;
#112095=CARTESIAN_POINT('Ctrl Pts',(65.9820329564894,246.415652093834,24.1261940060242)) ;
#112096=CARTESIAN_POINT('Ctrl Pts',(65.9848279100957,246.377720248034,24.0682484376437)) ;
#112097=CARTESIAN_POINT('Ctrl Pts',(65.9876228637021,246.342955412737,24.0084738519319)) ;
#112098=CARTESIAN_POINT('Ctrl Pts',(65.990550460685,246.306540702061,23.9458624739157)) ;
#112099=CARTESIAN_POINT('Ctrl Pts',(65.9934780576679,246.2736014171,23.8812446314221)) ;
#112100=CARTESIAN_POINT('Ctrl Pts',(65.9964056546508,246.244344543332,23.8150467297727)) ;
#112101=CARTESIAN_POINT('Ctrl Pts',(65.9992038520868,246.21638082099,23.7517747699573)) ;
#112102=CARTESIAN_POINT('Ctrl Pts',(66.0020020495227,246.191780974643,23.6870599811615)) ;
#112103=CARTESIAN_POINT('Ctrl Pts',(66.0048002469586,246.170675848666,23.6212938864612)) ;
#112104=CARTESIAN_POINT('Ctrl Pts',(66.0076002476715,246.149557121651,23.5554854093052)) ;
#112105=CARTESIAN_POINT('Ctrl Pts',(66.0104002483843,246.131937721229,23.4886247488484)) ;
#112106=CARTESIAN_POINT('Ctrl Pts',(66.0132002490971,246.11789786458,23.4211158315903)) ;
#112107=CARTESIAN_POINT('Ctrl Pts',(66.016004549903,246.103836446261,23.3535032377054)) ;
#112108=CARTESIAN_POINT('Ctrl Pts',(66.0188088507089,246.093365609272,23.2852408819788)) ;
#112109=CARTESIAN_POINT('Ctrl Pts',(66.0216131515148,246.08651389274,23.2167389703751)) ;
#112110=CARTESIAN_POINT('Ctrl Pts',(66.0219934435089,246.0855847296,23.2074494075337)) ;
#112111=CARTESIAN_POINT('Ctrl Pts',(66.022373735503,246.084722044184,23.1981554393433)) ;
#112112=CARTESIAN_POINT('Ctrl Pts',(66.0227540274971,246.083925833939,23.1888580873805)) ;
#112113=CARTESIAN_POINT('Ctrl Pts',(66.0255583084631,246.078054563263,23.1202992232747)) ;
#112114=CARTESIAN_POINT('Ctrl Pts',(66.0283625894291,246.075780794755,23.0513062766017)) ;
#112115=CARTESIAN_POINT('Ctrl Pts',(66.0311668703951,246.077153124161,22.9822871557965)) ;
#112116=CARTESIAN_POINT('Ctrl Pts',(66.0340380284878,246.078558181188,22.9116220513894)) ;
#112117=CARTESIAN_POINT('Ctrl Pts',(66.0369091865804,246.083785612578,22.8409300130663)) ;
#112118=CARTESIAN_POINT('Ctrl Pts',(66.0397803446731,246.092831154402,22.7706547352107)) ;
#112119=CARTESIAN_POINT('Ctrl Pts',(66.042577516201,246.10164360263,22.7021903734493)) ;
#112120=CARTESIAN_POINT('Ctrl Pts',(66.0453746877289,246.114079684301,22.6341220671762)) ;
#112121=CARTESIAN_POINT('Ctrl Pts',(66.0481718592568,246.130082831969,22.566858108434)) ;
#112122=CARTESIAN_POINT('Ctrl Pts',(66.050967452607,246.146076950585,22.4996321003405)) ;
#112123=CARTESIAN_POINT('Ctrl Pts',(66.0537630459573,246.165634028701,22.4332100124937)) ;
#112124=CARTESIAN_POINT('Ctrl Pts',(66.0565586393075,246.188646370115,22.3679901817676)) ;
#112125=CARTESIAN_POINT('Ctrl Pts',(66.0593535929166,246.211653445405,22.302785275892)) ;
#112126=CARTESIAN_POINT('Ctrl Pts',(66.0621485465256,246.238114051163,22.2387825400709)) ;
#112127=CARTESIAN_POINT('Ctrl Pts',(66.0649435001347,246.267871103425,22.1763636918273)) ;
#112128=CARTESIAN_POINT('Ctrl Pts',(66.0678710971751,246.299040371442,22.1109825582049)) ;
#112129=CARTESIAN_POINT('Ctrl Pts',(66.0707986942155,246.33382655352,22.047339934533)) ;
#112130=CARTESIAN_POINT('Ctrl Pts',(66.0737262912559,246.371994247573,21.9858472212796)) ;
#112131=CARTESIAN_POINT('Ctrl Pts',(66.0765244887789,246.408474933093,21.9270724802423)) ;
#112132=CARTESIAN_POINT('Ctrl Pts',(66.0793226863019,246.448044167759,21.8702619899651)) ;
#112133=CARTESIAN_POINT('Ctrl Pts',(66.082120883825,246.490452416229,21.8157446009826)) ;
#112134=CARTESIAN_POINT('Ctrl Pts',(66.0849208846539,246.53288799481,21.7611920781217)) ;
#112135=CARTESIAN_POINT('Ctrl Pts',(66.0877208854829,246.578165909477,21.7089359656719)) ;
#112136=CARTESIAN_POINT('Ctrl Pts',(66.0905208863119,246.625997831022,21.6592703004726)) ;
#112137=CARTESIAN_POINT('Ctrl Pts',(66.0933251872741,246.673903210985,21.6095283606616)) ;
#112138=CARTESIAN_POINT('Ctrl Pts',(66.0961294882363,246.724370065361,21.5623851343566)) ;
#112139=CARTESIAN_POINT('Ctrl Pts',(66.0989337891985,246.777075735682,21.5180955233138)) ;
#112140=CARTESIAN_POINT('Ctrl Pts',(66.0993140810054,246.784223162036,21.5120894004193)) ;
#112141=CARTESIAN_POINT('Ctrl Pts',(66.0996943728124,246.791411716169,21.5061356911673)) ;
#112142=CARTESIAN_POINT('Ctrl Pts',(66.1000746646193,246.798640553014,21.500234969563)) ;
#112143=CARTESIAN_POINT('Ctrl Pts',(66.1028789485387,246.851946226575,21.4567228601616)) ;
#112144=CARTESIAN_POINT('Ctrl Pts',(66.1056832324581,246.907639171652,21.4159368162257)) ;
#112145=CARTESIAN_POINT('Ctrl Pts',(66.1084875163775,246.965409937471,21.3781470073448)) ;
#112146=CARTESIAN_POINT('Ctrl Pts',(66.111358674101,247.024558363679,21.3394560242788)) ;
#112147=CARTESIAN_POINT('Ctrl Pts',(66.1142298318245,247.085884643482,21.303906411777)) ;
#112148=CARTESIAN_POINT('Ctrl Pts',(66.117100989548,247.14901996494,21.2717448678076)) ;
#112149=CARTESIAN_POINT('Ctrl Pts',(66.1198981639646,247.210528430505,21.2404120548259)) ;
#112150=CARTESIAN_POINT('Ctrl Pts',(66.1226953383813,247.273753365653,21.212295040097)) ;
#112151=CARTESIAN_POINT('Ctrl Pts',(66.125492512798,247.338325696517,21.1875773645937)) ;
#112152=CARTESIAN_POINT('Ctrl Pts',(66.128288109005,247.40286159466,21.1628736351897)) ;
#112153=CARTESIAN_POINT('Ctrl Pts',(66.1310837052121,247.468742925502,21.1415656127726)) ;
#112154=CARTESIAN_POINT('Ctrl Pts',(66.1338793014192,247.535580002394,21.1237890014218)) ;
#112155=CARTESIAN_POINT('Ctrl Pts',(66.1366742578485,247.602401783486,21.1060164582841)) ;
#112156=CARTESIAN_POINT('Ctrl Pts',(66.1394692142778,247.670178405283,21.0917738460281)) ;
#112157=CARTESIAN_POINT('Ctrl Pts',(66.1422641707071,247.738506053524,21.0811467113372)) ;
#112158=CARTESIAN_POINT('Ctrl Pts',(66.1451917649599,247.810076267716,21.0700152539309)) ;
#112159=CARTESIAN_POINT('Ctrl Pts',(66.1481193592128,247.882250543566,21.0628511036595)) ;
#112160=CARTESIAN_POINT('Ctrl Pts',(66.1510469534657,247.954556389716,21.0596918706711)) ;
#112161=CARTESIAN_POINT('Ctrl Pts',(66.1538451536853,248.023666456584,21.0566722697024)) ;
#112162=CARTESIAN_POINT('Ctrl Pts',(66.156643353905,248.092896198804,21.0573109666162)) ;
#112163=CARTESIAN_POINT('Ctrl Pts',(66.1594415541247,248.161833322598,21.0615873466574)) ;
#112164=CARTESIAN_POINT('Ctrl Pts',(66.1622415576052,248.230814871954,21.0658664825516)) ;
#112165=CARTESIAN_POINT('Ctrl Pts',(66.1650415610857,248.299502943777,21.0737879112051)) ;
#112166=CARTESIAN_POINT('Ctrl Pts',(66.1678415645663,248.367492116105,21.0852793483772)) ;
#112167=CARTESIAN_POINT('Ctrl Pts',(66.1706458680983,248.435585701495,21.0967884333028)) ;
#112168=CARTESIAN_POINT('Ctrl Pts',(66.1734501716303,248.50297777235,21.1118783550531)) ;
#112169=CARTESIAN_POINT('Ctrl Pts',(66.1762544751623,248.569275864971,21.1304264097859)) ;
#112170=CARTESIAN_POINT('Ctrl Pts',(66.1766347506886,248.578266169259,21.1329416051619)) ;
#112171=CARTESIAN_POINT('Ctrl Pts',(66.177015026215,248.587236385339,21.1355203173889)) ;
#112172=CARTESIAN_POINT('Ctrl Pts',(66.1773953017414,248.596185562741,21.1381621723581)) ;
#112173=CARTESIAN_POINT('Ctrl Pts',(66.1801995884356,248.662179973029,21.1576441485155)) ;
#112174=CARTESIAN_POINT('Ctrl Pts',(66.1830038751297,248.727269454682,21.1806349226248)) ;
#112175=CARTESIAN_POINT('Ctrl Pts',(66.1858081618239,248.791056384375,21.2070313067749)) ;
#112176=CARTESIAN_POINT('Ctrl Pts',(66.1886793192006,248.856364369505,21.2340571359195)) ;
#112177=CARTESIAN_POINT('Ctrl Pts',(66.1915504765772,248.920306364013,21.2646530243737)) ;
#112178=CARTESIAN_POINT('Ctrl Pts',(66.1944216339539,248.982470652671,21.2986535269093)) ;
#112179=CARTESIAN_POINT('Ctrl Pts',(66.1972188112544,249.043033176535,21.3317779507649)) ;
#112180=CARTESIAN_POINT('Ctrl Pts',(66.200015988555,249.101908047876,21.3681333979902)) ;
#112181=CARTESIAN_POINT('Ctrl Pts',(66.2028131658556,249.158735558242,21.4075185894839)) ;
#112182=CARTESIAN_POINT('Ctrl Pts',(66.2056087649783,249.215531006315,21.4468815597063)) ;
#112183=CARTESIAN_POINT('Ctrl Pts',(66.2084043641011,249.270280985882,21.4892706047942)) ;
#112184=CARTESIAN_POINT('Ctrl Pts',(66.2111999632238,249.322653668317,21.534440445982)) ;
#112185=CARTESIAN_POINT('Ctrl Pts',(66.2139949225952,249.375014365666,21.5795999503994)) ;
#112186=CARTESIAN_POINT('Ctrl Pts',(66.2167898819666,249.42499847763,21.6275386685791)) ;
#112187=CARTESIAN_POINT('Ctrl Pts',(66.219584841338,249.472307628976,21.6779713689805)) ;
#112188=CARTESIAN_POINT('Ctrl Pts',(66.2225124327985,249.521861790264,21.7307973043174)) ;
#112189=CARTESIAN_POINT('Ctrl Pts',(66.225440024259,249.568480366161,21.786359421252)) ;
#112190=CARTESIAN_POINT('Ctrl Pts',(66.2283676157194,249.611865839533,21.8442887424657)) ;
#112191=CARTESIAN_POINT('Ctrl Pts',(66.2311658189115,249.653333842059,21.8996578107674)) ;
#112192=CARTESIAN_POINT('Ctrl Pts',(66.2339640221036,249.691848263824,21.9571887949095)) ;
#112193=CARTESIAN_POINT('Ctrl Pts',(66.2367622252956,249.727193616902,22.0165295916453)) ;
#112194=CARTESIAN_POINT('Ctrl Pts',(66.239562231756,249.762561747866,22.0759086298412)) ;
#112195=CARTESIAN_POINT('Ctrl Pts',(66.2423622382163,249.794756518943,22.1370993707667)) ;
#112196=CARTESIAN_POINT('Ctrl Pts',(66.2451622446767,249.823608986797,22.199726247187)) ;
#112197=CARTESIAN_POINT('Ctrl Pts',(66.2479665511776,249.852505764114,22.2624493012825)) ;
#112198=CARTESIAN_POINT('Ctrl Pts',(66.2507708576786,249.87804982134,22.3266124379175)) ;
#112199=CARTESIAN_POINT('Ctrl Pts',(66.2535751641795,249.900121159985,22.3918223569875)) ;
#112200=CARTESIAN_POINT('Ctrl Pts',(66.2539554224075,249.90311398838,22.4006646886898)) ;
#112201=CARTESIAN_POINT('Ctrl Pts',(66.2543356806356,249.906043040956,22.4095262496389)) ;
#112202=CARTESIAN_POINT('Ctrl Pts',(66.2547159388636,249.908908090672,22.4184060440853)) ;
#112203=CARTESIAN_POINT('Ctrl Pts',(66.2580138048557,249.933755810796,22.4954178480688)) ;
#112204=CARTESIAN_POINT('Ctrl Pts',(66.2613116708477,249.953858330787,22.5740280426585)) ;
#112205=CARTESIAN_POINT('Ctrl Pts',(66.2646095368398,249.969042667699,22.6536936655638)) ;
#112206=CARTESIAN_POINT('Ctrl Pts',(66.2678762584172,249.984083606643,22.7326069415889)) ;
#112207=CARTESIAN_POINT('Ctrl Pts',(66.2711429799946,249.994298745068,22.8125556966939)) ;
#112208=CARTESIAN_POINT('Ctrl Pts',(66.2744097015721,249.999567098801,22.8929928016749)) ;
#112209=CARTESIAN_POINT('Ctrl Pts',(66.2761239100128,250.002331661444,22.9352020812362)) ;
#112210=CARTESIAN_POINT('Ctrl Pts',(66.2778381184536,250.003734863383,22.9775455190962)) ;
#112211=CARTESIAN_POINT('Ctrl Pts',(66.2795523268944,250.003764624032,23.019942046258)) ;
#112212=CARTESIAN_POINT('',(66.7795523268961,250.003764452858,23.0229240588049)) ;
#112213=CARTESIAN_POINT('Ctrl Pts',(66.2795523269168,250.003764624032,23.0199420468122)) ;
#112214=CARTESIAN_POINT('Ctrl Pts',(66.2823406185767,250.003813031993,23.0889032537952)) ;
#112215=CARTESIAN_POINT('Ctrl Pts',(66.2851289102367,250.000224085711,23.1579109029645)) ;
#112216=CARTESIAN_POINT('Ctrl Pts',(66.2879172018966,249.993009685332,23.2265540271134)) ;
#112217=CARTESIAN_POINT('Ctrl Pts',(66.2907048552082,249.98579693661,23.2951814361853)) ;
#112218=CARTESIAN_POINT('Ctrl Pts',(66.2934925085199,249.974960433389,23.3634439989452)) ;
#112219=CARTESIAN_POINT('Ctrl Pts',(66.2962801618316,249.96056397712,23.4309354097307)) ;
#112220=CARTESIAN_POINT('Ctrl Pts',(66.2990681239764,249.946165925925,23.4984342976234)) ;
#112221=CARTESIAN_POINT('Ctrl Pts',(66.3018560861212,249.928207243678,23.565161385473)) ;
#112222=CARTESIAN_POINT('Ctrl Pts',(66.304644048266,249.906802553114,23.6307218657)) ;
#112223=CARTESIAN_POINT('Ctrl Pts',(66.3074350008797,249.885374903107,23.6963526684659)) ;
#112224=CARTESIAN_POINT('Ctrl Pts',(66.3102259534934,249.860494023033,23.7608139008159)) ;
#112225=CARTESIAN_POINT('Ctrl Pts',(66.3130169061071,249.83232367605,23.823728181203)) ;
#112226=CARTESIAN_POINT('Ctrl Pts',(66.3158096453554,249.804135295755,23.8866827363103)) ;
#112227=CARTESIAN_POINT('Ctrl Pts',(66.3186023846038,249.772653481735,23.9480879332316)) ;
#112228=CARTESIAN_POINT('Ctrl Pts',(66.3213951238522,249.738087949321,24.0075910207892)) ;
#112229=CARTESIAN_POINT('Ctrl Pts',(66.3241924149176,249.703466079395,24.0671910909663)) ;
#112230=CARTESIAN_POINT('Ctrl Pts',(66.326989705983,249.665750732254,24.124882458082)) ;
#112231=CARTESIAN_POINT('Ctrl Pts',(66.3297869970484,249.625194313814,24.1803421992117)) ;
#112232=CARTESIAN_POINT('Ctrl Pts',(66.3305368566942,249.614322502174,24.1952090903813)) ;
#112233=CARTESIAN_POINT('Ctrl Pts',(66.33128671634,249.603246748992,24.209915810732)) ;
#112234=CARTESIAN_POINT('Ctrl Pts',(66.3320365759858,249.591972378206,24.224456577295)) ;
#112235=CARTESIAN_POINT('Ctrl Pts',(66.3348408832902,249.549808753952,24.2788357909423)) ;
#112236=CARTESIAN_POINT('Ctrl Pts',(66.3376451905946,249.504706239201,24.3310951425113)) ;
#112237=CARTESIAN_POINT('Ctrl Pts',(66.340449497899,249.456905656582,24.3809018253054)) ;
#112238=CARTESIAN_POINT('Ctrl Pts',(66.3433206526994,249.407965630633,24.4318957717145)) ;
#112239=CARTESIAN_POINT('Ctrl Pts',(66.3461918074997,249.356197496886,24.4803181537219)) ;
#112240=CARTESIAN_POINT('Ctrl Pts',(66.3490629623001,249.30190518708,24.525845704037)) ;
#112241=CARTESIAN_POINT('Ctrl Pts',(66.3518601597058,249.249011379988,24.5702005209955)) ;
#112242=CARTESIAN_POINT('Ctrl Pts',(66.3546573571116,249.193722271344,24.6118075141096)) ;
#112243=CARTESIAN_POINT('Ctrl Pts',(66.3574545545173,249.136356249685,24.6504048897544)) ;
#112244=CARTESIAN_POINT('Ctrl Pts',(66.3602501735027,249.079022598889,24.6889804854265)) ;
#112245=CARTESIAN_POINT('Ctrl Pts',(66.363045792488,249.019614764495,24.7245495622709)) ;
#112246=CARTESIAN_POINT('Ctrl Pts',(66.3658414114734,248.958481971273,24.7568923073823)) ;
#112247=CARTESIAN_POINT('Ctrl Pts',(66.3686363904332,248.897363173718,24.7892276479856)) ;
#112248=CARTESIAN_POINT('Ctrl Pts',(66.371431369393,248.834520632473,24.8183378962952)) ;
#112249=CARTESIAN_POINT('Ctrl Pts',(66.3742263483528,248.77032861088,24.8440489386746)) ;
#112250=CARTESIAN_POINT('Ctrl Pts',(66.3771539204158,248.70309133583,24.8709797064767)) ;
#112251=CARTESIAN_POINT('Ctrl Pts',(66.3800814924787,248.634373877362,24.8941804696978)) ;
#112252=CARTESIAN_POINT('Ctrl Pts',(66.3830090645416,248.564628171981,24.9135083962933)) ;
#112253=CARTESIAN_POINT('Ctrl Pts',(66.3858072864145,248.497964071442,24.9319823486997)) ;
#112254=CARTESIAN_POINT('Ctrl Pts',(66.3886055082874,248.430361183098,24.9469184298629)) ;
#112255=CARTESIAN_POINT('Ctrl Pts',(66.3914037301603,248.362225891714,24.958244065241)) ;
#112256=CARTESIAN_POINT('Ctrl Pts',(66.3942037549716,248.294046699689,24.9695769979045)) ;
#112257=CARTESIAN_POINT('Ctrl Pts',(66.3970037797829,248.225334905901,24.9772948007852)) ;
#112258=CARTESIAN_POINT('Ctrl Pts',(66.3998038045943,248.156501811782,24.9813767913805)) ;
#112259=CARTESIAN_POINT('Ctrl Pts',(66.4026081288559,248.087563024148,24.98546504989)) ;
#112260=CARTESIAN_POINT('Ctrl Pts',(66.4054124531175,248.018503050828,24.9859063585669)) ;
#112261=CARTESIAN_POINT('Ctrl Pts',(66.4082167773791,247.949731898289,24.9827320769746)) ;
#112262=CARTESIAN_POINT('Ctrl Pts',(66.4085969226221,247.940409500431,24.9823017814972)) ;
#112263=CARTESIAN_POINT('Ctrl Pts',(66.408977067865,247.931092398573,24.9818051247597)) ;
#112264=CARTESIAN_POINT('Ctrl Pts',(66.409357213108,247.921781601908,24.9812422575232)) ;
#112265=CARTESIAN_POINT('Ctrl Pts',(66.4121615246675,247.853096342257,24.9770900153815)) ;
#112266=CARTESIAN_POINT('Ctrl Pts',(66.414965836227,247.784504331069,24.9693152890603)) ;
#112267=CARTESIAN_POINT('Ctrl Pts',(66.4177701477865,247.716416217242,24.9579292731304)) ;
#112268=CARTESIAN_POINT('Ctrl Pts',(66.4206413020549,247.646705176046,24.9462718636219)) ;
#112269=CARTESIAN_POINT('Ctrl Pts',(66.4235124563234,247.577522881246,24.930828737212)) ;
#112270=CARTESIAN_POINT('Ctrl Pts',(66.4263836105919,247.509307690899,24.9116685843483)) ;
#112271=CARTESIAN_POINT('Ctrl Pts',(66.4291808136461,247.442849492929,24.8930019321602)) ;
#112272=CARTESIAN_POINT('Ctrl Pts',(66.4319780167002,247.377309680021,24.8708075687004)) ;
#112273=CARTESIAN_POINT('Ctrl Pts',(66.4347752197543,247.313083999177,24.8452007906509)) ;
#112274=CARTESIAN_POINT('Ctrl Pts',(66.4375708448837,247.248894548556,24.819608457591)) ;
#112275=CARTESIAN_POINT('Ctrl Pts',(66.4403664700131,247.186018210787,24.7906077102002)) ;
#112276=CARTESIAN_POINT('Ctrl Pts',(66.4431620951424,247.124833453977,24.7583629847186)) ;
#112277=CARTESIAN_POINT('Ctrl Pts',(66.4459570807273,247.063662694172,24.7261256357403)) ;
#112278=CARTESIAN_POINT('Ctrl Pts',(66.4487520663121,247.004183177623,24.6906460100167)) ;
#112279=CARTESIAN_POINT('Ctrl Pts',(66.4515470518969,246.946749753233,24.6521349925484)) ;
#112280=CARTESIAN_POINT('Ctrl Pts',(66.4544746184247,246.886591957883,24.6117971939199)) ;
#112281=CARTESIAN_POINT('Ctrl Pts',(66.4574021849525,246.8286797056,24.5681335426055)) ;
#112282=CARTESIAN_POINT('Ctrl Pts',(66.4603297514802,246.77338581049,24.5214367044075)) ;
#112283=CARTESIAN_POINT('Ctrl Pts',(66.463127981089,246.720534743567,24.4768028851435)) ;
#112284=CARTESIAN_POINT('Ctrl Pts',(66.4659262106978,246.670075887954,24.4293986300107)) ;
#112285=CARTESIAN_POINT('Ctrl Pts',(66.4687244403066,246.622298354367,24.379518611928)) ;
#112286=CARTESIAN_POINT('Ctrl Pts',(66.4715244732278,246.574490030663,24.3296064487869)) ;
#112287=CARTESIAN_POINT('Ctrl Pts',(66.474324506149,246.529366785742,24.2772157164121)) ;
#112288=CARTESIAN_POINT('Ctrl Pts',(66.4771245390702,246.487177649648,24.2226744118407)) ;
#112289=CARTESIAN_POINT('Ctrl Pts',(66.479928871907,246.444923725129,24.1680493500373)) ;
#112290=CARTESIAN_POINT('Ctrl Pts',(66.4827332047438,246.405613172611,24.111267529043)) ;
#112291=CARTESIAN_POINT('Ctrl Pts',(66.4855375375806,246.369451314658,24.0526852250122)) ;
#112292=CARTESIAN_POINT('Ctrl Pts',(66.4859176417971,246.364549872681,24.0447448762482)) ;
#112293=CARTESIAN_POINT('Ctrl Pts',(66.4862977460136,246.35970620678,24.0367714842076)) ;
#112294=CARTESIAN_POINT('Ctrl Pts',(66.4866778502301,246.354920761433,24.0287659670131)) ;
#112295=CARTESIAN_POINT('Ctrl Pts',(66.4894819430555,246.319617725101,23.9697079183149)) ;
#112296=CARTESIAN_POINT('Ctrl Pts',(66.4922860358808,246.287358211815,23.9086841781292)) ;
#112297=CARTESIAN_POINT('Ctrl Pts',(66.4950901287062,246.258364562065,23.8460401112139)) ;
#112298=CARTESIAN_POINT('Ctrl Pts',(66.4979613103164,246.228677230311,23.7818972656948)) ;
#112299=CARTESIAN_POINT('Ctrl Pts',(66.5008324919267,246.202414393297,23.716055954698)) ;
#112300=CARTESIAN_POINT('Ctrl Pts',(66.5037036735369,246.17976658824,23.6489169566531)) ;
#112301=CARTESIAN_POINT('Ctrl Pts',(66.5065006566966,246.15770405861,23.5835129967578)) ;
#112302=CARTESIAN_POINT('Ctrl Pts',(66.5092976398563,246.139072137996,23.5168781045418)) ;
#112303=CARTESIAN_POINT('Ctrl Pts',(66.512094623016,246.123998794174,23.449404056535)) ;
#112304=CARTESIAN_POINT('Ctrl Pts',(66.5148900284519,246.108933952931,23.3819680693253)) ;
#112305=CARTESIAN_POINT('Ctrl Pts',(66.5176854338878,246.097423811082,23.3136943405699)) ;
#112306=CARTESIAN_POINT('Ctrl Pts',(66.5204808393238,246.0895460126,23.2449880919614)) ;
#112307=CARTESIAN_POINT('Ctrl Pts',(66.5232756057897,246.081670014814,23.1762975481341)) ;
#112308=CARTESIAN_POINT('Ctrl Pts',(66.5260703722556,246.077424766582,23.1071751649751)) ;
#112309=CARTESIAN_POINT('Ctrl Pts',(66.5288651387215,246.076836234115,23.0380328548493)) ;
#112310=CARTESIAN_POINT('Ctrl Pts',(66.5317929177741,246.076219691355,22.9655998234315)) ;
#112311=CARTESIAN_POINT('Ctrl Pts',(66.5347206968267,246.079616675261,22.8931455006518)) ;
#112312=CARTESIAN_POINT('Ctrl Pts',(66.5376484758792,246.086995729267,22.8211429598744)) ;
#112313=CARTESIAN_POINT('Ctrl Pts',(66.5404464903734,246.094047730012,22.7523317042792)) ;
#112314=CARTESIAN_POINT('Ctrl Pts',(66.5432445048676,246.104736141785,22.6839335251056)) ;
#112315=CARTESIAN_POINT('Ctrl Pts',(66.5460425193617,246.118980656983,22.6163532966271)) ;
#112316=CARTESIAN_POINT('Ctrl Pts',(66.5488423387544,246.133234360804,22.5487294745744)) ;
#112317=CARTESIAN_POINT('Ctrl Pts',(66.5516421581471,246.151048607749,22.4819251239235)) ;
#112318=CARTESIAN_POINT('Ctrl Pts',(66.5544419775398,246.172292968435,22.4163308092623)) ;
#112319=CARTESIAN_POINT('Ctrl Pts',(66.5572461005754,246.193569984136,22.350635668628)) ;
#112320=CARTESIAN_POINT('Ctrl Pts',(66.5600502236111,246.218287455024,22.2861547275074)) ;
#112321=CARTESIAN_POINT('Ctrl Pts',(66.5628543466468,246.246266951478,22.2232584003724)) ;
#112322=CARTESIAN_POINT('Ctrl Pts',(66.563235726882,246.25007235759,22.2147040624463)) ;
#112323=CARTESIAN_POINT('Ctrl Pts',(66.5636171071171,246.253938035722,22.2061789975571)) ;
#112324=CARTESIAN_POINT('Ctrl Pts',(66.5639984873523,246.257863473067,22.1976840994865)) ;
#112325=CARTESIAN_POINT('Ctrl Pts',(66.56680310456,246.286730593358,22.1352138005322)) ;
#112326=CARTESIAN_POINT('Ctrl Pts',(66.5696077217676,246.318938468299,22.0741490763927)) ;
#112327=CARTESIAN_POINT('Ctrl Pts',(66.5724123389752,246.354327170167,22.0148683971174)) ;
#112328=CARTESIAN_POINT('Ctrl Pts',(66.5752834550377,246.39055495558,21.95418214375)) ;
#112329=CARTESIAN_POINT('Ctrl Pts',(66.5781545711002,246.430116201379,21.8953661229176)) ;
#112330=CARTESIAN_POINT('Ctrl Pts',(66.5810256871627,246.472787424797,21.838803551572)) ;
#112331=CARTESIAN_POINT('Ctrl Pts',(66.5838231904591,246.51436459743,21.7836911923528)) ;
#112332=CARTESIAN_POINT('Ctrl Pts',(66.5866206937555,246.558893868519,21.7307185269278)) ;
#112333=CARTESIAN_POINT('Ctrl Pts',(66.589418197052,246.60612377853,21.6802122577885)) ;
#112334=CARTESIAN_POINT('Ctrl Pts',(66.5922141195746,246.653327000528,21.6297345280219)) ;
#112335=CARTESIAN_POINT('Ctrl Pts',(66.5950100420972,246.703227500808,21.581720784043)) ;
#112336=CARTESIAN_POINT('Ctrl Pts',(66.5978059646198,246.755534338094,21.5364637513572)) ;
#112337=CARTESIAN_POINT('Ctrl Pts',(66.6006012442589,246.807829148151,21.4912171248968)) ;
#112338=CARTESIAN_POINT('Ctrl Pts',(66.603396523898,246.862528827727,21.4487262692637)) ;
#112339=CARTESIAN_POINT('Ctrl Pts',(66.6061918035371,246.919307766271,21.409245007695)) ;
#112340=CARTESIAN_POINT('Ctrl Pts',(66.6091190802819,246.978767887565,21.367899384442)) ;
#112341=CARTESIAN_POINT('Ctrl Pts',(66.6120463570266,247.040508054616,21.3298549997475)) ;
#112342=CARTESIAN_POINT('Ctrl Pts',(66.6149736337714,247.104120186999,21.2953525172994)) ;
#112343=CARTESIAN_POINT('Ctrl Pts',(66.617772145689,247.164934153733,21.2623677274298)) ;
#112344=CARTESIAN_POINT('Ctrl Pts',(66.6205706576066,247.227458366892,21.2326199408459)) ;
#112345=CARTESIAN_POINT('Ctrl Pts',(66.6233691695242,247.291313095359,21.2062712717487)) ;
#112346=CARTESIAN_POINT('Ctrl Pts',(66.6261694804375,247.355208872207,21.1799056646699)) ;
#112347=CARTESIAN_POINT('Ctrl Pts',(66.6289697913508,247.420436407318,21.1569436854979)) ;
#112348=CARTESIAN_POINT('Ctrl Pts',(66.6317701022641,247.48659950903,21.1374979913317)) ;
#112349=CARTESIAN_POINT('Ctrl Pts',(66.6345747050863,247.552864015911,21.1180224936366)) ;
#112350=CARTESIAN_POINT('Ctrl Pts',(66.6373793079084,247.620066476324,21.1020741416477)) ;
#112351=CARTESIAN_POINT('Ctrl Pts',(66.6401839107306,247.687800256479,21.089714592224)) ;
#112352=CARTESIAN_POINT('Ctrl Pts',(66.6405623153119,247.696939080884,21.0880470084621)) ;
#112353=CARTESIAN_POINT('Ctrl Pts',(66.6409407198932,247.706087571098,21.0864446783601)) ;
#112354=CARTESIAN_POINT('Ctrl Pts',(66.6413191244745,247.715244723888,21.084907680915)) ;
#112355=CARTESIAN_POINT('Ctrl Pts',(66.6441234978784,247.78310879586,21.0735169235878)) ;
#112356=CARTESIAN_POINT('Ctrl Pts',(66.6469278712823,247.8516960402,21.0656772442205)) ;
#112357=CARTESIAN_POINT('Ctrl Pts',(66.6497322446863,247.920603762888,21.0614699889312)) ;
#112358=CARTESIAN_POINT('Ctrl Pts',(66.6526033912242,247.991152203105,21.0571625573883)) ;
#112359=CARTESIAN_POINT('Ctrl Pts',(66.6554745377622,248.062036086872,21.0566629239467)) ;
#112360=CARTESIAN_POINT('Ctrl Pts',(66.6583456843001,248.132812836757,21.060002631443)) ;
#112361=CARTESIAN_POINT('Ctrl Pts',(66.66114295754,248.201768532974,21.0632564097804)) ;
#112362=CARTESIAN_POINT('Ctrl Pts',(66.66394023078,248.270622022945,21.0701543075325)) ;
#112363=CARTESIAN_POINT('Ctrl Pts',(66.6667375040199,248.338961748443,21.0806728828239)) ;
#112364=CARTESIAN_POINT('Ctrl Pts',(66.6695332021673,248.407262993113,21.0911855353011)) ;
#112365=CARTESIAN_POINT('Ctrl Pts',(66.6723289003146,248.475050566595,21.1053147454544)) ;
#112366=CARTESIAN_POINT('Ctrl Pts',(66.675124598462,248.541918708859,21.1229853060779)) ;
#112367=CARTESIAN_POINT('Ctrl Pts',(66.6779196597248,248.608771617973,21.1406518411926)) ;
#112368=CARTESIAN_POINT('Ctrl Pts',(66.6807147209876,248.674705040942,21.1618579997019)) ;
#112369=CARTESIAN_POINT('Ctrl Pts',(66.6835097822504,248.739325798165,21.1864780066908)) ;
#112370=CARTESIAN_POINT('Ctrl Pts',(66.6864372805292,248.807008449014,21.2122645713879)) ;
#112371=CARTESIAN_POINT('Ctrl Pts',(66.6893647788081,248.873250389559,21.2417963754347)) ;
#112372=CARTESIAN_POINT('Ctrl Pts',(66.692292277087,248.937622622676,21.2748720218303)) ;
#112373=CARTESIAN_POINT('Ctrl Pts',(66.6950905879347,248.999154176604,21.3064880746122)) ;
#112374=CARTESIAN_POINT('Ctrl Pts',(66.6978888987824,249.058977155078,21.3413414730132)) ;
#112375=CARTESIAN_POINT('Ctrl Pts',(66.7006872096301,249.116743609473,21.379210028932)) ;
#112376=CARTESIAN_POINT('Ctrl Pts',(66.7034873255982,249.174547327564,21.4171030129107)) ;
#112377=CARTESIAN_POINT('Ctrl Pts',(66.7062874415664,249.230291488826,21.4580147371391)) ;
#112378=CARTESIAN_POINT('Ctrl Pts',(66.7090875575346,249.283659712831,21.5016815357681)) ;
#112379=CARTESIAN_POINT('Ctrl Pts',(66.7118919753153,249.337109926331,21.545415419612)) ;
#112380=CARTESIAN_POINT('Ctrl Pts',(66.7146963930959,249.38817656324,21.5919124921997)) ;
#112381=CARTESIAN_POINT('Ctrl Pts',(66.7175008108766,249.436579478484,21.6408717106214)) ;
#112382=CARTESIAN_POINT('Ctrl Pts',(66.7178804611166,249.443132060812,21.6474996029249)) ;
#112383=CARTESIAN_POINT('Ctrl Pts',(66.7182601113567,249.449635886879,21.6541725687552)) ;
#112384=CARTESIAN_POINT('Ctrl Pts',(66.7186397615967,249.456090319567,21.6608898162314)) ;
#112385=CARTESIAN_POINT('Ctrl Pts',(66.72140456754,249.503094777811,21.709808225302)) ;
#112386=CARTESIAN_POINT('Ctrl Pts',(66.7241693734833,249.54765892548,21.7612677748274)) ;
#112387=CARTESIAN_POINT('Ctrl Pts',(66.7269341794266,249.589492264482,21.8149922509759)) ;
#112388=CARTESIAN_POINT('Ctrl Pts',(66.7296954263439,249.631271753071,21.8686475697182)) ;
#112389=CARTESIAN_POINT('Ctrl Pts',(66.7324566732612,249.670327093644,21.9245616439305)) ;
#112390=CARTESIAN_POINT('Ctrl Pts',(66.7352179201785,249.706405216602,21.9824221831053)) ;
#112391=CARTESIAN_POINT('Ctrl Pts',(66.7379766065846,249.742449884226,22.0402290680572)) ;
#112392=CARTESIAN_POINT('Ctrl Pts',(66.7407352929908,249.775522543469,22.0999784146441)) ;
#112393=CARTESIAN_POINT('Ctrl Pts',(66.7434939793969,249.805412160736,22.1613272439004)) ;
#112394=CARTESIAN_POINT('Ctrl Pts',(66.7462511002973,249.835284816175,22.2226412587823)) ;
#112395=CARTESIAN_POINT('Ctrl Pts',(66.7490082211978,249.861977794241,22.285552504173)) ;
#112396=CARTESIAN_POINT('Ctrl Pts',(66.7517653420982,249.885325908284,22.3496932949189)) ;
#112397=CARTESIAN_POINT('Ctrl Pts',(66.7545228691849,249.908677462033,22.4138435350553)) ;
#112398=CARTESIAN_POINT('Ctrl Pts',(66.7572803962717,249.928682984491,22.4792232138235)) ;
#112399=CARTESIAN_POINT('Ctrl Pts',(66.7600379233585,249.94522595852,22.5454459828584)) ;
#112400=CARTESIAN_POINT('Ctrl Pts',(66.7627957000588,249.961770430031,22.6116747464332)) ;
#112401=CARTESIAN_POINT('Ctrl Pts',(66.7655534767592,249.974851620613,22.6787462610508)) ;
#112402=CARTESIAN_POINT('Ctrl Pts',(66.7683112534596,249.984403886993,22.7462627910657)) ;
#112403=CARTESIAN_POINT('Ctrl Pts',(66.7710716188912,249.993965120107,22.8138426989994)) ;
#112404=CARTESIAN_POINT('Ctrl Pts',(66.7738319843228,249.999990765927,22.8818679558387)) ;
#112405=CARTESIAN_POINT('Ctrl Pts',(66.7765923497544,250.002467061614,22.9499358747035)) ;
#112406=CARTESIAN_POINT('Ctrl Pts',(66.7775790088016,250.003352183386,22.9742659243427)) ;
#112407=CARTESIAN_POINT('Ctrl Pts',(66.7785656678489,250.003784318705,22.9986014255071)) ;
#112408=CARTESIAN_POINT('Ctrl Pts',(66.7795523268961,250.003764452858,23.0229240588049)) ;
#112409=CARTESIAN_POINT('',(66.9402651077866,247.187420265513,24.7899322074257)) ;
#112410=CARTESIAN_POINT('Ctrl Pts',(66.7795523269168,250.003764452857,23.0229240593157)) ;
#112411=CARTESIAN_POINT('Ctrl Pts',(66.7833403875917,250.003688182277,23.1163054669723)) ;
#112412=CARTESIAN_POINT('Ctrl Pts',(66.7871284482667,249.996946522773,23.2094191785349)) ;
#112413=CARTESIAN_POINT('Ctrl Pts',(66.7909165089416,249.983675392804,23.3014787167803)) ;
#112414=CARTESIAN_POINT('Ctrl Pts',(66.7925978055341,249.977785121368,23.3423385131858)) ;
#112415=CARTESIAN_POINT('Ctrl Pts',(66.7942791021265,249.970609197882,23.3829909913529)) ;
#112416=CARTESIAN_POINT('Ctrl Pts',(66.7959603987189,249.962162427064,23.4233687786404)) ;
#112417=CARTESIAN_POINT('Ctrl Pts',(66.7987684406399,249.948054930112,23.4908063264787)) ;
#112418=CARTESIAN_POINT('Ctrl Pts',(66.8015764825609,249.930368358597,23.5576217364157)) ;
#112419=CARTESIAN_POINT('Ctrl Pts',(66.8043845244819,249.909174104639,23.6234095491443)) ;
#112420=CARTESIAN_POINT('Ctrl Pts',(66.8072552124552,249.887507017163,23.6906650560432)) ;
#112421=CARTESIAN_POINT('Ctrl Pts',(66.8101259004285,249.862173867243,23.7568460432548)) ;
#112422=CARTESIAN_POINT('Ctrl Pts',(66.8129965884018,249.833306360801,23.8215298879838)) ;
#112423=CARTESIAN_POINT('Ctrl Pts',(66.8157975052758,249.80514046933,23.8846416137651)) ;
#112424=CARTESIAN_POINT('Ctrl Pts',(66.8185984221498,249.773610291121,23.9463276776076)) ;
#112425=CARTESIAN_POINT('Ctrl Pts',(66.8213993390237,249.738887943492,24.0062125772683)) ;
#112426=CARTESIAN_POINT('Ctrl Pts',(66.8241986612997,249.704185363741,24.0660633836856)) ;
#112427=CARTESIAN_POINT('Ctrl Pts',(66.8269979835757,249.666294464709,24.1241146414449)) ;
#112428=CARTESIAN_POINT('Ctrl Pts',(66.8297973058516,249.625433461131,24.1800151012739)) ;
#112429=CARTESIAN_POINT('Ctrl Pts',(66.8325959657634,249.584582125916,24.2359023341646)) ;
#112430=CARTESIAN_POINT('Ctrl Pts',(66.8353946256752,249.540762368943,24.2896393879892)) ;
#112431=CARTESIAN_POINT('Ctrl Pts',(66.838193285587,249.494234927956,24.3409051312997)) ;
#112432=CARTESIAN_POINT('Ctrl Pts',(66.8411172647748,249.445624066544,24.3944664682303)) ;
#112433=CARTESIAN_POINT('Ctrl Pts',(66.8440412439626,249.394057673407,24.4453295090004)) ;
#112434=CARTESIAN_POINT('Ctrl Pts',(66.8469652231504,249.339877448202,24.4931695255883)) ;
#112435=CARTESIAN_POINT('Ctrl Pts',(66.8497670277675,249.287961071449,24.5390106108855)) ;
#112436=CARTESIAN_POINT('Ctrl Pts',(66.8525688323846,249.233645384136,24.582076004081)) ;
#112437=CARTESIAN_POINT('Ctrl Pts',(66.8553706370016,249.177264424868,24.6221216438323)) ;
#112438=CARTESIAN_POINT('Ctrl Pts',(66.8581742072453,249.120847935742,24.6621925193357)) ;
#112439=CARTESIAN_POINT('Ctrl Pts',(66.860977777489,249.062363994278,24.6992395936262)) ;
#112440=CARTESIAN_POINT('Ctrl Pts',(66.8637813477326,249.002173853502,24.7330632608564)) ;
#112441=CARTESIAN_POINT('Ctrl Pts',(66.8665891405139,248.941893058629,24.7669378708818)) ;
#112442=CARTESIAN_POINT('Ctrl Pts',(66.8693969332951,248.879901373507,24.7975791757488)) ;
#112443=CARTESIAN_POINT('Ctrl Pts',(66.8722047260763,248.816581757081,24.8248348874507)) ;
#112444=CARTESIAN_POINT('Ctrl Pts',(66.8725634959978,248.808490998401,24.8283175267732)) ;
#112445=CARTESIAN_POINT('Ctrl Pts',(66.8729222659194,248.800378580186,24.8317449564989)) ;
#112446=CARTESIAN_POINT('Ctrl Pts',(66.8732810358409,248.792245318936,24.8351169176106)) ;
#112447=CARTESIAN_POINT('Ctrl Pts',(66.8760720388387,248.728973692283,24.8613486416366)) ;
#112448=CARTESIAN_POINT('Ctrl Pts',(66.8788630418364,248.664195049807,24.8843205322089)) ;
#112449=CARTESIAN_POINT('Ctrl Pts',(66.8816540448341,248.59828361459,24.9038578853005)) ;
#112450=CARTESIAN_POINT('Ctrl Pts',(66.8844124564412,248.533141847243,24.9231670947795)) ;
#112451=CARTESIAN_POINT('Ctrl Pts',(66.8871708680483,248.466894088193,24.9391213768116)) ;
#112452=CARTESIAN_POINT('Ctrl Pts',(66.8899292796554,248.399922967563,24.9515997207226)) ;
#112453=CARTESIAN_POINT('Ctrl Pts',(66.8926852815423,248.333010352218,24.9640671636802)) ;
#112454=CARTESIAN_POINT('Ctrl Pts',(66.8954412834293,248.265376120888,24.9730645956052)) ;
#112455=CARTESIAN_POINT('Ctrl Pts',(66.8981972853162,248.197416078765,24.9785213609108)) ;
#112456=CARTESIAN_POINT('Ctrl Pts',(66.9009518753248,248.129490852044,24.9839753307578)) ;
#112457=CARTESIAN_POINT('Ctrl Pts',(66.9037064653333,248.061240646926,24.9858921916273)) ;
#112458=CARTESIAN_POINT('Ctrl Pts',(66.9064610553419,247.993067466502,24.9842530048237)) ;
#112459=CARTESIAN_POINT('Ctrl Pts',(66.9092780597123,247.923349596837,24.9825766768128)) ;
#112460=CARTESIAN_POINT('Ctrl Pts',(66.9120950640826,247.853712829984,24.9771811257619)) ;
#112461=CARTESIAN_POINT('Ctrl Pts',(66.914912068453,247.784586283387,24.9681024548278)) ;
#112462=CARTESIAN_POINT('Ctrl Pts',(66.9176681774467,247.71695405009,24.9592200381461)) ;
#112463=CARTESIAN_POINT('Ctrl Pts',(66.9204242864404,247.649810699675,24.9468122973506)) ;
#112464=CARTESIAN_POINT('Ctrl Pts',(66.923180395434,247.583549651707,24.930965138326)) ;
#112465=CARTESIAN_POINT('Ctrl Pts',(66.9260278474928,247.515092577662,24.9145927721772)) ;
#112466=CARTESIAN_POINT('Ctrl Pts',(66.9288752995515,247.447577886713,24.8945491173228)) ;
#112467=CARTESIAN_POINT('Ctrl Pts',(66.9317227516103,247.381421698607,24.8709845325901)) ;
#112468=CARTESIAN_POINT('Ctrl Pts',(66.9345702036691,247.315265510502,24.8474199478574)) ;
#112469=CARTESIAN_POINT('Ctrl Pts',(66.9374176557278,247.250468345473,24.8203347117332)) ;
#112470=CARTESIAN_POINT('Ctrl Pts',(66.9402651077866,247.187420265513,24.7899322074257)) ;
#112471=CARTESIAN_POINT('',(66.9402651077866,247.154495177753,24.7736741551653)) ;
#112472=CARTESIAN_POINT('Ctrl Pts',(66.9402651077866,247.187420265513,24.7899322074257)) ;
#112473=CARTESIAN_POINT('Ctrl Pts',(66.9402651077866,247.176445236259,24.7845128566722)) ;
#112474=CARTESIAN_POINT('Ctrl Pts',(66.9402651077866,247.165470207006,24.7790935059188)) ;
#112475=CARTESIAN_POINT('Ctrl Pts',(66.9402651077866,247.154495177753,24.7736741551653)) ;
#112476=CARTESIAN_POINT('',(66.9402651077866,248.892162375845,24.7903888257488)) ;
#112477=CARTESIAN_POINT('Origin',(66.9402651077866,248.040265107786,23.0213203435596)) ;
#112478=CARTESIAN_POINT('',(66.8509778886564,250.003764893262,23.0222381855048)) ;
#112479=CARTESIAN_POINT('Ctrl Pts',(66.9402651077866,248.892162375845,24.7903888257488)) ;
#112480=CARTESIAN_POINT('Ctrl Pts',(66.9144915620792,249.465128147431,24.5144764004134)) ;
#112481=CARTESIAN_POINT('Ctrl Pts',(66.8847291557025,249.954933534302,23.8517629624628)) ;
#112482=CARTESIAN_POINT('Ctrl Pts',(66.8549667493257,250.005277703762,23.1203925250327)) ;
#112483=CARTESIAN_POINT('Ctrl Pts',(66.8509778886564,250.00450609953,23.0222385319832)) ;
#112484=CARTESIAN_POINT('',(66.3509778886297,250.003764831718,23.0202791324881)) ;
#112485=CARTESIAN_POINT('Ctrl Pts',(66.8509778886564,250.003764893262,23.0222381855048)) ;
#112486=CARTESIAN_POINT('Ctrl Pts',(66.8482267036004,250.003796526989,22.9545655163395)) ;
#112487=CARTESIAN_POINT('Ctrl Pts',(66.8454755185445,250.000325357658,22.8867680494306)) ;
#112488=CARTESIAN_POINT('Ctrl Pts',(66.8427243334885,249.993338983009,22.8192443976375)) ;
#112489=CARTESIAN_POINT('Ctrl Pts',(66.8399758974318,249.986359589185,22.7517882158492)) ;
#112490=CARTESIAN_POINT('Ctrl Pts',(66.8372274613752,249.975872000238,22.6846058083517)) ;
#112491=CARTESIAN_POINT('Ctrl Pts',(66.8344790253185,249.961915836364,22.6180949384146)) ;
#112492=CARTESIAN_POINT('Ctrl Pts',(66.831732330507,249.947968514284,22.5516262057995)) ;
#112493=CARTESIAN_POINT('Ctrl Pts',(66.8289856356955,249.930557076584,22.4858286624589)) ;
#112494=CARTESIAN_POINT('Ctrl Pts',(66.8262389408841,249.90977260833,22.4210920908021)) ;
#112495=CARTESIAN_POINT('Ctrl Pts',(66.8234929821263,249.888993709856,22.3563728671186)) ;
#112496=CARTESIAN_POINT('Ctrl Pts',(66.8207470233684,249.864843729529,22.2927145333732)) ;
#112497=CARTESIAN_POINT('Ctrl Pts',(66.8180010646106,249.837463659151,22.2304919064297)) ;
#112498=CARTESIAN_POINT('Ctrl Pts',(66.815252997896,249.810062570247,22.1682215137992)) ;
#112499=CARTESIAN_POINT('Ctrl Pts',(66.8125049311814,249.779426638707,22.1073894964761)) ;
#112500=CARTESIAN_POINT('Ctrl Pts',(66.8097568644668,249.745744629783,22.0483497119119)) ;
#112501=CARTESIAN_POINT('Ctrl Pts',(66.8070078405071,249.712050888268,21.9892893617802)) ;
#112502=CARTESIAN_POINT('Ctrl Pts',(66.8042588165472,249.675309229075,21.9320229161002)) ;
#112503=CARTESIAN_POINT('Ctrl Pts',(66.8015097925875,249.635752384316,21.8768761114409)) ;
#112504=CARTESIAN_POINT('Ctrl Pts',(66.7987559331582,249.596125959985,21.8216323048304)) ;
#112505=CARTESIAN_POINT('Ctrl Pts',(66.796002073729,249.553674774807,21.7685159848195)) ;
#112506=CARTESIAN_POINT('Ctrl Pts',(66.7932482142998,249.508672063172,21.7178199548472)) ;
#112507=CARTESIAN_POINT('Ctrl Pts',(66.7907067540473,249.467140312619,21.6710339991927)) ;
#112508=CARTESIAN_POINT('Ctrl Pts',(66.7881652937948,249.423436103688,21.6263092066677)) ;
#112509=CARTESIAN_POINT('Ctrl Pts',(66.7856238335423,249.377799747824,21.5838457049321)) ;
#112510=CARTESIAN_POINT('Ctrl Pts',(66.7828201544163,249.327454794291,21.5370009693849)) ;
#112511=CARTESIAN_POINT('Ctrl Pts',(66.7800164752903,249.274551903111,21.4927167710767)) ;
#112512=CARTESIAN_POINT('Ctrl Pts',(66.7772127961643,249.219381460994,21.4512831224729)) ;
#112513=CARTESIAN_POINT('Ctrl Pts',(66.7743415628416,249.162881695966,21.4088511367836)) ;
#112514=CARTESIAN_POINT('Ctrl Pts',(66.771470329519,249.104004001477,21.369409270451)) ;
#112515=CARTESIAN_POINT('Ctrl Pts',(66.7685990961963,249.043099853033,21.3332283070507)) ;
#112516=CARTESIAN_POINT('Ctrl Pts',(66.7658027497716,248.983784193659,21.2979910078564)) ;
#112517=CARTESIAN_POINT('Ctrl Pts',(66.7630064033468,248.922546947128,21.2658468506903)) ;
#112518=CARTESIAN_POINT('Ctrl Pts',(66.7602100569221,248.85974380801,21.2370034126644)) ;
#112519=CARTESIAN_POINT('Ctrl Pts',(66.7574153681327,248.79697789772,21.208177072628)) ;
#112520=CARTESIAN_POINT('Ctrl Pts',(66.7546206793433,248.732648379345,21.1826477722248)) ;
#112521=CARTESIAN_POINT('Ctrl Pts',(66.7518259905539,248.66713472333,21.160576746202)) ;
#112522=CARTESIAN_POINT('Ctrl Pts',(66.7490320186323,248.601637872276,21.1385113816357)) ;
#112523=CARTESIAN_POINT('Ctrl Pts',(66.7462380467108,248.534957949055,21.1199026851751)) ;
#112524=CARTESIAN_POINT('Ctrl Pts',(66.7434440747892,248.467491879638,21.1048627950048)) ;
#112525=CARTESIAN_POINT('Ctrl Pts',(66.7405156682585,248.396779616297,21.089099246253)) ;
#112526=CARTESIAN_POINT('Ctrl Pts',(66.7375872617277,248.325204202411,21.0772567738979)) ;
#112527=CARTESIAN_POINT('Ctrl Pts',(66.7346588551969,248.253235180171,21.0694043622048)) ;
#112528=CARTESIAN_POINT('Ctrl Pts',(66.7318618178326,248.184494709143,21.0619042119778)) ;
#112529=CARTESIAN_POINT('Ctrl Pts',(66.7290647804682,248.115395702809,21.0580437680177)) ;
#112530=CARTESIAN_POINT('Ctrl Pts',(66.7262677431038,248.046350626325,21.0578297740727)) ;
#112531=CARTESIAN_POINT('Ctrl Pts',(66.7234689624468,247.977262516533,21.0576156467529)) ;
#112532=CARTESIAN_POINT('Ctrl Pts',(66.7206701817898,247.908228890469,21.0610524685653)) ;
#112533=CARTESIAN_POINT('Ctrl Pts',(66.7178714011328,247.839658797962,21.0680949703733)) ;
#112534=CARTESIAN_POINT('Ctrl Pts',(66.7150683953953,247.770985191034,21.0751481036457)) ;
#112535=CARTESIAN_POINT('Ctrl Pts',(66.7122653896578,247.702776994151,21.0858176978745)) ;
#112536=CARTESIAN_POINT('Ctrl Pts',(66.7094623839203,247.635433671554,21.1000073138222)) ;
#112537=CARTESIAN_POINT('Ctrl Pts',(66.7090759880869,247.626150358677,21.1019633599361)) ;
#112538=CARTESIAN_POINT('Ctrl Pts',(66.7086895922535,247.616883456562,21.1039862189317)) ;
#112539=CARTESIAN_POINT('Ctrl Pts',(66.7083031964201,247.607633986837,21.1060755646381)) ;
#112540=CARTESIAN_POINT('Ctrl Pts',(66.7054954325608,247.540422271368,21.121257895442)) ;
#112541=CARTESIAN_POINT('Ctrl Pts',(66.7026876687015,247.473891429089,21.1400093724741)) ;
#112542=CARTESIAN_POINT('Ctrl Pts',(66.6998799048422,247.408445683413,21.1622516345052)) ;
#112543=CARTESIAN_POINT('Ctrl Pts',(66.6970091821112,247.341532438862,21.1849926378093)) ;
#112544=CARTESIAN_POINT('Ctrl Pts',(66.6941384593802,247.275754062132,21.2113828453259)) ;
#112545=CARTESIAN_POINT('Ctrl Pts',(66.6912677366492,247.211530999387,21.2412832575483)) ;
#112546=CARTESIAN_POINT('Ctrl Pts',(66.688466935483,247.148872203716,21.2704553919782)) ;
#112547=CARTESIAN_POINT('Ctrl Pts',(66.6856661343169,247.08769428332,21.3029684559092)) ;
#112548=CARTESIAN_POINT('Ctrl Pts',(66.6828653331508,247.028369760528,21.3386438873749)) ;
#112549=CARTESIAN_POINT('Ctrl Pts',(66.6800660661747,246.969077733829,21.3742997769703)) ;
#112550=CARTESIAN_POINT('Ctrl Pts',(66.6772667991987,246.911637505547,21.4131143461349)) ;
#112551=CARTESIAN_POINT('Ctrl Pts',(66.6744675322227,246.856396541157,21.4548633645944)) ;
#112552=CARTESIAN_POINT('Ctrl Pts',(66.6716688672921,246.801167457582,21.4966034039868)) ;
#112553=CARTESIAN_POINT('Ctrl Pts',(66.6688702023615,246.748137085706,21.541276345894)) ;
#112554=CARTESIAN_POINT('Ctrl Pts',(66.6660715374309,246.697622033173,21.5886159692403)) ;
#112555=CARTESIAN_POINT('Ctrl Pts',(66.6631474559198,246.64484324943,21.638077023279)) ;
#112556=CARTESIAN_POINT('Ctrl Pts',(66.6602233744087,246.5948109811,21.6904490326929)) ;
#112557=CARTESIAN_POINT('Ctrl Pts',(66.6572992928976,246.54784403798,21.7453847650921)) ;
#112558=CARTESIAN_POINT('Ctrl Pts',(66.6544973328726,246.502838624615,21.7980261588232)) ;
#112559=CARTESIAN_POINT('Ctrl Pts',(66.6516953728476,246.460647846571,21.8530209500657)) ;
#112560=CARTESIAN_POINT('Ctrl Pts',(66.6488934128226,246.421509977807,21.9100309666791)) ;
#112561=CARTESIAN_POINT('Ctrl Pts',(66.6460896353153,246.382346722391,21.9670779626554)) ;
#112562=CARTESIAN_POINT('Ctrl Pts',(66.643285857808,246.346240570875,22.0261423714026)) ;
#112563=CARTESIAN_POINT('Ctrl Pts',(66.6404820803007,246.313384870534,22.0868595920092)) ;
#112564=CARTESIAN_POINT('Ctrl Pts',(66.6376740088167,246.280478851789,22.1476698008527)) ;
#112565=CARTESIAN_POINT('Ctrl Pts',(66.6348659373327,246.250833420726,22.2101374322724)) ;
#112566=CARTESIAN_POINT('Ctrl Pts',(66.6320578658488,246.224594237369,22.2738770077013)) ;
#112567=CARTESIAN_POINT('Ctrl Pts',(66.6316994303318,246.221244943982,22.2820130283832)) ;
#112568=CARTESIAN_POINT('Ctrl Pts',(66.6313409948149,246.217951082534,22.2901697529364)) ;
#112569=CARTESIAN_POINT('Ctrl Pts',(66.6309825592979,246.214712897158,22.2983463632043)) ;
#112570=CARTESIAN_POINT('Ctrl Pts',(66.6281800443638,246.189394360223,22.3622771716815)) ;
#112571=CARTESIAN_POINT('Ctrl Pts',(66.6253775294297,246.167391336414,22.4276576817178)) ;
#112572=CARTESIAN_POINT('Ctrl Pts',(66.6225750144956,246.148867895085,22.4941118138594)) ;
#112573=CARTESIAN_POINT('Ctrl Pts',(66.619703635649,246.129889292348,22.5621988691624)) ;
#112574=CARTESIAN_POINT('Ctrl Pts',(66.6168322568023,246.114563812163,22.6314125618807)) ;
#112575=CARTESIAN_POINT('Ctrl Pts',(66.6139608779556,246.103015479204,22.7013263958668)) ;
#112576=CARTESIAN_POINT('Ctrl Pts',(66.6111655312091,246.091772938011,22.7693889605107)) ;
#112577=CARTESIAN_POINT('Ctrl Pts',(66.6083701844626,246.084110072188,22.8381145319354)) ;
#112578=CARTESIAN_POINT('Ctrl Pts',(66.6055748377161,246.080090340551,22.9070963010212)) ;
#112579=CARTESIAN_POINT('Ctrl Pts',(66.6027810857162,246.076072902172,22.9760387159777)) ;
#112580=CARTESIAN_POINT('Ctrl Pts',(66.5999873337162,246.075694501959,23.0452365521402)) ;
#112581=CARTESIAN_POINT('Ctrl Pts',(66.5971935817163,246.078966771708,23.1142777902697)) ;
#112582=CARTESIAN_POINT('Ctrl Pts',(66.5944004829009,246.082238276395,23.1833028864261)) ;
#112583=CARTESIAN_POINT('Ctrl Pts',(66.5916073840854,246.089158732519,23.2521709698612)) ;
#112584=CARTESIAN_POINT('Ctrl Pts',(66.58881428527,246.099687690267,23.320471704272)) ;
#112585=CARTESIAN_POINT('Ctrl Pts',(66.5858849216788,246.110730316225,23.3921045743768)) ;
#112586=CARTESIAN_POINT('Ctrl Pts',(66.5829555580876,246.12574249303,23.4631127389016)) ;
#112587=CARTESIAN_POINT('Ctrl Pts',(66.5800261944964,246.144616879569,23.5330331974709)) ;
#112588=CARTESIAN_POINT('Ctrl Pts',(66.5772298638925,246.162634112004,23.5997783153261)) ;
#112589=CARTESIAN_POINT('Ctrl Pts',(66.5744335332887,246.184170152109,23.6655319101723)) ;
#112590=CARTESIAN_POINT('Ctrl Pts',(66.5716372026848,246.20908072843,23.729907683838)) ;
#112591=CARTESIAN_POINT('Ctrl Pts',(66.5688390712557,246.234007347058,23.7943249152326)) ;
#112592=CARTESIAN_POINT('Ctrl Pts',(66.5660409398266,246.262312626854,23.8573621146967)) ;
#112593=CARTESIAN_POINT('Ctrl Pts',(66.5632428083975,246.293805132647,23.9186551780761)) ;
#112594=CARTESIAN_POINT('Ctrl Pts',(66.5604403673259,246.325346142753,23.9800426441668)) ;
#112595=CARTESIAN_POINT('Ctrl Pts',(66.5576379262542,246.360083924017,24.0396801960135)) ;
#112596=CARTESIAN_POINT('Ctrl Pts',(66.5548354851826,246.39778291499,24.0972313511934)) ;
#112597=CARTESIAN_POINT('Ctrl Pts',(66.5544442975136,246.4030452488,24.1052648126169)) ;
#112598=CARTESIAN_POINT('Ctrl Pts',(66.5540531098447,246.408365216766,24.1132576730071)) ;
#112599=CARTESIAN_POINT('Ctrl Pts',(66.5536619221757,246.413742116473,24.1212090691728)) ;
#112600=CARTESIAN_POINT('Ctrl Pts',(66.5508575245513,246.452288742457,24.1782120840603)) ;
#112601=CARTESIAN_POINT('Ctrl Pts',(66.5480531269269,246.493905844935,24.2332903096945)) ;
#112602=CARTESIAN_POINT('Ctrl Pts',(66.5452487293026,246.538374695132,24.2860959910081)) ;
#112603=CARTESIAN_POINT('Ctrl Pts',(66.5423775857922,246.583901923349,24.3401584705568)) ;
#112604=CARTESIAN_POINT('Ctrl Pts',(66.5395064422818,246.63241817426,24.3918383655865)) ;
#112605=CARTESIAN_POINT('Ctrl Pts',(66.5366352987714,246.683641153788,24.4407933786813)) ;
#112606=CARTESIAN_POINT('Ctrl Pts',(66.5338380154614,246.733546421569,24.4884890234926)) ;
#112607=CARTESIAN_POINT('Ctrl Pts',(66.5310407321513,246.786020452675,24.5335979395467)) ;
#112608=CARTESIAN_POINT('Ctrl Pts',(66.5282434488413,246.840762508303,24.5758381993054)) ;
#112609=CARTESIAN_POINT('Ctrl Pts',(66.5254477458841,246.895473636864,24.6180545950115)) ;
#112610=CARTESIAN_POINT('Ctrl Pts',(66.5226520429269,246.952449861992,24.6574052534587)) ;
#112611=CARTESIAN_POINT('Ctrl Pts',(66.5198563399697,247.011356947953,24.693648136975)) ;
#112612=CARTESIAN_POINT('Ctrl Pts',(66.5170612791496,247.070250503714,24.7298826959663)) ;
#112613=CARTESIAN_POINT('Ctrl Pts',(66.5142662183296,247.131073624387,24.7630106427246)) ;
#112614=CARTESIAN_POINT('Ctrl Pts',(66.5114711575094,247.193464120806,24.7928339163131)) ;
#112615=CARTESIAN_POINT('Ctrl Pts',(66.5085436681381,247.258810647016,24.8240702013415)) ;
#112616=CARTESIAN_POINT('Ctrl Pts',(66.5056161787668,247.325876260209,24.85168059151)) ;
#112617=CARTESIAN_POINT('Ctrl Pts',(66.5026886893955,247.394219302264,24.875493223085)) ;
#112618=CARTESIAN_POINT('Ctrl Pts',(66.4998903921052,247.459546319764,24.8982549871627)) ;
#112619=CARTESIAN_POINT('Ctrl Pts',(66.497092094815,247.526039885201,24.9175470467986)) ;
#112620=CARTESIAN_POINT('Ctrl Pts',(66.4942937975247,247.593299161412,24.9332705763801)) ;
#112621=CARTESIAN_POINT('Ctrl Pts',(66.4914936996295,247.66060171658,24.9490042234946)) ;
#112622=CARTESIAN_POINT('Ctrl Pts',(66.4886936017343,247.728670483708,24.961164685035)) ;
#112623=CARTESIAN_POINT('Ctrl Pts',(66.4858935038391,247.797096347173,24.9697045982337)) ;
#112624=CARTESIAN_POINT('Ctrl Pts',(66.4830891103635,247.865627181538,24.9782576123614)) ;
#112625=CARTESIAN_POINT('Ctrl Pts',(66.4802847168879,247.934515719959,24.9831789660512)) ;
#112626=CARTESIAN_POINT('Ctrl Pts',(66.4774803234124,248.00335075709,24.9844733128192)) ;
#112627=CARTESIAN_POINT('Ctrl Pts',(66.4771006439594,248.012670151629,24.984648551022)) ;
#112628=CARTESIAN_POINT('Ctrl Pts',(66.4767209645065,248.021988571689,24.9847573850635)) ;
#112629=CARTESIAN_POINT('Ctrl Pts',(66.4763412850535,248.031305004152,24.9847998994865)) ;
#112630=CARTESIAN_POINT('Ctrl Pts',(66.4735367028759,248.100122793056,24.9851139412185)) ;
#112631=CARTESIAN_POINT('Ctrl Pts',(66.4707321206983,248.169082326696,24.981806256511)) ;
#112632=CARTESIAN_POINT('Ctrl Pts',(66.4679275385207,248.237773013919,24.9748614557492)) ;
#112633=CARTESIAN_POINT('Ctrl Pts',(66.4650564180795,248.30809337671,24.9677518907)) ;
#112634=CARTESIAN_POINT('Ctrl Pts',(66.4621852976383,248.378131459492,24.9568303286319)) ;
#112635=CARTESIAN_POINT('Ctrl Pts',(66.4593141771971,248.447445444109,24.9421369469113)) ;
#112636=CARTESIAN_POINT('Ctrl Pts',(66.4565166884835,248.514981827075,24.9278203864017)) ;
#112637=CARTESIAN_POINT('Ctrl Pts',(66.45371919977,248.581830299186,24.9099232607873)) ;
#112638=CARTESIAN_POINT('Ctrl Pts',(66.4509217110564,248.647588407351,24.8885350231841)) ;
#112639=CARTESIAN_POINT('Ctrl Pts',(66.4481257955151,248.713309536339,24.8671588132905)) ;
#112640=CARTESIAN_POINT('Ctrl Pts',(66.4453298799738,248.77794105567,24.8422955378968)) ;
#112641=CARTESIAN_POINT('Ctrl Pts',(66.4425339644325,248.841094575183,24.8140848049847)) ;
#112642=CARTESIAN_POINT('Ctrl Pts',(66.4397386841844,248.904233744834,24.7858804821683)) ;
#112643=CARTESIAN_POINT('Ctrl Pts',(66.4369434039363,248.965895137064,24.7543304114707)) ;
#112644=CARTESIAN_POINT('Ctrl Pts',(66.4341481236882,249.025710924317,24.7196220813791)) ;
#112645=CARTESIAN_POINT('Ctrl Pts',(66.4312208340418,249.088351561096,24.6832746219824)) ;
#112646=CARTESIAN_POINT('Ctrl Pts',(66.4282935443954,249.148967429664,24.6434634608389)) ;
#112647=CARTESIAN_POINT('Ctrl Pts',(66.425366254749,249.20716770085,24.6004563694609)) ;
#112648=CARTESIAN_POINT('Ctrl Pts',(66.4225677232717,249.262808006586,24.5593409645963)) ;
#112649=CARTESIAN_POINT('Ctrl Pts',(66.4197691917944,249.316240403472,24.5153052507546)) ;
#112650=CARTESIAN_POINT('Ctrl Pts',(66.4169706603171,249.367157228193,24.4686245793031)) ;
#112651=CARTESIAN_POINT('Ctrl Pts',(66.4141703233186,249.418106902789,24.4219137910052)) ;
#112652=CARTESIAN_POINT('Ctrl Pts',(66.4113699863201,249.466537434248,24.3725549965347)) ;
#112653=CARTESIAN_POINT('Ctrl Pts',(66.4085696493216,249.51217899423,24.3208594006466)) ;
#112654=CARTESIAN_POINT('Ctrl Pts',(66.4057650114089,249.557890653073,24.26908440777)) ;
#112655=CARTESIAN_POINT('Ctrl Pts',(66.4029603734962,249.600804495448,24.214965836329)) ;
#112656=CARTESIAN_POINT('Ctrl Pts',(66.4001557355835,249.640692473552,24.1588459463071)) ;
#112657=CARTESIAN_POINT('Ctrl Pts',(66.3997773730328,249.6460736021,24.1512750350546)) ;
#112658=CARTESIAN_POINT('Ctrl Pts',(66.3993990104821,249.651399728399,24.1436677390925)) ;
#112659=CARTESIAN_POINT('Ctrl Pts',(66.3990206479314,249.656670356245,24.1360249334639)) ;
#112660=CARTESIAN_POINT('Ctrl Pts',(66.3961923042638,249.696069463972,24.0788932726709)) ;
#112661=CARTESIAN_POINT('Ctrl Pts',(66.3933639605962,249.73250654892,24.0195681046214)) ;
#112662=CARTESIAN_POINT('Ctrl Pts',(66.3905356169286,249.765733822899,23.9583848894514)) ;
#112663=CARTESIAN_POINT('Ctrl Pts',(66.3877114631021,249.798911874783,23.897292309643)) ;
#112664=CARTESIAN_POINT('Ctrl Pts',(66.3848873092756,249.828889330847,23.8343475626674)) ;
#112665=CARTESIAN_POINT('Ctrl Pts',(66.3820631554491,249.855461540977,23.7699151331032)) ;
#112666=CARTESIAN_POINT('Ctrl Pts',(66.3792426862401,249.881999082872,23.7055667672503)) ;
#112667=CARTESIAN_POINT('Ctrl Pts',(66.376422217031,249.905140028878,23.6397350147491)) ;
#112668=CARTESIAN_POINT('Ctrl Pts',(66.3736017478219,249.924726369716,23.5728074261705)) ;
#112669=CARTESIAN_POINT('Ctrl Pts',(66.3707834643677,249.944297531895,23.505931703891)) ;
#112670=CARTESIAN_POINT('Ctrl Pts',(66.3679651809134,249.960319426279,23.437962287707)) ;
#112671=CARTESIAN_POINT('Ctrl Pts',(66.3651468974592,249.972683213614,23.3693038406779)) ;
#112672=CARTESIAN_POINT('Ctrl Pts',(66.3623295387996,249.985042943883,23.3006679233083)) ;
#112673=CARTESIAN_POINT('Ctrl Pts',(66.35951218014,249.993746861307,23.2313438912878)) ;
#112674=CARTESIAN_POINT('Ctrl Pts',(66.3566948214805,249.998737100951,23.1617471999234)) ;
#112675=CARTESIAN_POINT('Ctrl Pts',(66.3547891772058,250.002112468718,23.1146724208622)) ;
#112676=CARTESIAN_POINT('Ctrl Pts',(66.3528835329311,250.003789857887,23.067473125536)) ;
#112677=CARTESIAN_POINT('Ctrl Pts',(66.3509778886564,250.003764831718,23.0202791331489)) ;
#112678=CARTESIAN_POINT('',(65.8509778886254,250.003764915913,23.0221883796948)) ;
#112679=CARTESIAN_POINT('Ctrl Pts',(66.3509778886297,250.003764831718,23.0202791324881)) ;
#112680=CARTESIAN_POINT('Ctrl Pts',(66.3478598655463,250.00372388377,22.9430601259727)) ;
#112681=CARTESIAN_POINT('Ctrl Pts',(66.3447418424628,249.999123582142,22.8659967115464)) ;
#112682=CARTESIAN_POINT('Ctrl Pts',(66.3416238193793,249.99004343271,22.7895947867999)) ;
#112683=CARTESIAN_POINT('Ctrl Pts',(66.3384932790686,249.980926831241,22.7128861483981)) ;
#112684=CARTESIAN_POINT('Ctrl Pts',(66.3353627387578,249.967294471348,22.6368445763685)) ;
#112685=CARTESIAN_POINT('Ctrl Pts',(66.332232198447,249.949276702868,22.5619653829443)) ;
#112686=CARTESIAN_POINT('Ctrl Pts',(66.3290871137584,249.931175224483,22.4867383034769)) ;
#112687=CARTESIAN_POINT('Ctrl Pts',(66.3259420290698,249.908647624235,22.4126846747573)) ;
#112688=CARTESIAN_POINT('Ctrl Pts',(66.3227969443812,249.881874367055,22.3402861401784)) ;
#112689=CARTESIAN_POINT('Ctrl Pts',(66.3224312998572,249.8787617339,22.3318691561106)) ;
#112690=CARTESIAN_POINT('Ctrl Pts',(66.3220656553331,249.875591767863,22.3234745173636)) ;
#112691=CARTESIAN_POINT('Ctrl Pts',(66.3217000108091,249.872364793347,22.3151029604768)) ;
#112692=CARTESIAN_POINT('Ctrl Pts',(66.3188956978973,249.847615492569,22.2508972537666)) ;
#112693=CARTESIAN_POINT('Ctrl Pts',(66.3160913849855,249.819441896056,22.1878769828483)) ;
#112694=CARTESIAN_POINT('Ctrl Pts',(66.3132870720737,249.787978979235,22.1264301416105)) ;
#112695=CARTESIAN_POINT('Ctrl Pts',(66.3104159179742,249.755766139423,22.0635187063797)) ;
#112696=CARTESIAN_POINT('Ctrl Pts',(66.3075447638748,249.720105261573,22.0022571831292)) ;
#112697=CARTESIAN_POINT('Ctrl Pts',(66.3046736097753,249.681194506994,21.9430425700643)) ;
#112698=CARTESIAN_POINT('Ctrl Pts',(66.3018764061595,249.643285951886,21.885353109994)) ;
#112699=CARTESIAN_POINT('Ctrl Pts',(66.2990792025437,249.602293203379,21.8296068199877)) ;
#112700=CARTESIAN_POINT('Ctrl Pts',(66.2962819989278,249.558445944019,21.7761459788644)) ;
#112701=CARTESIAN_POINT('Ctrl Pts',(66.2934863735306,249.514623423853,21.7227153010431)) ;
#112702=CARTESIAN_POINT('Ctrl Pts',(66.2906907481334,249.467949897479,21.6715678893151)) ;
#112703=CARTESIAN_POINT('Ctrl Pts',(66.2878951227363,249.418696651158,21.6230146794661)) ;
#112704=CARTESIAN_POINT('Ctrl Pts',(66.2851001371771,249.369454677485,21.574472582046)) ;
#112705=CARTESIAN_POINT('Ctrl Pts',(66.2823051516179,249.317634503699,21.528523849089)) ;
#112706=CARTESIAN_POINT('Ctrl Pts',(66.2795101660587,249.263544535983,21.4854428450103)) ;
#112707=CARTESIAN_POINT('Ctrl Pts',(66.2765826000278,249.206888804227,21.4403182883889)) ;
#112708=CARTESIAN_POINT('Ctrl Pts',(66.2736550339968,249.147743009541,21.3983406892389)) ;
#112709=CARTESIAN_POINT('Ctrl Pts',(66.2707274679658,249.086498940256,21.3597767787396)) ;
#112710=CARTESIAN_POINT('Ctrl Pts',(66.2679292391154,249.027960577747,21.322916586415)) ;
#112711=CARTESIAN_POINT('Ctrl Pts',(66.265131010265,248.967505907819,21.2891750088955)) ;
#112712=CARTESIAN_POINT('Ctrl Pts',(66.2623327814145,248.905503294256,21.2587383935005)) ;
#112713=CARTESIAN_POINT('Ctrl Pts',(66.259532749504,248.843460728835,21.2282821660402)) ;
#112714=CARTESIAN_POINT('Ctrl Pts',(66.2567327175935,248.779868682643,21.2011353301055)) ;
#112715=CARTESIAN_POINT('Ctrl Pts',(66.2539326856829,248.715115147543,21.1774359453826)) ;
#112716=CARTESIAN_POINT('Ctrl Pts',(66.251128354205,248.65026218065,21.1537001692522)) ;
#112717=CARTESIAN_POINT('Ctrl Pts',(66.248324022727,248.584244632475,21.1334225449265)) ;
#112718=CARTESIAN_POINT('Ctrl Pts',(66.2455196912491,248.517464216764,21.116690914933)) ;
#112719=CARTESIAN_POINT('Ctrl Pts',(66.2451395853951,248.50841263811,21.1144230694384)) ;
#112720=CARTESIAN_POINT('Ctrl Pts',(66.2447594795411,248.49934705575,21.1122202925466)) ;
#112721=CARTESIAN_POINT('Ctrl Pts',(66.2443793736871,248.490268479293,21.1100827299615)) ;
#112722=CARTESIAN_POINT('Ctrl Pts',(66.2415750693281,248.42328952787,21.0943124490994)) ;
#112723=CARTESIAN_POINT('Ctrl Pts',(66.2387707649692,248.355358414636,21.0820385006588)) ;
#112724=CARTESIAN_POINT('Ctrl Pts',(66.2359664606102,248.286871667356,21.0733682253655)) ;
#112725=CARTESIAN_POINT('Ctrl Pts',(66.2330953054417,248.216752288978,21.0644912624774)) ;
#112726=CARTESIAN_POINT('Ctrl Pts',(66.2302241502731,248.146050924723,21.0593922007215)) ;
#112727=CARTESIAN_POINT('Ctrl Pts',(66.2273529951046,248.075207175511,21.0581312793319)) ;
#112728=CARTESIAN_POINT('Ctrl Pts',(66.2245557989252,248.00618831272,21.0569028384131)) ;
#112729=CARTESIAN_POINT('Ctrl Pts',(66.2217586027458,247.937034832054,21.0593171883096)) ;
#112730=CARTESIAN_POINT('Ctrl Pts',(66.2189614065664,247.868158918274,21.0653776783642)) ;
#112731=CARTESIAN_POINT('Ctrl Pts',(66.2161657881682,247.799321854513,21.0714347499501)) ;
#112732=CARTESIAN_POINT('Ctrl Pts',(66.2133701697701,247.730762531577,21.0811338376834)) ;
#112733=CARTESIAN_POINT('Ctrl Pts',(66.210574551372,247.662890712547,21.0944262582976)) ;
#112734=CARTESIAN_POINT('Ctrl Pts',(66.2077795723613,247.595034416518,21.1077156387949)) ;
#112735=CARTESIAN_POINT('Ctrl Pts',(66.2049845933506,247.527865790172,21.1245966259734)) ;
#112736=CARTESIAN_POINT('Ctrl Pts',(66.2021896143399,247.461785328639,21.1449692583098)) ;
#112737=CARTESIAN_POINT('Ctrl Pts',(66.199262041192,247.392570002138,21.1663083707512)) ;
#112738=CARTESIAN_POINT('Ctrl Pts',(66.1963344680441,247.32454922249,21.1914785334405)) ;
#112739=CARTESIAN_POINT('Ctrl Pts',(66.1934068948962,247.258164209242,21.2203066194318)) ;
#112740=CARTESIAN_POINT('Ctrl Pts',(66.190608671379,247.194712300146,21.2478609875378)) ;
#112741=CARTESIAN_POINT('Ctrl Pts',(66.1878104478619,247.132755087318,21.2787565729174)) ;
#112742=CARTESIAN_POINT('Ctrl Pts',(66.1850122243447,247.072654192038,21.312794263652)) ;
#112743=CARTESIAN_POINT('Ctrl Pts',(66.1822121973405,247.012514561043,21.3468538920675)) ;
#112744=CARTESIAN_POINT('Ctrl Pts',(66.1794121703363,246.954234039149,21.3840593940906)) ;
#112745=CARTESIAN_POINT('Ctrl Pts',(66.1766121433321,246.898145439722,21.4241682174863)) ;
#112746=CARTESIAN_POINT('Ctrl Pts',(66.1738078161204,246.841970700905,21.4643386389532)) ;
#112747=CARTESIAN_POINT('Ctrl Pts',(66.1710034889088,246.787994978288,21.507420971324)) ;
#112748=CARTESIAN_POINT('Ctrl Pts',(66.1681991616971,246.736517353207,21.5531330113605)) ;
#112749=CARTESIAN_POINT('Ctrl Pts',(66.1678190199863,246.729539282894,21.559329525458)) ;
#112750=CARTESIAN_POINT('Ctrl Pts',(66.1674388782756,246.722607058264,21.5655743079229)) ;
#112751=CARTESIAN_POINT('Ctrl Pts',(66.1670587365648,246.715721369191,21.5718666069575)) ;
#112752=CARTESIAN_POINT('Ctrl Pts',(66.164254472231,246.664926384755,21.6182842171846)) ;
#112753=CARTESIAN_POINT('Ctrl Pts',(66.1614502078971,246.616481631369,21.6674598175612)) ;
#112754=CARTESIAN_POINT('Ctrl Pts',(66.1586459435633,246.570699372434,21.719126502582)) ;
#112755=CARTESIAN_POINT('Ctrl Pts',(66.1557747833916,246.523824975881,21.7720256984405)) ;
#112756=CARTESIAN_POINT('Ctrl Pts',(66.1529036232199,246.479742176359,21.8275360775242)) ;
#112757=CARTESIAN_POINT('Ctrl Pts',(66.1500324630482,246.438748647046,21.8853285847958)) ;
#112758=CARTESIAN_POINT('Ctrl Pts',(66.1472353088917,246.398811752532,21.9416314527184)) ;
#112759=CARTESIAN_POINT('Ctrl Pts',(66.1444381547351,246.361807088797,22.0000997932479)) ;
#112760=CARTESIAN_POINT('Ctrl Pts',(66.1416410005786,246.32796987339,22.0603951226066)) ;
#112761=CARTESIAN_POINT('Ctrl Pts',(66.1388454248234,246.294151751928,22.1206564280162)) ;
#112762=CARTESIAN_POINT('Ctrl Pts',(66.1360498490683,246.26349776992,22.1827422520709)) ;
#112763=CARTESIAN_POINT('Ctrl Pts',(66.1332542733131,246.236198810827,22.2462867661089)) ;
#112764=CARTESIAN_POINT('Ctrl Pts',(66.1304593374925,246.208906100731,22.3098167341885)) ;
#112765=CARTESIAN_POINT('Ctrl Pts',(66.1276644016719,246.184967080257,22.3748042812797)) ;
#112766=CARTESIAN_POINT('Ctrl Pts',(66.1248694658512,246.16452506053,22.4408623131028)) ;
#112767=CARTESIAN_POINT('Ctrl Pts',(66.1219418519838,246.143112640257,22.5100561774446)) ;
#112768=CARTESIAN_POINT('Ctrl Pts',(66.1190142381165,246.125537714434,22.5804241505789)) ;
#112769=CARTESIAN_POINT('Ctrl Pts',(66.1160866242491,246.111906148906,22.6515042058526)) ;
#112770=CARTESIAN_POINT('Ctrl Pts',(66.1132884447899,246.098877256305,22.7194417002207)) ;
#112771=CARTESIAN_POINT('Ctrl Pts',(66.1104902653307,246.089450404183,22.7880291263575)) ;
#112772=CARTESIAN_POINT('Ctrl Pts',(66.1076920858715,246.083665100118,22.8568555753116)) ;
#112773=CARTESIAN_POINT('Ctrl Pts',(66.1048921031845,246.077876067837,22.9257263780205)) ;
#112774=CARTESIAN_POINT('Ctrl Pts',(66.1020921204975,246.075733269037,22.9948360232998)) ;
#112775=CARTESIAN_POINT('Ctrl Pts',(66.0992921378105,246.077224091665,23.0637728938718)) ;
#112776=CARTESIAN_POINT('Ctrl Pts',(66.0964878549738,246.078717203865,23.1328156361199)) ;
#112777=CARTESIAN_POINT('Ctrl Pts',(66.0936835721371,246.083855031025,23.2016845896588)) ;
#112778=CARTESIAN_POINT('Ctrl Pts',(66.0908792893005,246.092573193766,23.2699736324214)) ;
#112779=CARTESIAN_POINT('Ctrl Pts',(66.0904988926812,246.093755799026,23.279236935202)) ;
#112780=CARTESIAN_POINT('Ctrl Pts',(66.090118496062,246.095004207766,23.2884895848537)) ;
#112781=CARTESIAN_POINT('Ctrl Pts',(66.0897380994427,246.096318187715,23.297730585677)) ;
#112782=CARTESIAN_POINT('Ctrl Pts',(66.0869338127968,246.106004857464,23.3658553110087)) ;
#112783=CARTESIAN_POINT('Ctrl Pts',(66.084129526151,246.119294572346,23.4335945163826)) ;
#112784=CARTESIAN_POINT('Ctrl Pts',(66.0813252395051,246.136143011513,23.5005398052726)) ;
#112785=CARTESIAN_POINT('Ctrl Pts',(66.0784540821224,246.153393216863,23.5690814647762)) ;
#112786=CARTESIAN_POINT('Ctrl Pts',(66.0755829247397,246.174374068109,23.6367903357114)) ;
#112787=CARTESIAN_POINT('Ctrl Pts',(66.072711767357,246.198981695181,23.7032350335809)) ;
#112788=CARTESIAN_POINT('Ctrl Pts',(66.0699145900767,246.222955266182,23.7679676742907)) ;
#112789=CARTESIAN_POINT('Ctrl Pts',(66.0671174127965,246.25037078009,23.8315000180623)) ;
#112790=CARTESIAN_POINT('Ctrl Pts',(66.0643202355162,246.281081356968,23.8934469288994)) ;
#112791=CARTESIAN_POINT('Ctrl Pts',(66.0615246364033,246.311774606937,23.9553588892896)) ;
#112792=CARTESIAN_POINT('Ctrl Pts',(66.0587290372905,246.345759014471,24.0156867559789)) ;
#112793=CARTESIAN_POINT('Ctrl Pts',(66.0559334381776,246.382840116105,24.0740665840905)) ;
#112794=CARTESIAN_POINT('Ctrl Pts',(66.0531384788057,246.419912732153,24.132433052645)) ;
#112795=CARTESIAN_POINT('Ctrl Pts',(66.0503435194338,246.460080373364,24.1888519568964)) ;
#112796=CARTESIAN_POINT('Ctrl Pts',(66.0475485600618,246.503104186896,24.242986645497)) ;
#112797=CARTESIAN_POINT('Ctrl Pts',(66.0446209685834,246.548169654084,24.2996902436343)) ;
#112798=CARTESIAN_POINT('Ctrl Pts',(66.0416933771049,246.596368790051,24.3538869569526)) ;
#112799=CARTESIAN_POINT('Ctrl Pts',(66.0387657856265,246.64737976016,24.4052288153768)) ;
#112800=CARTESIAN_POINT('Ctrl Pts',(66.0359675824079,246.696136241994,24.4543015615391)) ;
#112801=CARTESIAN_POINT('Ctrl Pts',(66.0331693791894,246.747460835214,24.5007661813184)) ;
#112802=CARTESIAN_POINT('Ctrl Pts',(66.0303711759709,246.801036481884,24.5443583150971)) ;
#112803=CARTESIAN_POINT('Ctrl Pts',(66.0275711694751,246.854646654904,24.5879785414393)) ;
#112804=CARTESIAN_POINT('Ctrl Pts',(66.0247711629794,246.910510374953,24.6287223107252)) ;
#112805=CARTESIAN_POINT('Ctrl Pts',(66.0219711564836,246.968280606469,24.6663679048587)) ;
#112806=CARTESIAN_POINT('Ctrl Pts',(66.0191668499349,247.026139557442,24.7040713124466)) ;
#112807=CARTESIAN_POINT('Ctrl Pts',(66.0163625433862,247.085910438564,24.7386668120072)) ;
#112808=CARTESIAN_POINT('Ctrl Pts',(66.0135582368375,247.14722155821,24.7699785344481)) ;
#112809=CARTESIAN_POINT('Ctrl Pts',(66.0131779786652,247.155535219323,24.7742243392991)) ;
#112810=CARTESIAN_POINT('Ctrl Pts',(66.0127977204928,247.163877171844,24.7784098389931)) ;
#112811=CARTESIAN_POINT('Ctrl Pts',(66.0124174623205,247.172246463579,24.7825346642229)) ;
#112812=CARTESIAN_POINT('Ctrl Pts',(66.0096131786355,247.233967341589,24.8129539449549)) ;
#112813=CARTESIAN_POINT('Ctrl Pts',(66.0068088949506,247.297401774136,24.8401803846579)) ;
#112814=CARTESIAN_POINT('Ctrl Pts',(66.0040046112657,247.362187508978,24.8640202702962)) ;
#112815=CARTESIAN_POINT('Ctrl Pts',(66.0011334535129,247.428518196513,24.8884286683639)) ;
#112816=CARTESIAN_POINT('Ctrl Pts',(65.9982622957601,247.496265043163,24.9092866076992)) ;
#112817=CARTESIAN_POINT('Ctrl Pts',(65.9953911380073,247.565013228913,24.9264365871594)) ;
#112818=CARTESIAN_POINT('Ctrl Pts',(65.9925939636882,247.631989924803,24.9431446492891)) ;
#112819=CARTESIAN_POINT('Ctrl Pts',(65.9897967893692,247.699916471284,24.9563334198154)) ;
#112820=CARTESIAN_POINT('Ctrl Pts',(65.9869996150501,247.768391987,24.9659069978885)) ;
#112821=CARTESIAN_POINT('Ctrl Pts',(65.9842040188898,247.836828869002,24.975475174573)) ;
#112822=CARTESIAN_POINT('Ctrl Pts',(65.9814084227294,247.905813623758,24.9814321391612)) ;
#112823=CARTESIAN_POINT('Ctrl Pts',(65.978612826569,247.974936035212,24.983733236474)) ;
#112824=CARTESIAN_POINT('Ctrl Pts',(65.9758178701356,248.044042629119,24.9860338072178)) ;
#112825=CARTESIAN_POINT('Ctrl Pts',(65.9730229137023,248.113286330197,24.98468015634)) ;
#112826=CARTESIAN_POINT('Ctrl Pts',(65.9702279572689,248.182254428473,24.9796796780054)) ;
#112827=CARTESIAN_POINT('Ctrl Pts',(65.9673003629297,248.254495488007,24.9744418961598)) ;
#112828=CARTESIAN_POINT('Ctrl Pts',(65.9643727685905,248.326433553938,24.9652025381067)) ;
#112829=CARTESIAN_POINT('Ctrl Pts',(65.9614451742512,248.397599769185,24.95203114266)) ;
#112830=CARTESIAN_POINT('Ctrl Pts',(65.9586469739006,248.46562057582,24.9394418973321)) ;
#112831=CARTESIAN_POINT('Ctrl Pts',(65.95584877355,248.532935839477,24.9232610403545)) ;
#112832=CARTESIAN_POINT('Ctrl Pts',(65.9530505731994,248.599148446129,24.9036013173046)) ;
#112833=CARTESIAN_POINT('Ctrl Pts',(65.9502505695442,248.665403723597,24.8839289245158)) ;
#112834=CARTESIAN_POINT('Ctrl Pts',(65.9474505658891,248.730554470939,24.8607733669065)) ;
#112835=CARTESIAN_POINT('Ctrl Pts',(65.9446505622339,248.794221882277,24.8342961934261)) ;
#112836=CARTESIAN_POINT('Ctrl Pts',(65.941846258467,248.857987070981,24.8077783575687)) ;
#112837=CARTESIAN_POINT('Ctrl Pts',(65.9390419547001,248.920263941948,24.7779289420863)) ;
#112838=CARTESIAN_POINT('Ctrl Pts',(65.9362376509332,248.980697647301,24.7449557135322)) ;
#112839=CARTESIAN_POINT('Ctrl Pts',(65.9358573756882,248.988892708899,24.7404844067096)) ;
#112840=CARTESIAN_POINT('Ctrl Pts',(65.9354771004433,248.997053921597,24.7359557225192)) ;
#112841=CARTESIAN_POINT('Ctrl Pts',(65.9350968251983,249.005180443317,24.7313702391054)) ;
#112842=CARTESIAN_POINT('Ctrl Pts',(65.9322925440763,249.065108223923,24.6975552991548)) ;
#112843=CARTESIAN_POINT('Ctrl Pts',(65.9294882629542,249.12336567858,24.6605247010165)) ;
#112844=CARTESIAN_POINT('Ctrl Pts',(65.9266839818322,249.179588546289,24.6204683518684)) ;
#112845=CARTESIAN_POINT('Ctrl Pts',(65.923812823759,249.237152226068,24.5794567324075)) ;
#112846=CARTESIAN_POINT('Ctrl Pts',(65.9209416656859,249.292582536227,24.535273362707)) ;
#112847=CARTESIAN_POINT('Ctrl Pts',(65.9180705076127,249.345515473325,24.4881719833853)) ;
#112848=CARTESIAN_POINT('Ctrl Pts',(65.9152733360198,249.397084388795,24.4422843530754)) ;
#112849=CARTESIAN_POINT('Ctrl Pts',(65.912476164427,249.44628270396,24.3936276378496)) ;
#112850=CARTESIAN_POINT('Ctrl Pts',(65.9096789928341,249.492805147331,24.3424788062426)) ;
#112851=CARTESIAN_POINT('Ctrl Pts',(65.9068833994527,249.539301341954,24.2913588336705)) ;
#112852=CARTESIAN_POINT('Ctrl Pts',(65.9040878060713,249.583124333545,24.237749895005)) ;
#112853=CARTESIAN_POINT('Ctrl Pts',(65.9012922126899,249.624005905544,24.1819655673543)) ;
#112854=CARTESIAN_POINT('Ctrl Pts',(65.8984972590836,249.664878121744,24.1261940060159)) ;
#112855=CARTESIAN_POINT('Ctrl Pts',(65.8957023054772,249.702809967544,24.0682484376347)) ;
#112856=CARTESIAN_POINT('Ctrl Pts',(65.8929073518708,249.737574802841,24.0084738519221)) ;
#112857=CARTESIAN_POINT('Ctrl Pts',(65.8899797548879,249.773989513516,23.9458624739065)) ;
#112858=CARTESIAN_POINT('Ctrl Pts',(65.887052157905,249.806928798476,23.8812446314136)) ;
#112859=CARTESIAN_POINT('Ctrl Pts',(65.8841245609221,249.836185672244,23.815046729765)) ;
#112860=CARTESIAN_POINT('Ctrl Pts',(65.8813263634862,249.864149394586,23.7517747699488)) ;
#112861=CARTESIAN_POINT('Ctrl Pts',(65.8785281660502,249.888749240932,23.6870599811523)) ;
#112862=CARTESIAN_POINT('Ctrl Pts',(65.8757299686142,249.90985436691,23.6212938864512)) ;
#112863=CARTESIAN_POINT('Ctrl Pts',(65.8729299679014,249.930973093924,23.5554854092946)) ;
#112864=CARTESIAN_POINT('Ctrl Pts',(65.8701299671885,249.948592494345,23.488624748837)) ;
#112865=CARTESIAN_POINT('Ctrl Pts',(65.8673299664757,249.962632350994,23.4211158315783)) ;
#112866=CARTESIAN_POINT('Ctrl Pts',(65.8645256656697,249.976693769313,23.3535032376927)) ;
#112867=CARTESIAN_POINT('Ctrl Pts',(65.8617213648638,249.987164606302,23.2852408819655)) ;
#112868=CARTESIAN_POINT('Ctrl Pts',(65.8589170640578,249.994016322833,23.2167389703612)) ;
#112869=CARTESIAN_POINT('Ctrl Pts',(65.8585367720639,249.994945485973,23.2074494075246)) ;
#112870=CARTESIAN_POINT('Ctrl Pts',(65.85815648007,249.995808171389,23.1981554393389)) ;
#112871=CARTESIAN_POINT('Ctrl Pts',(65.8577761880761,249.996604381633,23.1888580873809)) ;
#112872=CARTESIAN_POINT('Ctrl Pts',(65.8555100882696,250.001348872468,23.1334566384633)) ;
#112873=CARTESIAN_POINT('Ctrl Pts',(65.853243988463,250.003740308255,23.0778509121811)) ;
#112874=CARTESIAN_POINT('Ctrl Pts',(65.8509778886564,250.003764915912,23.0221883804556)) ;
#112875=CARTESIAN_POINT('',(65.3509778886241,250.003765042575,23.0208142978541)) ;
#112876=CARTESIAN_POINT('Ctrl Pts',(65.8509778886254,250.003764915913,23.0221883796948)) ;
#112877=CARTESIAN_POINT('Ctrl Pts',(65.8482056816273,250.00379501938,22.9540942650674)) ;
#112878=CARTESIAN_POINT('Ctrl Pts',(65.8454334746292,250.000278609981,22.8858688531145)) ;
#112879=CARTESIAN_POINT('Ctrl Pts',(65.842661267631,249.993201004529,22.8179152472297)) ;
#112880=CARTESIAN_POINT('Ctrl Pts',(65.839893088671,249.986133682892,22.7500603784575)) ;
#112881=CARTESIAN_POINT('Ctrl Pts',(65.837124909711,249.975515490756,22.6824770252418)) ;
#112882=CARTESIAN_POINT('Ctrl Pts',(65.834356730751,249.961383762869,22.6155675085799)) ;
#112883=CARTESIAN_POINT('Ctrl Pts',(65.8315907501217,249.947263257598,22.5487111276625)) ;
#112884=CARTESIAN_POINT('Ctrl Pts',(65.8288247694925,249.929634851148,22.4825280095449)) ;
#112885=CARTESIAN_POINT('Ctrl Pts',(65.8260587888633,249.908587403347,22.4174130245871)) ;
#112886=CARTESIAN_POINT('Ctrl Pts',(65.8232940214172,249.887549187141,22.3523265996291)) ;
#112887=CARTESIAN_POINT('Ctrl Pts',(65.8205292539712,249.863095057984,22.288307853408)) ;
#112888=CARTESIAN_POINT('Ctrl Pts',(65.8177644865251,249.835363955398,22.2257373011925)) ;
#112889=CARTESIAN_POINT('Ctrl Pts',(65.81499994881,249.807635157054,22.163171948108)) ;
#112890=CARTESIAN_POINT('Ctrl Pts',(65.8122354110949,249.776630130297,22.1020550060658)) ;
#112891=CARTESIAN_POINT('Ctrl Pts',(65.8094708733797,249.742535503141,22.0427459973307)) ;
#112892=CARTESIAN_POINT('Ctrl Pts',(65.8067038695793,249.708410462128,21.9833840824373)) ;
#112893=CARTESIAN_POINT('Ctrl Pts',(65.803936865779,249.671190568739,21.9258337541972)) ;
#112894=CARTESIAN_POINT('Ctrl Pts',(65.8011698619786,249.631107292221,21.8704279097408)) ;
#112895=CARTESIAN_POINT('Ctrl Pts',(65.7984014827221,249.591004090618,21.8149945234684)) ;
#112896=CARTESIAN_POINT('Ctrl Pts',(65.7956331034655,249.548034986855,21.7617081317784)) ;
#112897=CARTESIAN_POINT('Ctrl Pts',(65.792864724209,249.502471713444,21.7108684778389)) ;
#112898=CARTESIAN_POINT('Ctrl Pts',(65.7900918625712,249.456834666917,21.6599465076085)) ;
#112899=CARTESIAN_POINT('Ctrl Pts',(65.7873190009335,249.408595420747,21.6114795351642)) ;
#112900=CARTESIAN_POINT('Ctrl Pts',(65.7845461392957,249.358061767697,21.5657296685664)) ;
#112901=CARTESIAN_POINT('Ctrl Pts',(65.7831826098485,249.333212304215,21.5432325884877)) ;
#112902=CARTESIAN_POINT('Ctrl Pts',(65.7818190804012,249.307808527302,21.5213919009542)) ;
#112903=CARTESIAN_POINT('Ctrl Pts',(65.780455550954,249.28188966256,21.5002349695647)) ;
#112904=CARTESIAN_POINT('Ctrl Pts',(65.7776512670346,249.228583988999,21.4567228601631)) ;
#112905=CARTESIAN_POINT('Ctrl Pts',(65.7748469831152,249.172891043922,21.415936816227)) ;
#112906=CARTESIAN_POINT('Ctrl Pts',(65.7720426991958,249.115120278103,21.3781470073459)) ;
#112907=CARTESIAN_POINT('Ctrl Pts',(65.7691715414723,249.055971851894,21.3394560242798)) ;
#112908=CARTESIAN_POINT('Ctrl Pts',(65.7663003837488,248.994645572091,21.3039064117778)) ;
#112909=CARTESIAN_POINT('Ctrl Pts',(65.7634292260253,248.931510250634,21.2717448678083)) ;
#112910=CARTESIAN_POINT('Ctrl Pts',(65.7606320516086,248.870001785068,21.2404120548264)) ;
#112911=CARTESIAN_POINT('Ctrl Pts',(65.757834877192,248.80677684992,21.2122950400974)) ;
#112912=CARTESIAN_POINT('Ctrl Pts',(65.7550377027753,248.742204519056,21.187577364594)) ;
#112913=CARTESIAN_POINT('Ctrl Pts',(65.7522421065682,248.677668620912,21.1628736351899)) ;
#112914=CARTESIAN_POINT('Ctrl Pts',(65.7494465103611,248.61178729007,21.1415656127727)) ;
#112915=CARTESIAN_POINT('Ctrl Pts',(65.746650914154,248.544950213178,21.1237890014219)) ;
#112916=CARTESIAN_POINT('Ctrl Pts',(65.7438559577247,248.478128432086,21.1060164582841)) ;
#112917=CARTESIAN_POINT('Ctrl Pts',(65.7410610012954,248.410351810289,21.0917738460281)) ;
#112918=CARTESIAN_POINT('Ctrl Pts',(65.7382660448661,248.342024162048,21.0811467113372)) ;
#112919=CARTESIAN_POINT('Ctrl Pts',(65.7353384506133,248.270453947855,21.0700152539309)) ;
#112920=CARTESIAN_POINT('Ctrl Pts',(65.7324108563604,248.198279672005,21.0628511036595)) ;
#112921=CARTESIAN_POINT('Ctrl Pts',(65.7294832621075,248.125973825856,21.0596918706711)) ;
#112922=CARTESIAN_POINT('Ctrl Pts',(65.7266850618879,248.056863758987,21.0566722697024)) ;
#112923=CARTESIAN_POINT('Ctrl Pts',(65.7238868616682,247.987634016768,21.0573109666162)) ;
#112924=CARTESIAN_POINT('Ctrl Pts',(65.7210886614485,247.918696892974,21.0615873466574)) ;
#112925=CARTESIAN_POINT('Ctrl Pts',(65.718288657968,247.849715343617,21.0658664825517)) ;
#112926=CARTESIAN_POINT('Ctrl Pts',(65.7154886544874,247.781027271794,21.0737879112052)) ;
#112927=CARTESIAN_POINT('Ctrl Pts',(65.7126886510069,247.713038099466,21.0852793483774)) ;
#112928=CARTESIAN_POINT('Ctrl Pts',(65.7098843474749,247.644944514076,21.096788433303)) ;
#112929=CARTESIAN_POINT('Ctrl Pts',(65.7070800439429,247.577552443221,21.1118783550534)) ;
#112930=CARTESIAN_POINT('Ctrl Pts',(65.7042757404108,247.511254350599,21.1304264097862)) ;
#112931=CARTESIAN_POINT('Ctrl Pts',(65.7038954648845,247.502264046312,21.1329416051622)) ;
#112932=CARTESIAN_POINT('Ctrl Pts',(65.7035151893581,247.493293830232,21.135520317389)) ;
#112933=CARTESIAN_POINT('Ctrl Pts',(65.7031349138318,247.484344652831,21.1381621723581)) ;
#112934=CARTESIAN_POINT('Ctrl Pts',(65.7003306271379,247.41835024255,21.1576441485133)) ;
#112935=CARTESIAN_POINT('Ctrl Pts',(65.6975263404441,247.353260760904,21.1806349226197)) ;
#112936=CARTESIAN_POINT('Ctrl Pts',(65.6947220537502,247.289473831217,21.2070313067662)) ;
#112937=CARTESIAN_POINT('Ctrl Pts',(65.6918508963735,247.224165846086,21.2340571359106)) ;
#112938=CARTESIAN_POINT('Ctrl Pts',(65.6889797389968,247.160223851577,21.2646530243647)) ;
#112939=CARTESIAN_POINT('Ctrl Pts',(65.6861085816201,247.098059562917,21.2986535269004)) ;
#112940=CARTESIAN_POINT('Ctrl Pts',(65.6833114043199,247.037497039059,21.3317779507521)) ;
#112941=CARTESIAN_POINT('Ctrl Pts',(65.6805142270196,246.978622167724,21.3681333979727)) ;
#112942=CARTESIAN_POINT('Ctrl Pts',(65.6777170497193,246.921794657363,21.4075185894613)) ;
#112943=CARTESIAN_POINT('Ctrl Pts',(65.6749214505969,246.864999209295,21.4468815596785)) ;
#112944=CARTESIAN_POINT('Ctrl Pts',(65.6721258514745,246.810249229733,21.4892706047607)) ;
#112945=CARTESIAN_POINT('Ctrl Pts',(65.6693302523521,246.757876547301,21.5344404459424)) ;
#112946=CARTESIAN_POINT('Ctrl Pts',(65.666535292981,246.705515849955,21.5795999503536)) ;
#112947=CARTESIAN_POINT('Ctrl Pts',(65.6637403336099,246.655531737995,21.6275386685267)) ;
#112948=CARTESIAN_POINT('Ctrl Pts',(65.6609453742388,246.608222586651,21.677971368921)) ;
#112949=CARTESIAN_POINT('Ctrl Pts',(65.658017782778,246.558668425356,21.7307973042619)) ;
#112950=CARTESIAN_POINT('Ctrl Pts',(65.6550901913172,246.512049849452,21.7863594212012)) ;
#112951=CARTESIAN_POINT('Ctrl Pts',(65.6521625998565,246.468664376074,21.84428874242)) ;
#112952=CARTESIAN_POINT('Ctrl Pts',(65.6493643966647,246.42719637355,21.8996578107149)) ;
#112953=CARTESIAN_POINT('Ctrl Pts',(65.646566193473,246.388681951787,21.9571887948497)) ;
#112954=CARTESIAN_POINT('Ctrl Pts',(65.6437679902812,246.353336598711,22.0165295915777)) ;
#112955=CARTESIAN_POINT('Ctrl Pts',(65.6409679838212,246.317968467748,22.075908629766)) ;
#112956=CARTESIAN_POINT('Ctrl Pts',(65.6381679773612,246.285773696671,22.1370993706835)) ;
#112957=CARTESIAN_POINT('Ctrl Pts',(65.6353679709011,246.256921228817,22.1997262470955)) ;
#112958=CARTESIAN_POINT('Ctrl Pts',(65.6325636644005,246.2280244515,22.2624493011828)) ;
#112959=CARTESIAN_POINT('Ctrl Pts',(65.6297593578998,246.202480394273,22.3266124378093)) ;
#112960=CARTESIAN_POINT('Ctrl Pts',(65.6269550513992,246.180409055626,22.3918223568706)) ;
#112961=CARTESIAN_POINT('Ctrl Pts',(65.6265747931693,246.177416227217,22.400664688615)) ;
#112962=CARTESIAN_POINT('Ctrl Pts',(65.6261945349395,246.174487174627,22.4095262496064)) ;
#112963=CARTESIAN_POINT('Ctrl Pts',(65.6258142767096,246.171622124897,22.4184060440952)) ;
#112964=CARTESIAN_POINT('Ctrl Pts',(65.6230100136664,246.150493448529,22.4838912264291)) ;
#112965=CARTESIAN_POINT('Ctrl Pts',(65.6202057506231,246.13277264757,22.5506078742004)) ;
#112966=CARTESIAN_POINT('Ctrl Pts',(65.6174014875799,246.118598747863,22.6181694398748)) ;
#112967=CARTESIAN_POINT('Ctrl Pts',(65.6145303272469,246.104086721718,22.6873427251233)) ;
#112968=CARTESIAN_POINT('Ctrl Pts',(65.6116591669139,246.093293244499,22.7574012971836)) ;
#112969=CARTESIAN_POINT('Ctrl Pts',(65.6087880065809,246.086313879054,22.8279118490807)) ;
#112970=CARTESIAN_POINT('Ctrl Pts',(65.6059908529616,246.079514412967,22.8966049287275)) ;
#112971=CARTESIAN_POINT('Ctrl Pts',(65.6031936993423,246.076334850784,22.9657264507413)) ;
#112972=CARTESIAN_POINT('Ctrl Pts',(65.6003965457231,246.076811831283,23.034865859025)) ;
#112973=CARTESIAN_POINT('Ctrl Pts',(65.5976009702251,246.077288542675,23.1039662596639)) ;
#112974=CARTESIAN_POINT('Ctrl Pts',(65.5948053947272,246.081417699443,23.1730840400311)) ;
#112975=CARTESIAN_POINT('Ctrl Pts',(65.5920098192293,246.089183882217,23.2418068538744)) ;
#112976=CARTESIAN_POINT('Ctrl Pts',(65.5892148833862,246.096948288012,23.310513943269)) ;
#112977=CARTESIAN_POINT('Ctrl Pts',(65.5864199475432,246.108348011975,23.3788257615127)) ;
#112978=CARTESIAN_POINT('Ctrl Pts',(65.5836250117002,246.123315775349,23.44633505727)) ;
#112979=CARTESIAN_POINT('Ctrl Pts',(65.5806973973574,246.138994073956,23.5170490892284)) ;
#112980=CARTESIAN_POINT('Ctrl Pts',(65.5777697830147,246.158587523414,23.5868819323492)) ;
#112981=CARTESIAN_POINT('Ctrl Pts',(65.574842168672,246.181959195878,23.6553797948474)) ;
#112982=CARTESIAN_POINT('Ctrl Pts',(65.5720439884921,246.204297572112,23.7208492654699)) ;
#112983=CARTESIAN_POINT('Ctrl Pts',(65.5692458083123,246.230086890269,23.7850988572933)) ;
#112984=CARTESIAN_POINT('Ctrl Pts',(65.5664476281324,246.25915790344,23.8477520567871)) ;
#112985=CARTESIAN_POINT('Ctrl Pts',(65.5636476444843,246.288247653306,23.9104456371874)) ;
#112986=CARTESIAN_POINT('Ctrl Pts',(65.5608476608363,246.320623079513,23.9715403472528)) ;
#112987=CARTESIAN_POINT('Ctrl Pts',(65.5580476771882,246.356069309894,24.0306848784831)) ;
#112988=CARTESIAN_POINT('Ctrl Pts',(65.5552433930587,246.39156998197,24.0899202495158)) ;
#112989=CARTESIAN_POINT('Ctrl Pts',(65.5524391089292,246.430150593162,24.1471990646923)) ;
#112990=CARTESIAN_POINT('Ctrl Pts',(65.5496348247996,246.471554025327,24.2022004347507)) ;
#112991=CARTESIAN_POINT('Ctrl Pts',(65.5492544297289,246.47717031126,24.2096612515182)) ;
#112992=CARTESIAN_POINT('Ctrl Pts',(65.5488740346582,246.48283848028,24.2170802156454)) ;
#112993=CARTESIAN_POINT('Ctrl Pts',(65.5484936395874,246.488557837358,24.2244565772841)) ;
#112994=CARTESIAN_POINT('Ctrl Pts',(65.5456893322833,246.530721461607,24.278835790927)) ;
#112995=CARTESIAN_POINT('Ctrl Pts',(65.5428850249792,246.575823976354,24.3310951424919)) ;
#112996=CARTESIAN_POINT('Ctrl Pts',(65.5400807176752,246.623624558968,24.3809018252824)) ;
#112997=CARTESIAN_POINT('Ctrl Pts',(65.5372095628748,246.672564584918,24.4318957716942)) ;
#112998=CARTESIAN_POINT('Ctrl Pts',(65.5343384080743,246.724332718666,24.4803181537042)) ;
#112999=CARTESIAN_POINT('Ctrl Pts',(65.5314672532739,246.778625028474,24.5258457040215)) ;
#113000=CARTESIAN_POINT('Ctrl Pts',(65.5286700558685,246.831518835561,24.5702005209769)) ;
#113001=CARTESIAN_POINT('Ctrl Pts',(65.5258728584631,246.886807944199,24.6118075140883)) ;
#113002=CARTESIAN_POINT('Ctrl Pts',(65.5230756610576,246.944173965852,24.6504048897309)) ;
#113003=CARTESIAN_POINT('Ctrl Pts',(65.5202800420725,247.001507616642,24.6889804854009)) ;
#113004=CARTESIAN_POINT('Ctrl Pts',(65.5174844230875,247.06091545103,24.7245495622436)) ;
#113005=CARTESIAN_POINT('Ctrl Pts',(65.5146888041024,247.122048244245,24.7568923073538)) ;
#113006=CARTESIAN_POINT('Ctrl Pts',(65.5118938251428,247.183167041794,24.7892276479561)) ;
#113007=CARTESIAN_POINT('Ctrl Pts',(65.5090988461833,247.246009583031,24.8183378962652)) ;
#113008=CARTESIAN_POINT('Ctrl Pts',(65.5063038672238,247.310201604617,24.8440489386447)) ;
#113009=CARTESIAN_POINT('Ctrl Pts',(65.5033762951605,247.377438879672,24.8709797064522)) ;
#113010=CARTESIAN_POINT('Ctrl Pts',(65.5004487230973,247.446156338146,24.8941804696778)) ;
#113011=CARTESIAN_POINT('Ctrl Pts',(65.4975211510341,247.515902043533,24.9135083962772)) ;
#113012=CARTESIAN_POINT('Ctrl Pts',(65.4947229291615,247.582566144064,24.9319823486838)) ;
#113013=CARTESIAN_POINT('Ctrl Pts',(65.4919247072889,247.650169032401,24.9469184298479)) ;
#113014=CARTESIAN_POINT('Ctrl Pts',(65.4891264854162,247.718304323777,24.9582440652276)) ;
#113015=CARTESIAN_POINT('Ctrl Pts',(65.4863264606051,247.786483515794,24.9695769978927)) ;
#113016=CARTESIAN_POINT('Ctrl Pts',(65.483526435794,247.855195309575,24.9772948007758)) ;
#113017=CARTESIAN_POINT('Ctrl Pts',(65.480726410983,247.924028403685,24.9813767913742)) ;
#113018=CARTESIAN_POINT('Ctrl Pts',(65.4779220867216,247.992967191311,24.9854650498871)) ;
#113019=CARTESIAN_POINT('Ctrl Pts',(65.4751177624602,248.062027164623,24.9859063585679)) ;
#113020=CARTESIAN_POINT('Ctrl Pts',(65.4723134381988,248.130798317154,24.9827320769806)) ;
#113021=CARTESIAN_POINT('Ctrl Pts',(65.4719332929543,248.14012071505,24.982301781502)) ;
#113022=CARTESIAN_POINT('Ctrl Pts',(65.4715531477098,248.149437816945,24.9818051247629)) ;
#113023=CARTESIAN_POINT('Ctrl Pts',(65.4711730024652,248.158748613648,24.9812422575242)) ;
#113024=CARTESIAN_POINT('Ctrl Pts',(65.4683686909079,248.227433873243,24.9770900153864)) ;
#113025=CARTESIAN_POINT('Ctrl Pts',(65.4655643793505,248.296025884377,24.9693152890749)) ;
#113026=CARTESIAN_POINT('Ctrl Pts',(65.4627600677932,248.364113998153,24.9579292731601)) ;
#113027=CARTESIAN_POINT('Ctrl Pts',(65.4598889135244,248.433825039354,24.9462718636571)) ;
#113028=CARTESIAN_POINT('Ctrl Pts',(65.4570177592556,248.503007334162,24.930828737252)) ;
#113029=CARTESIAN_POINT('Ctrl Pts',(65.4541466049869,248.571222524517,24.9116685843919)) ;
#113030=CARTESIAN_POINT('Ctrl Pts',(65.4513494019349,248.637680722439,24.8930019322235)) ;
#113031=CARTESIAN_POINT('Ctrl Pts',(65.4485521988829,248.7032205353,24.8708075687884)) ;
#113032=CARTESIAN_POINT('Ctrl Pts',(65.4457549958309,248.7674462161,24.8452007907684)) ;
#113033=CARTESIAN_POINT('Ctrl Pts',(65.4429593707037,248.831635666677,24.819608457738)) ;
#113034=CARTESIAN_POINT('Ctrl Pts',(65.4401637455764,248.894512004406,24.7906077103815)) ;
#113035=CARTESIAN_POINT('Ctrl Pts',(65.4373681204492,248.955696761178,24.7583629849385)) ;
#113036=CARTESIAN_POINT('Ctrl Pts',(65.4345731348665,249.016867520945,24.7261256359989)) ;
#113037=CARTESIAN_POINT('Ctrl Pts',(65.4317781492838,249.07634703746,24.6906460103184)) ;
#113038=CARTESIAN_POINT('Ctrl Pts',(65.4289831637011,249.133780461819,24.6521349928972)) ;
#113039=CARTESIAN_POINT('Ctrl Pts',(65.4260555971713,249.193938257225,24.6117971942588)) ;
#113040=CARTESIAN_POINT('Ctrl Pts',(65.4231280306415,249.251850509562,24.5681335429293)) ;
#113041=CARTESIAN_POINT('Ctrl Pts',(65.4202004641116,249.307144404721,24.5214367047118)) ;
#113042=CARTESIAN_POINT('Ctrl Pts',(65.4174022345049,249.359995471616,24.4768028854939)) ;
#113043=CARTESIAN_POINT('Ctrl Pts',(65.4146040048982,249.410454327204,24.4293986304115)) ;
#113044=CARTESIAN_POINT('Ctrl Pts',(65.4118057752914,249.458231860769,24.3795186123828)) ;
#113045=CARTESIAN_POINT('Ctrl Pts',(65.4090057423723,249.506040184452,24.3296064492953)) ;
#113046=CARTESIAN_POINT('Ctrl Pts',(65.4062057094532,249.551163429357,24.277215716978)) ;
#113047=CARTESIAN_POINT('Ctrl Pts',(65.403405676534,249.593352565439,24.2226744124676)) ;
#113048=CARTESIAN_POINT('Ctrl Pts',(65.4006013436993,249.635606489946,24.1680493507246)) ;
#113049=CARTESIAN_POINT('Ctrl Pts',(65.3977970108645,249.674917042458,24.1112675297942)) ;
#113050=CARTESIAN_POINT('Ctrl Pts',(65.3949926780297,249.711078900409,24.0526852258304)) ;
#113051=CARTESIAN_POINT('Ctrl Pts',(65.3946125738008,249.715980342549,24.0447448768113)) ;
#113052=CARTESIAN_POINT('Ctrl Pts',(65.394232469572,249.720824008609,24.0367714845135)) ;
#113053=CARTESIAN_POINT('Ctrl Pts',(65.3938523653431,249.725609454111,24.0287659670596)) ;
#113054=CARTESIAN_POINT('Ctrl Pts',(65.3909709021382,249.761886569934,23.9680783918435)) ;
#113055=CARTESIAN_POINT('Ctrl Pts',(65.3880894389332,249.794939945734,23.9053322650928)) ;
#113056=CARTESIAN_POINT('Ctrl Pts',(65.3852079757282,249.824539173868,23.8408923703566)) ;
#113057=CARTESIAN_POINT('Ctrl Pts',(65.3823327770366,249.854074051099,23.776592572699)) ;
#113058=CARTESIAN_POINT('Ctrl Pts',(65.3794575783449,249.880169538016,23.710606740984)) ;
#113059=CARTESIAN_POINT('Ctrl Pts',(65.3765823796533,249.90264063787,23.6433248732417)) ;
#113060=CARTESIAN_POINT('Ctrl Pts',(65.3737108851966,249.925082787295,23.5761296874564)) ;
#113061=CARTESIAN_POINT('Ctrl Pts',(65.3708393907399,249.943909684919,23.5076422072702)) ;
#113062=CARTESIAN_POINT('Ctrl Pts',(65.3679678962833,249.958984224268,23.4382726214603)) ;
#113063=CARTESIAN_POINT('Ctrl Pts',(65.3650999636564,249.974040065011,23.3689890823635)) ;
#113064=CARTESIAN_POINT('Ctrl Pts',(65.3622320310296,249.985352710673,23.2988260522388)) ;
#113065=CARTESIAN_POINT('Ctrl Pts',(65.3593640984028,249.992835185236,23.2282076139426)) ;
#113066=CARTESIAN_POINT('Ctrl Pts',(65.356568695154,250.000128429683,23.1593751002392)) ;
#113067=CARTESIAN_POINT('Ctrl Pts',(65.3537732919052,250.00378290197,23.0901103612602)) ;
#113068=CARTESIAN_POINT('Ctrl Pts',(65.3509778886564,250.003765042576,23.0208142986557)) ;
#113069=CARTESIAN_POINT('',(64.9402651077866,248.893109917435,24.7899322231574)) ;
#113070=CARTESIAN_POINT('Ctrl Pts',(65.3509778886241,250.003765042575,23.0208142978541)) ;
#113071=CARTESIAN_POINT('Ctrl Pts',(65.3479806653745,250.003745893754,22.946515260666)) ;
#113072=CARTESIAN_POINT('Ctrl Pts',(65.344983442125,249.999505258812,22.8723256198793)) ;
#113073=CARTESIAN_POINT('Ctrl Pts',(65.3419862188755,249.99110566956,22.7987145203243)) ;
#113074=CARTESIAN_POINT('Ctrl Pts',(65.338982572516,249.982688079818,22.7249456706965)) ;
#113075=CARTESIAN_POINT('Ctrl Pts',(65.3359789261565,249.970093813032,22.6517582009852)) ;
#113076=CARTESIAN_POINT('Ctrl Pts',(65.332975279797,249.953436469231,22.579610493379)) ;
#113077=CARTESIAN_POINT('Ctrl Pts',(65.3299608740215,249.936719456857,22.5072043441616)) ;
#113078=CARTESIAN_POINT('Ctrl Pts',(65.3269464682459,249.915910352595,22.4358457658401)) ;
#113079=CARTESIAN_POINT('Ctrl Pts',(65.3239320624703,249.891172956104,22.3659789157249)) ;
#113080=CARTESIAN_POINT('Ctrl Pts',(65.3214652843872,249.870929607317,22.3088047900646)) ;
#113081=CARTESIAN_POINT('Ctrl Pts',(65.318998506304,249.84805658175,22.2526293393555)) ;
#113082=CARTESIAN_POINT('Ctrl Pts',(65.3165317282209,249.822666742645,22.1976840997892)) ;
#113083=CARTESIAN_POINT('Ctrl Pts',(65.3137271110147,249.793799622371,22.1352138008449)) ;
#113084=CARTESIAN_POINT('Ctrl Pts',(65.3109224938086,249.761591747449,22.0741490767129)) ;
#113085=CARTESIAN_POINT('Ctrl Pts',(65.3081178766025,249.726203045599,22.0148683974425)) ;
#113086=CARTESIAN_POINT('Ctrl Pts',(65.3052467605398,249.689975260183,21.954182144044)) ;
#113087=CARTESIAN_POINT('Ctrl Pts',(65.3023756444771,249.650414014378,21.8953661231801)) ;
#113088=CARTESIAN_POINT('Ctrl Pts',(65.2995045284145,249.607742790949,21.8388035518035)) ;
#113089=CARTESIAN_POINT('Ctrl Pts',(65.2967070251196,249.566165618334,21.7836911925892)) ;
#113090=CARTESIAN_POINT('Ctrl Pts',(65.2939095218248,249.521636347261,21.7307185271669)) ;
#113091=CARTESIAN_POINT('Ctrl Pts',(65.2911120185299,249.474406437266,21.6802122580281)) ;
#113092=CARTESIAN_POINT('Ctrl Pts',(65.288316096009,249.427203215285,21.6297345282628)) ;
#113093=CARTESIAN_POINT('Ctrl Pts',(65.285520173488,249.377302715022,21.581720784283)) ;
#113094=CARTESIAN_POINT('Ctrl Pts',(65.2827242509671,249.324995877752,21.5364637515943)) ;
#113095=CARTESIAN_POINT('Ctrl Pts',(65.2799289713297,249.272701067712,21.4912171251316)) ;
#113096=CARTESIAN_POINT('Ctrl Pts',(65.2771336916922,249.218001388152,21.4487262694942)) ;
#113097=CARTESIAN_POINT('Ctrl Pts',(65.2743384120548,249.161222449624,21.4092450079194)) ;
#113098=CARTESIAN_POINT('Ctrl Pts',(65.2714111353085,249.101762328279,21.3678993846132)) ;
#113099=CARTESIAN_POINT('Ctrl Pts',(65.2684838585621,249.040022161171,21.3298549998709)) ;
#113100=CARTESIAN_POINT('Ctrl Pts',(65.2655565818158,248.976410028725,21.2953525173818)) ;
#113101=CARTESIAN_POINT('Ctrl Pts',(65.2627580699,248.915596062002,21.2623677275113)) ;
#113102=CARTESIAN_POINT('Ctrl Pts',(65.2599595579842,248.853071848854,21.2326199409251)) ;
#113103=CARTESIAN_POINT('Ctrl Pts',(65.2571610460684,248.789217120396,21.2062712718244)) ;
#113104=CARTESIAN_POINT('Ctrl Pts',(65.2543607351569,248.725321343559,21.1799056647423)) ;
#113105=CARTESIAN_POINT('Ctrl Pts',(65.2515604242454,248.660093808458,21.1569436855658)) ;
#113106=CARTESIAN_POINT('Ctrl Pts',(65.2487601133339,248.593930706755,21.137497991394)) ;
#113107=CARTESIAN_POINT('Ctrl Pts',(65.2459555105135,248.527666199883,21.1180224936936)) ;
#113108=CARTESIAN_POINT('Ctrl Pts',(65.2431509076932,248.460463739478,21.1020741416983)) ;
#113109=CARTESIAN_POINT('Ctrl Pts',(65.2403463048729,248.392729959331,21.0897145922673)) ;
#113110=CARTESIAN_POINT('Ctrl Pts',(65.2399679002815,248.383591134676,21.0880470084589)) ;
#113111=CARTESIAN_POINT('Ctrl Pts',(65.2395894956901,248.374442644214,21.0864446783139)) ;
#113112=CARTESIAN_POINT('Ctrl Pts',(65.2392110910987,248.365285491174,21.0849076808294)) ;
#113113=CARTESIAN_POINT('Ctrl Pts',(65.2364067177151,248.297421419652,21.0735169235961)) ;
#113114=CARTESIAN_POINT('Ctrl Pts',(65.2336023443314,248.228834175757,21.0656772442728)) ;
#113115=CARTESIAN_POINT('Ctrl Pts',(65.2307979709478,248.159926453501,21.0614699889811)) ;
#113116=CARTESIAN_POINT('Ctrl Pts',(65.2279268244073,248.089378013155,21.0571625574008)) ;
#113117=CARTESIAN_POINT('Ctrl Pts',(65.2250556778669,248.018494129241,21.056662923935)) ;
#113118=CARTESIAN_POINT('Ctrl Pts',(65.2221845313264,247.947717379197,21.060002631425)) ;
#113119=CARTESIAN_POINT('Ctrl Pts',(65.2193872581074,247.878761683402,21.063256409729)) ;
#113120=CARTESIAN_POINT('Ctrl Pts',(65.2165899848883,247.809908193841,21.0701543074036)) ;
#113121=CARTESIAN_POINT('Ctrl Pts',(65.2137927116693,247.741568468735,21.0806728825766)) ;
#113122=CARTESIAN_POINT('Ctrl Pts',(65.210997013543,247.673267224463,21.0911855349348)) ;
#113123=CARTESIAN_POINT('Ctrl Pts',(65.2082013154167,247.60547965136,21.1053147449279)) ;
#113124=CARTESIAN_POINT('Ctrl Pts',(65.2054056172904,247.538611509456,21.1229853053531)) ;
#113125=CARTESIAN_POINT('Ctrl Pts',(65.2026105560488,247.471758600705,21.1406518402685)) ;
#113126=CARTESIAN_POINT('Ctrl Pts',(65.1998154948073,247.405825178078,21.16185799854)) ;
#113127=CARTESIAN_POINT('Ctrl Pts',(65.1970204335657,247.341204421173,21.1864780052558)) ;
#113128=CARTESIAN_POINT('Ctrl Pts',(65.1940929352666,247.273521769676,21.2122645700411)) ;
#113129=CARTESIAN_POINT('Ctrl Pts',(65.1911654369675,247.207279828497,21.241796374246)) ;
#113130=CARTESIAN_POINT('Ctrl Pts',(65.1882379386684,247.142907594777,21.274872020864)) ;
#113131=CARTESIAN_POINT('Ctrl Pts',(65.1854396278421,247.081376041167,21.3064880733985)) ;
#113132=CARTESIAN_POINT('Ctrl Pts',(65.1826413170157,247.021553062989,21.3413414715165)) ;
#113133=CARTESIAN_POINT('Ctrl Pts',(65.1798430061894,246.963786608865,21.3792100271189)) ;
#113134=CARTESIAN_POINT('Ctrl Pts',(65.1770428902427,246.905982891044,21.4171030107807)) ;
#113135=CARTESIAN_POINT('Ctrl Pts',(65.1742427742959,246.850238730028,21.4580147346589)) ;
#113136=CARTESIAN_POINT('Ctrl Pts',(65.1714426583492,246.796870506239,21.5016815329066)) ;
#113137=CARTESIAN_POINT('Ctrl Pts',(65.1686382405898,246.743420292952,21.5454154163703)) ;
#113138=CARTESIAN_POINT('Ctrl Pts',(65.1658338228304,246.692353656227,21.5919124885469)) ;
#113139=CARTESIAN_POINT('Ctrl Pts',(65.1630294050711,246.643950741133,21.640871706529)) ;
#113140=CARTESIAN_POINT('Ctrl Pts',(65.1626497547062,246.637398156621,21.6474996010029)) ;
#113141=CARTESIAN_POINT('Ctrl Pts',(65.1622701043414,246.630894328402,21.6541725690334)) ;
#113142=CARTESIAN_POINT('Ctrl Pts',(65.1618904539765,246.624439893596,21.6608898187387)) ;
#113143=CARTESIAN_POINT('Ctrl Pts',(65.159088027919,246.576795855917,21.7104738501322)) ;
#113144=CARTESIAN_POINT('Ctrl Pts',(65.1562856018614,246.531672008957,21.7626549423151)) ;
#113145=CARTESIAN_POINT('Ctrl Pts',(65.1534831758038,246.489362512684,21.8171470211069)) ;
#113146=CARTESIAN_POINT('Ctrl Pts',(65.1506117858476,246.446011837179,21.8729800759395)) ;
#113147=CARTESIAN_POINT('Ctrl Pts',(65.1477403958914,246.405616285875,21.9312390567331)) ;
#113148=CARTESIAN_POINT('Ctrl Pts',(65.1448690059351,246.368452042583,21.9915760427659)) ;
#113149=CARTESIAN_POINT('Ctrl Pts',(65.1420736961978,246.332272501406,22.0503143427368)) ;
#113150=CARTESIAN_POINT('Ctrl Pts',(65.1392783864604,246.299155428829,22.1110214496346)) ;
#113151=CARTESIAN_POINT('Ctrl Pts',(65.136483076723,246.269313470916,22.1733447838484)) ;
#113152=CARTESIAN_POINT('Ctrl Pts',(65.1336893424598,246.239488332333,22.2356329917911)) ;
#113153=CARTESIAN_POINT('Ctrl Pts',(65.1308956081967,246.212934855869,22.299535179937)) ;
#113154=CARTESIAN_POINT('Ctrl Pts',(65.1281018739335,246.189819680115,22.3646743436401)) ;
#113155=CARTESIAN_POINT('Ctrl Pts',(65.1253087736113,246.166709749546,22.4297987262746)) ;
#113156=CARTESIAN_POINT('Ctrl Pts',(65.122515673289,246.147036733082,22.4961590670286)) ;
#113157=CARTESIAN_POINT('Ctrl Pts',(65.1197225729667,246.130918419439,22.5633602211707)) ;
#113158=CARTESIAN_POINT('Ctrl Pts',(65.116793176624,246.114013574075,22.6338406165929)) ;
#113159=CARTESIAN_POINT('Ctrl Pts',(65.1138637802813,246.101019404348,22.7052454260632)) ;
#113160=CARTESIAN_POINT('Ctrl Pts',(65.1109343839386,246.092011701315,22.7771054501234)) ;
#113161=CARTESIAN_POINT('Ctrl Pts',(65.1081380037395,246.083413014264,22.8457025004649)) ;
#113162=CARTESIAN_POINT('Ctrl Pts',(65.1053416235404,246.078446591114,22.9147138070442)) ;
#113163=CARTESIAN_POINT('Ctrl Pts',(65.1025452433413,246.07712501953,22.9837272074345)) ;
#113164=CARTESIAN_POINT('Ctrl Pts',(65.0997470457728,246.075802589056,23.0527854596817)) ;
#113165=CARTESIAN_POINT('Ctrl Pts',(65.0969488482042,246.078129707593,23.1218453209855)) ;
#113166=CARTESIAN_POINT('Ctrl Pts',(65.0941506506357,246.084066908575,23.1904973378721)) ;
#113167=CARTESIAN_POINT('Ctrl Pts',(65.0913481205674,246.090013302233,23.2592556499141)) ;
#113168=CARTESIAN_POINT('Ctrl Pts',(65.0885455904991,246.099580858384,23.3276043760247)) ;
#113169=CARTESIAN_POINT('Ctrl Pts',(65.0857430604308,246.11267881539,23.3951429423531)) ;
#113170=CARTESIAN_POINT('Ctrl Pts',(65.0853519792387,246.114506579773,23.4045676630132)) ;
#113171=CARTESIAN_POINT('Ctrl Pts',(65.0849608980465,246.116403012254,23.4139766312272)) ;
#113172=CARTESIAN_POINT('Ctrl Pts',(65.0845698168544,246.118367789474,23.4233687832602)) ;
#113173=CARTESIAN_POINT('Ctrl Pts',(65.0817617749785,246.132475286387,23.4908063301007)) ;
#113174=CARTESIAN_POINT('Ctrl Pts',(65.0789537331027,246.150161857754,23.5576217390252)) ;
#113175=CARTESIAN_POINT('Ctrl Pts',(65.0761456912268,246.171356111447,23.6234095507392)) ;
#113176=CARTESIAN_POINT('Ctrl Pts',(65.0732750032479,246.193023199043,23.6906650578138)) ;
#113177=CARTESIAN_POINT('Ctrl Pts',(65.0704043152689,246.218356349094,23.7568460451602)) ;
#113178=CARTESIAN_POINT('Ctrl Pts',(65.06753362729,246.247223855661,23.8215298899763)) ;
#113179=CARTESIAN_POINT('Ctrl Pts',(65.0647327104559,246.275389746797,23.8846416148205)) ;
#113180=CARTESIAN_POINT('Ctrl Pts',(65.0619317936218,246.306919924558,23.9463276777269)) ;
#113181=CARTESIAN_POINT('Ctrl Pts',(65.0591308767876,246.341642271617,24.0062125764685)) ;
#113182=CARTESIAN_POINT('Ctrl Pts',(65.0563315545494,246.376344850823,24.0660633820118)) ;
#113183=CARTESIAN_POINT('Ctrl Pts',(65.0535322323112,246.414235749193,24.1241146389114)) ;
#113184=CARTESIAN_POINT('Ctrl Pts',(65.050732910073,246.455096751985,24.1800150979131)) ;
#113185=CARTESIAN_POINT('Ctrl Pts',(65.0479342501967,246.495948086445,24.2359023300204)) ;
#113186=CARTESIAN_POINT('Ctrl Pts',(65.0451355903205,246.539767842544,24.2896393830908)) ;
#113187=CARTESIAN_POINT('Ctrl Pts',(65.0423369304442,246.586295282531,24.3409051256965)) ;
#113188=CARTESIAN_POINT('Ctrl Pts',(65.0394129512182,246.634906144149,24.3944664632699)) ;
#113189=CARTESIAN_POINT('Ctrl Pts',(65.0364889719922,246.686472537509,24.4453295045976)) ;
#113190=CARTESIAN_POINT('Ctrl Pts',(65.0335649927662,246.740652762921,24.4931695216599)) ;
#113191=CARTESIAN_POINT('Ctrl Pts',(65.0307631881786,246.792569138649,24.539010606331)) ;
#113192=CARTESIAN_POINT('Ctrl Pts',(65.027961383591,246.846884824809,24.582075998955)) ;
#113193=CARTESIAN_POINT('Ctrl Pts',(65.0251595790034,246.903265782795,24.6221216382147)) ;
#113194=CARTESIAN_POINT('Ctrl Pts',(65.0223560087871,246.959682270682,24.6621925132574)) ;
#113195=CARTESIAN_POINT('Ctrl Pts',(65.0195524385707,247.01816621078,24.6992395871625)) ;
#113196=CARTESIAN_POINT('Ctrl Pts',(65.0167488683544,247.078356350065,24.7330632541101)) ;
#113197=CARTESIAN_POINT('Ctrl Pts',(65.0139410755972,247.138637143516,24.7669378638926)) ;
#113198=CARTESIAN_POINT('Ctrl Pts',(65.01113328284,247.200628827093,24.7975791686121)) ;
#113199=CARTESIAN_POINT('Ctrl Pts',(65.0083254900828,247.263948441857,24.8248348802908)) ;
#113200=CARTESIAN_POINT('Ctrl Pts',(65.0079667199659,247.272039204799,24.828317521536)) ;
#113201=CARTESIAN_POINT('Ctrl Pts',(65.0076079498491,247.280151627297,24.8317449531255)) ;
#113202=CARTESIAN_POINT('Ctrl Pts',(65.0072491797322,247.288284892852,24.8351169160415)) ;
#113203=CARTESIAN_POINT('Ctrl Pts',(65.0044581767345,247.351556518543,24.8613486398238)) ;
#113204=CARTESIAN_POINT('Ctrl Pts',(65.0016671737367,247.416335160015,24.8843205302459)) ;
#113205=CARTESIAN_POINT('Ctrl Pts',(64.998876170739,247.482246594188,24.9038578832867)) ;
#113206=CARTESIAN_POINT('Ctrl Pts',(64.9961177591618,247.547388359798,24.9231670925065)) ;
#113207=CARTESIAN_POINT('Ctrl Pts',(64.9933593475846,247.613636117047,24.9391213744491)) ;
#113208=CARTESIAN_POINT('Ctrl Pts',(64.9906009360073,247.680607235827,24.9515997184528)) ;
#113209=CARTESIAN_POINT('Ctrl Pts',(64.9878449341485,247.747519849367,24.964067161511)) ;
#113210=CARTESIAN_POINT('Ctrl Pts',(64.9850889322896,247.815154078844,24.973064593714)) ;
#113211=CARTESIAN_POINT('Ctrl Pts',(64.9823329304307,247.883114119084,24.9785213594877)) ;
#113212=CARTESIAN_POINT('Ctrl Pts',(64.9795783404483,247.951039343968,24.9839753298063)) ;
#113213=CARTESIAN_POINT('Ctrl Pts',(64.976823750466,248.019289547218,24.9858921913326)) ;
#113214=CARTESIAN_POINT('Ctrl Pts',(64.9740691604836,248.087462725763,24.9842530053841)) ;
#113215=CARTESIAN_POINT('Ctrl Pts',(64.9712521560922,248.15718059469,24.9825766782192)) ;
#113216=CARTESIAN_POINT('Ctrl Pts',(64.9684351517008,248.22681736079,24.9771811280954)) ;
#113217=CARTESIAN_POINT('Ctrl Pts',(64.9656181473094,248.295943906619,24.9681024581855)) ;
#113218=CARTESIAN_POINT('Ctrl Pts',(64.9628620383367,248.363576138146,24.9592200426397)) ;
#113219=CARTESIAN_POINT('Ctrl Pts',(64.960105929364,248.430719486793,24.9468123031796)) ;
#113220=CARTESIAN_POINT('Ctrl Pts',(64.9573498203913,248.496980533019,24.9309651457034)) ;
#113221=CARTESIAN_POINT('Ctrl Pts',(64.9545023682905,248.565437606793,24.9145927807882)) ;
#113222=CARTESIAN_POINT('Ctrl Pts',(64.9516549161897,248.632952297457,24.8945491272306)) ;
#113223=CARTESIAN_POINT('Ctrl Pts',(64.9488074640889,248.699108485264,24.8709845438818)) ;
#113224=CARTESIAN_POINT('Ctrl Pts',(64.9459600119882,248.765264673071,24.847419960533)) ;
#113225=CARTESIAN_POINT('Ctrl Pts',(64.9431125598874,248.830061837789,24.8203347258801)) ;
#113226=CARTESIAN_POINT('Ctrl Pts',(64.9402651077866,248.893109917435,24.7899322231574)) ;
#113227=CARTESIAN_POINT('Ctrl Pts',(64.9402651077866,248.893109917435,24.7899322231574)) ;
#113228=CARTESIAN_POINT('Ctrl Pts',(64.9402651077866,248.904085124906,24.7845127825723)) ;
#113229=CARTESIAN_POINT('Ctrl Pts',(64.9402651077866,248.915060332378,24.7790933419871)) ;
#113230=CARTESIAN_POINT('Ctrl Pts',(64.9402651077866,248.926035539849,24.773673901402)) ;
#113231=CARTESIAN_POINT('',(57.9402651077866,248.936544011728,24.7683224547054)) ;
#113232=CARTESIAN_POINT('',(57.9402651077866,247.188367839728,24.7903888257488)) ;
#113233=CARTESIAN_POINT('Origin',(57.9402651077866,248.040265107786,23.0213203435596)) ;
#113234=CARTESIAN_POINT('',(58.2795523269168,250.003764327853,23.0195702593774)) ;
#113235=CARTESIAN_POINT('Ctrl Pts',(57.9402651077866,247.188367839728,24.7903888257487)) ;
#113236=CARTESIAN_POINT('Ctrl Pts',(57.9666399231151,246.602035381373,24.5080396547158)) ;
#113237=CARTESIAN_POINT('Ctrl Pts',(58.0193895537721,245.742675425061,23.3177389351249)) ;
#113238=CARTESIAN_POINT('Ctrl Pts',(58.0985139997576,246.538528075967,21.2534684972079)) ;
#113239=CARTESIAN_POINT('Ctrl Pts',(58.1776384457431,248.70384260527,20.8001158056293)) ;
#113240=CARTESIAN_POINT('Ctrl Pts',(58.2379844498895,249.893805686828,21.994549066635)) ;
#113241=CARTESIAN_POINT('Ctrl Pts',(58.2719556387072,250.004418999133,22.8319096049426)) ;
#113242=CARTESIAN_POINT('Ctrl Pts',(58.2795520121964,250.002860502623,23.019563290465)) ;
#113243=CARTESIAN_POINT('',(58.7795523269483,250.003764821541,23.0223805714202)) ;
#113244=CARTESIAN_POINT('Ctrl Pts',(58.2795523269168,250.003764327853,23.0195702593774)) ;
#113245=CARTESIAN_POINT('Ctrl Pts',(58.2823182633917,250.003825255953,23.0879282718707)) ;
#113246=CARTESIAN_POINT('Ctrl Pts',(58.2850841998665,250.000312138262,23.1563562695139)) ;
#113247=CARTESIAN_POINT('Ctrl Pts',(58.2878501363414,249.993229751855,23.2244492410987)) ;
#113248=CARTESIAN_POINT('Ctrl Pts',(58.2906148535111,249.98615048757,23.2925121953241)) ;
#113249=CARTESIAN_POINT('Ctrl Pts',(58.2933795706809,249.975505126965,23.360239920402)) ;
#113250=CARTESIAN_POINT('Ctrl Pts',(58.2961442878506,249.961350421642,23.4272310072374)) ;
#113251=CARTESIAN_POINT('Ctrl Pts',(58.2989087672538,249.947196933628,23.4942163328193)) ;
#113252=CARTESIAN_POINT('Ctrl Pts',(58.3016732466571,249.929534804802,23.5604646577782)) ;
#113253=CARTESIAN_POINT('Ctrl Pts',(58.3044377260603,249.90847180973,23.6255851603507)) ;
#113254=CARTESIAN_POINT('Ctrl Pts',(58.3072048962958,249.887388312792,23.6907690485835)) ;
#113255=CARTESIAN_POINT('Ctrl Pts',(58.3099720665314,249.862897492722,23.7548224458987)) ;
#113256=CARTESIAN_POINT('Ctrl Pts',(58.3127392367669,249.835156583672,23.8173711207049)) ;
#113257=CARTESIAN_POINT('Ctrl Pts',(58.3155077613593,249.807402097179,23.8799504091782)) ;
#113258=CARTESIAN_POINT('Ctrl Pts',(58.3182762859518,249.776394581466,23.9410230634081)) ;
#113259=CARTESIAN_POINT('Ctrl Pts',(58.3210448105442,249.742337590698,24.0002388860917)) ;
#113260=CARTESIAN_POINT('Ctrl Pts',(58.3238184206147,249.708218040949,24.0595634817899)) ;
#113261=CARTESIAN_POINT('Ctrl Pts',(58.3265920306851,249.671038101262,24.1170240146228)) ;
#113262=CARTESIAN_POINT('Ctrl Pts',(58.3293656407556,249.631044645718,24.1722993666953)) ;
#113263=CARTESIAN_POINT('Ctrl Pts',(58.3315395397418,249.599698591206,24.2156230599248)) ;
#113264=CARTESIAN_POINT('Ctrl Pts',(58.333713438728,249.566625063434,24.2576049393308)) ;
#113265=CARTESIAN_POINT('Ctrl Pts',(58.3358873377142,249.531959030203,24.2981059527453)) ;
#113266=CARTESIAN_POINT('Ctrl Pts',(58.3386837429993,249.48736621372,24.3502046236985)) ;
#113267=CARTESIAN_POINT('Ctrl Pts',(58.3414801482845,249.439953245343,24.4000665465058)) ;
#113268=CARTESIAN_POINT('Ctrl Pts',(58.3442765535696,249.389973128362,24.4473710120822)) ;
#113269=CARTESIAN_POINT('Ctrl Pts',(58.3470687747069,249.340067794603,24.494604697904)) ;
#113270=CARTESIAN_POINT('Ctrl Pts',(58.3498609958442,249.287603289537,24.5392881866717)) ;
#113271=CARTESIAN_POINT('Ctrl Pts',(58.3526532169815,249.232871932943,24.581134823102)) ;
#113272=CARTESIAN_POINT('Ctrl Pts',(58.3554421775713,249.178204487541,24.6229325941542)) ;
#113273=CARTESIAN_POINT('Ctrl Pts',(58.3582311381612,249.121275836045,24.6618997954725)) ;
#113274=CARTESIAN_POINT('Ctrl Pts',(58.3610200987511,249.062412750517,24.6977887883742)) ;
#113275=CARTESIAN_POINT('Ctrl Pts',(58.3638073250054,249.00358626943,24.7336554634434)) ;
#113276=CARTESIAN_POINT('Ctrl Pts',(58.3665945512598,248.942828158839,24.7664474725727)) ;
#113277=CARTESIAN_POINT('Ctrl Pts',(58.3693817775141,248.880494381143,24.7959603121712)) ;
#113278=CARTESIAN_POINT('Ctrl Pts',(58.3721682218784,248.818178089708,24.8254648726438)) ;
#113279=CARTESIAN_POINT('Ctrl Pts',(58.3749546662426,248.754287452094,24.8516918799336)) ;
#113280=CARTESIAN_POINT('Ctrl Pts',(58.3777411106069,248.689201645731,24.8744834825519)) ;
#113281=CARTESIAN_POINT('Ctrl Pts',(58.3805277243677,248.624111882601,24.8972764707421)) ;
#113282=CARTESIAN_POINT('Ctrl Pts',(58.3833143381285,248.557827270531,24.9166334798408)) ;
#113283=CARTESIAN_POINT('Ctrl Pts',(58.3861009518893,248.490743802197,24.9324459793779)) ;
#113284=CARTESIAN_POINT('Ctrl Pts',(58.388890510028,248.423589452464,24.9482751866391)) ;
#113285=CARTESIAN_POINT('Ctrl Pts',(58.3916800681667,248.355635040572,24.9605522974399)) ;
#113286=CARTESIAN_POINT('Ctrl Pts',(58.3944696263054,248.287287471066,24.9692197768054)) ;
#113287=CARTESIAN_POINT('Ctrl Pts',(58.3972608512449,248.218899062914,24.9778924351134)) ;
#113288=CARTESIAN_POINT('Ctrl Pts',(58.4000520761843,248.150117519127,24.9829511333549)) ;
#113289=CARTESIAN_POINT('Ctrl Pts',(58.4028433011238,248.081352802459,24.9843904012362)) ;
#113290=CARTESIAN_POINT('Ctrl Pts',(58.4056392855601,248.012470830658,24.9858321233056)) ;
#113291=CARTESIAN_POINT('Ctrl Pts',(58.4084352699964,247.943606233485,24.9836421131475)) ;
#113292=CARTESIAN_POINT('Ctrl Pts',(58.4112312544326,247.875166021403,24.977866929173)) ;
#113293=CARTESIAN_POINT('Ctrl Pts',(58.412491430855,247.844319375589,24.9752639995625)) ;
#113294=CARTESIAN_POINT('Ctrl Pts',(58.4137516072774,247.813558825869,24.9719334780948)) ;
#113295=CARTESIAN_POINT('Ctrl Pts',(58.4150117836997,247.782920898768,24.9678830083831)) ;
#113296=CARTESIAN_POINT('Ctrl Pts',(58.4178084842444,247.714926365708,24.958893829846)) ;
#113297=CARTESIAN_POINT('Ctrl Pts',(58.4206051847891,247.647270448959,24.9463201700162)) ;
#113298=CARTESIAN_POINT('Ctrl Pts',(58.4234018853337,247.580360008718,24.9301994779868)) ;
#113299=CARTESIAN_POINT('Ctrl Pts',(58.4261944131009,247.513549401254,24.914102838608)) ;
#113300=CARTESIAN_POINT('Ctrl Pts',(58.428986940868,247.447482535954,24.8944697850432)) ;
#113301=CARTESIAN_POINT('Ctrl Pts',(58.4317794686352,247.382559132849,24.8713892883646)) ;
#113302=CARTESIAN_POINT('Ctrl Pts',(58.4345687511967,247.317711177444,24.8483356136071)) ;
#113303=CARTESIAN_POINT('Ctrl Pts',(58.4373580337581,247.254004505233,24.8218426162695)) ;
#113304=CARTESIAN_POINT('Ctrl Pts',(58.4401473163196,247.191824888038,24.7920494147372)) ;
#113305=CARTESIAN_POINT('Ctrl Pts',(58.4429348738925,247.129683724863,24.7622746383484)) ;
#113306=CARTESIAN_POINT('Ctrl Pts',(58.4457224314654,247.06906818475,24.7292039182264)) ;
#113307=CARTESIAN_POINT('Ctrl Pts',(58.4485099890383,247.010343770323,24.6930243510438)) ;
#113308=CARTESIAN_POINT('Ctrl Pts',(58.4512967735691,246.95163564128,24.6568548171349)) ;
#113309=CARTESIAN_POINT('Ctrl Pts',(58.4540835580999,246.894818014287,24.617578405069)) ;
#113310=CARTESIAN_POINT('Ctrl Pts',(58.4568703426308,246.84022991973,24.575427095822)) ;
#113311=CARTESIAN_POINT('Ctrl Pts',(58.4596573049167,246.785638343269,24.5332730979523)) ;
#113312=CARTESIAN_POINT('Ctrl Pts',(58.4624442672027,246.733276968376,24.4882441407519)) ;
#113313=CARTESIAN_POINT('Ctrl Pts',(58.4652312294887,246.683452629847,24.4406131779352)) ;
#113314=CARTESIAN_POINT('Ctrl Pts',(58.4680211464405,246.633575468835,24.3929317179949)) ;
#113315=CARTESIAN_POINT('Ctrl Pts',(58.4708110633923,246.586241067216,24.3426430869953)) ;
#113316=CARTESIAN_POINT('Ctrl Pts',(58.4736009803441,246.541719445691,24.2900571754578)) ;
#113317=CARTESIAN_POINT('Ctrl Pts',(58.476392570498,246.49717112313,24.237439726474)) ;
#113318=CARTESIAN_POINT('Ctrl Pts',(58.4791841606519,246.455439234969,24.1825226455728)) ;
#113319=CARTESIAN_POINT('Ctrl Pts',(58.4819757508057,246.416751811975,24.1256467574084)) ;
#113320=CARTESIAN_POINT('Ctrl Pts',(58.4847721065347,246.377998344967,24.0686737753646)) ;
#113321=CARTESIAN_POINT('Ctrl Pts',(58.4875684622637,246.342299969793,24.0097357317403)) ;
#113322=CARTESIAN_POINT('Ctrl Pts',(58.4903648179927,246.309839483422,23.9491993273412)) ;
#113323=CARTESIAN_POINT('Ctrl Pts',(58.4916219552236,246.295246459535,23.9219844179492)) ;
#113324=CARTESIAN_POINT('Ctrl Pts',(58.4928790924545,246.281307191147,23.8944467528534)) ;
#113325=CARTESIAN_POINT('Ctrl Pts',(58.4941362296853,246.268035077378,23.866620863683)) ;
#113326=CARTESIAN_POINT('Ctrl Pts',(58.4969323681109,246.238515096276,23.8047302156097)) ;
#113327=CARTESIAN_POINT('Ctrl Pts',(58.4997285065364,246.21218309461,23.7411698010235)) ;
#113328=CARTESIAN_POINT('Ctrl Pts',(58.502524644962,246.189229532673,23.676300915536)) ;
#113329=CARTESIAN_POINT('Ctrl Pts',(58.5053165998703,246.166310313322,23.6115290853648)) ;
#113330=CARTESIAN_POINT('Ctrl Pts',(58.5081085547787,246.146759663823,23.5454531289407)) ;
#113331=CARTESIAN_POINT('Ctrl Pts',(58.510900509687,246.130720968833,23.4784564626628)) ;
#113332=CARTESIAN_POINT('Ctrl Pts',(58.5136892063705,246.114700991077,23.4115379818187)) ;
#113333=CARTESIAN_POINT('Ctrl Pts',(58.516477903054,246.102184941641,23.3437014003189)) ;
#113334=CARTESIAN_POINT('Ctrl Pts',(58.5192665997374,246.093266566467,23.2753457952426)) ;
#113335=CARTESIAN_POINT('Ctrl Pts',(58.522053563702,246.084353732605,23.2070326619946)) ;
#113336=CARTESIAN_POINT('Ctrl Pts',(58.5248405276666,246.07903420188,23.1382016306277)) ;
#113337=CARTESIAN_POINT('Ctrl Pts',(58.5276274916312,246.077350451562,23.0692609566347)) ;
#113338=CARTESIAN_POINT('Ctrl Pts',(58.5304136757485,246.07566717239,23.0003395735963)) ;
#113339=CARTESIAN_POINT('Ctrl Pts',(58.5331998598658,246.077617665834,22.9313090993776)) ;
#113340=CARTESIAN_POINT('Ctrl Pts',(58.5359860439832,246.083192350296,22.8625800780558)) ;
#113341=CARTESIAN_POINT('Ctrl Pts',(58.5387723999681,246.088767378637,22.7938468171395)) ;
#113342=CARTESIAN_POINT('Ctrl Pts',(58.541558755953,246.097966999588,22.725415535126)) ;
#113343=CARTESIAN_POINT('Ctrl Pts',(58.5443451119379,246.110729730287,22.657692130987)) ;
#113344=CARTESIAN_POINT('Ctrl Pts',(58.547134417857,246.123505972976,22.5898970276161)) ;
#113345=CARTESIAN_POINT('Ctrl Pts',(58.549923723776,246.139852762486,22.5228117810505)) ;
#113346=CARTESIAN_POINT('Ctrl Pts',(58.5527130296951,246.159657579804,22.4568315698038)) ;
#113347=CARTESIAN_POINT('Ctrl Pts',(58.5555040052378,246.179474251896,22.3908118641018)) ;
#113348=CARTESIAN_POINT('Ctrl Pts',(58.5582949807805,246.202752905681,22.3258989723056)) ;
#113349=CARTESIAN_POINT('Ctrl Pts',(58.5610859563231,246.229332196717,22.262469737968)) ;
#113350=CARTESIAN_POINT('Ctrl Pts',(58.5638816983426,246.25595688033,22.1989321780755)) ;
#113351=CARTESIAN_POINT('Ctrl Pts',(58.5666774403621,246.285893238002,22.1368837744407)) ;
#113352=CARTESIAN_POINT('Ctrl Pts',(58.5694731823816,246.318933572051,22.0766775570614)) ;
#113353=CARTESIAN_POINT('Ctrl Pts',(58.5707356801446,246.333853885705,22.0494897070255)) ;
#113354=CARTESIAN_POINT('Ctrl Pts',(58.5719981779077,246.349406580268,22.0226771347491)) ;
#113355=CARTESIAN_POINT('Ctrl Pts',(58.5732606756708,246.365569721326,21.9962702898693)) ;
#113356=CARTESIAN_POINT('Ctrl Pts',(58.5760570346494,246.401370136934,21.9377806672056)) ;
#113357=CARTESIAN_POINT('Ctrl Pts',(58.578853393628,246.440308605341,21.8810541206144)) ;
#113358=CARTESIAN_POINT('Ctrl Pts',(58.5816497526066,246.482185959513,21.8264472884962)) ;
#113359=CARTESIAN_POINT('Ctrl Pts',(58.5844419309789,246.524000706297,21.7719220945611)) ;
#113360=CARTESIAN_POINT('Ctrl Pts',(58.5872341093512,246.568745322163,21.7195107118026)) ;
#113361=CARTESIAN_POINT('Ctrl Pts',(58.5900262877235,246.61617643857,21.669542361711)) ;
#113362=CARTESIAN_POINT('Ctrl Pts',(58.5928152110515,246.663552261093,21.6196322633398)) ;
#113363=CARTESIAN_POINT('Ctrl Pts',(58.5956041343795,246.713608027649,21.5721598954964)) ;
#113364=CARTESIAN_POINT('Ctrl Pts',(58.5983930577075,246.766060187121,21.5274213944491)) ;
#113365=CARTESIAN_POINT('Ctrl Pts',(58.6011802501525,246.818479793332,21.4827106593532)) ;
#113366=CARTESIAN_POINT('Ctrl Pts',(58.6039674425975,246.873292469407,21.4407307429236)) ;
#113367=CARTESIAN_POINT('Ctrl Pts',(58.6067546350425,246.930179027894,21.4017397974827)) ;
#113368=CARTESIAN_POINT('Ctrl Pts',(58.6095410491183,246.987049699876,21.362759740903)) ;
#113369=CARTESIAN_POINT('Ctrl Pts',(58.6123274631941,247.045992699782,21.3267672754933)) ;
#113370=CARTESIAN_POINT('Ctrl Pts',(58.6151138772699,247.106658548957,21.2939781529931)) ;
#113371=CARTESIAN_POINT('Ctrl Pts',(58.6179004643351,247.16732816446,21.2611869948399)) ;
#113372=CARTESIAN_POINT('Ctrl Pts',(58.6206870514004,247.229720408583,21.2315998055393)) ;
#113373=CARTESIAN_POINT('Ctrl Pts',(58.6234736384656,247.293461409716,21.2053862900903)) ;
#113374=CARTESIAN_POINT('Ctrl Pts',(58.6262631755665,247.357269890609,21.1791450235597)) ;
#113375=CARTESIAN_POINT('Ctrl Pts',(58.6290527126674,247.422429523254,21.1562847454821)) ;
#113376=CARTESIAN_POINT('Ctrl Pts',(58.6318422497683,247.488547607392,21.1369265286263)) ;
#113377=CARTESIAN_POINT('Ctrl Pts',(58.6346334568804,247.554705274421,21.1175567225933)) ;
#113378=CARTESIAN_POINT('Ctrl Pts',(58.6374246639925,247.621822057238,21.1016932634121)) ;
#113379=CARTESIAN_POINT('Ctrl Pts',(58.6402158711046,247.689494014506,21.0894062952337)) ;
#113380=CARTESIAN_POINT('Ctrl Pts',(58.6430118428712,247.757281489355,21.0770983529192)) ;
#113381=CARTESIAN_POINT('Ctrl Pts',(58.6458078146379,247.825625543487,21.0683791482484)) ;
#113382=CARTESIAN_POINT('Ctrl Pts',(58.6486037864045,247.894116934739,21.0632669833278)) ;
#113383=CARTESIAN_POINT('Ctrl Pts',(58.6498642314884,247.924993368625,21.0609623809639)) ;
#113384=CARTESIAN_POINT('Ctrl Pts',(58.6511246765724,247.955899747104,21.0593901220406)) ;
#113385=CARTESIAN_POINT('Ctrl Pts',(58.6523851216563,247.986798772013,21.0585484258527)) ;
#113386=CARTESIAN_POINT('Ctrl Pts',(58.6551814899633,248.055349996556,21.0566810755222)) ;
#113387=CARTESIAN_POINT('Ctrl Pts',(58.6579778582703,248.124133566806,21.0584056752107)) ;
#113388=CARTESIAN_POINT('Ctrl Pts',(58.6607742265772,248.192741916983,21.0637496366228)) ;
#113389=CARTESIAN_POINT('Ctrl Pts',(58.6635664151064,248.261247717128,21.0690856103277)) ;
#113390=CARTESIAN_POINT('Ctrl Pts',(58.6663586036356,248.329578331552,21.0780301706077)) ;
#113391=CARTESIAN_POINT('Ctrl Pts',(58.6691507921648,248.397325088048,21.0905587268665)) ;
#113392=CARTESIAN_POINT('Ctrl Pts',(58.6719397268291,248.464992896152,21.1030726830261)) ;
#113393=CARTESIAN_POINT('Ctrl Pts',(58.6747286614933,248.532077717279,21.1191622511777)) ;
#113394=CARTESIAN_POINT('Ctrl Pts',(58.6775175961576,248.598176715433,21.1387511182579)) ;
#113395=CARTESIAN_POINT('Ctrl Pts',(58.6803048006659,248.664234708116,21.1583278331008)) ;
#113396=CARTESIAN_POINT('Ctrl Pts',(58.6830920051742,248.72930762151,21.1813994011998)) ;
#113397=CARTESIAN_POINT('Ctrl Pts',(58.6858792096824,248.793005041016,21.2078389284572)) ;
#113398=CARTESIAN_POINT('Ctrl Pts',(58.688665636531,248.856684688264,21.2342710788057)) ;
#113399=CARTESIAN_POINT('Ctrl Pts',(58.6914520633797,248.918989150438,21.264069134643)) ;
#113400=CARTESIAN_POINT('Ctrl Pts',(58.6942384902283,248.979547050605,21.2970576948037)) ;
#113401=CARTESIAN_POINT('Ctrl Pts',(58.6970250907593,249.04010872544,21.3300483111932)) ;
#113402=CARTESIAN_POINT('Ctrl Pts',(58.6998116912902,249.098923192355,21.3662295896848)) ;
#113403=CARTESIAN_POINT('Ctrl Pts',(58.7025982918212,249.155644383876,21.4053805796855)) ;
#113404=CARTESIAN_POINT('Ctrl Pts',(58.7053878433467,249.212425642824,21.4445730303674)) ;
#113405=CARTESIAN_POINT('Ctrl Pts',(58.7081773948722,249.267108797801,21.4867411893515)) ;
#113406=CARTESIAN_POINT('Ctrl Pts',(58.7109669463977,249.319378291217,21.5316218123213)) ;
#113407=CARTESIAN_POINT('Ctrl Pts',(58.7137581685039,249.371679087302,21.5765293129827)) ;
#113408=CARTESIAN_POINT('Ctrl Pts',(58.7165493906102,249.42156298993,21.6241521716751)) ;
#113409=CARTESIAN_POINT('Ctrl Pts',(58.7193406127164,249.468751012494,21.6741899600959)) ;
#113410=CARTESIAN_POINT('Ctrl Pts',(58.7221366001999,249.516019597879,21.7243131766656)) ;
#113411=CARTESIAN_POINT('Ctrl Pts',(58.7249325876834,249.560582800146,21.7768591773811)) ;
#113412=CARTESIAN_POINT('Ctrl Pts',(58.7277285751669,249.602202207231,21.831494832244)) ;
#113413=CARTESIAN_POINT('Ctrl Pts',(58.7289889059919,249.620962742454,21.8561226248836)) ;
#113414=CARTESIAN_POINT('Ctrl Pts',(58.7302492368168,249.639125725635,21.8811746274393)) ;
#113415=CARTESIAN_POINT('Ctrl Pts',(58.7315095676418,249.65667232475,21.9066186081401)) ;
#113416=CARTESIAN_POINT('Ctrl Pts',(58.734341194748,249.696094851511,21.9637844442945)) ;
#113417=CARTESIAN_POINT('Ctrl Pts',(58.7371728218541,249.73255539459,22.0231515764158)) ;
#113418=CARTESIAN_POINT('Ctrl Pts',(58.7400044489602,249.765804160563,22.0843853258864)) ;
#113419=CARTESIAN_POINT('Ctrl Pts',(58.7428315631313,249.798999935969,22.1455214834324)) ;
#113420=CARTESIAN_POINT('Ctrl Pts',(58.7456586773023,249.828993872798,22.2085179383267)) ;
#113421=CARTESIAN_POINT('Ctrl Pts',(58.7484857914733,249.855579119968,22.273010723698)) ;
#113422=CARTESIAN_POINT('Ctrl Pts',(58.7513087092328,249.882124905471,22.3374077795556)) ;
#113423=CARTESIAN_POINT('Ctrl Pts',(58.7541316269924,249.905271880031,22.4032963141276)) ;
#113424=CARTESIAN_POINT('Ctrl Pts',(58.7569545447519,249.924859700972,22.4702890655611)) ;
#113425=CARTESIAN_POINT('Ctrl Pts',(58.7597749878247,249.944430350418,22.5372230883702)) ;
#113426=CARTESIAN_POINT('Ctrl Pts',(58.7625954308975,249.96044790909,22.6052589520035)) ;
#113427=CARTESIAN_POINT('Ctrl Pts',(58.7654158739702,249.972801063341,22.6739919247885)) ;
#113428=CARTESIAN_POINT('Ctrl Pts',(58.7682349199379,249.985148098463,22.742690850728)) ;
#113429=CARTESIAN_POINT('Ctrl Pts',(58.7710539659055,249.99383424755,22.8120857340777)) ;
#113430=CARTESIAN_POINT('Ctrl Pts',(58.7738730118731,249.998799091685,22.8817607365289)) ;
#113431=CARTESIAN_POINT('Ctrl Pts',(58.7757661168877,250.002133188196,22.9285503589917)) ;
#113432=CARTESIAN_POINT('Ctrl Pts',(58.7776592219022,250.003790153872,22.9754660703664)) ;
#113433=CARTESIAN_POINT('Ctrl Pts',(58.7795523269168,250.003764821542,23.0223805706392)) ;
#113434=CARTESIAN_POINT('',(59.2795523268825,250.003764929479,23.0221571305627)) ;
#113435=CARTESIAN_POINT('Ctrl Pts',(58.7795523269483,250.003764821541,23.0223805714202)) ;
#113436=CARTESIAN_POINT('Ctrl Pts',(58.7826465261243,250.0037234169,23.0990603155281)) ;
#113437=CARTESIAN_POINT('Ctrl Pts',(58.7857407253004,249.999186060935,23.1755820244515)) ;
#113438=CARTESIAN_POINT('Ctrl Pts',(58.7888349244764,249.990232745583,23.2514473987812)) ;
#113439=CARTESIAN_POINT('Ctrl Pts',(58.7919411809528,249.981244541458,23.3276084010112)) ;
#113440=CARTESIAN_POINT('Ctrl Pts',(58.7950474374292,249.967806032364,23.4031076705707)) ;
#113441=CARTESIAN_POINT('Ctrl Pts',(58.7981536939056,249.950047983388,23.4774580618604)) ;
#113442=CARTESIAN_POINT('Ctrl Pts',(58.8012752838319,249.932202275149,23.5521754698508)) ;
#113443=CARTESIAN_POINT('Ctrl Pts',(58.8043968737583,249.909994416863,23.6257323648907)) ;
#113444=CARTESIAN_POINT('Ctrl Pts',(58.8075184636846,249.883605268359,23.6976555433071)) ;
#113445=CARTESIAN_POINT('Ctrl Pts',(58.8085569803322,249.8748259057,23.721583547912)) ;
#113446=CARTESIAN_POINT('Ctrl Pts',(58.8095954969798,249.865584135377,23.7453309205817)) ;
#113447=CARTESIAN_POINT('Ctrl Pts',(58.8106340136274,249.855887747668,23.7688808291055)) ;
#113448=CARTESIAN_POINT('Ctrl Pts',(58.8134303540687,249.829778969199,23.8322920047936)) ;
#113449=CARTESIAN_POINT('Ctrl Pts',(58.8162266945101,249.800293020772,23.8944581076853)) ;
#113450=CARTESIAN_POINT('Ctrl Pts',(58.8190230349514,249.767570213188,23.9549955134402)) ;
#113451=CARTESIAN_POINT('Ctrl Pts',(58.8218151949193,249.734896325552,24.0154424169766)) ;
#113452=CARTESIAN_POINT('Ctrl Pts',(58.8246073548873,249.698995414582,24.0742650276122)) ;
#113453=CARTESIAN_POINT('Ctrl Pts',(58.8273995148552,249.660055769466,24.1310998091892)) ;
#113454=CARTESIAN_POINT('Ctrl Pts',(58.8301884200708,249.621161515339,24.1878683398563)) ;
#113455=CARTESIAN_POINT('Ctrl Pts',(58.8329773252864,249.579235838321,24.2426532405667)) ;
#113456=CARTESIAN_POINT('Ctrl Pts',(58.835766230502,249.534511933172,24.29511729552)) ;
#113457=CARTESIAN_POINT('Ctrl Pts',(58.8385534050279,249.489815781997,24.3475487932539)) ;
#113458=CARTESIAN_POINT('Ctrl Pts',(58.8413405795538,249.442325165229,24.3976619296572)) ;
#113459=CARTESIAN_POINT('Ctrl Pts',(58.8441277540797,249.39231446803,24.4451513649466)) ;
#113460=CARTESIAN_POINT('Ctrl Pts',(58.8469141504586,249.342317733242,24.4926275417321)) ;
#113461=CARTESIAN_POINT('Ctrl Pts',(58.8497005468374,249.289802670604,24.5374811338375)) ;
#113462=CARTESIAN_POINT('Ctrl Pts',(58.8524869432162,249.235080275476,24.5794438832885)) ;
#113463=CARTESIAN_POINT('Ctrl Pts',(58.8552735128358,249.180354478052,24.6214092417208)) ;
#113464=CARTESIAN_POINT('Ctrl Pts',(58.8580600824553,249.123421466723,24.660483104034)) ;
#113465=CARTESIAN_POINT('Ctrl Pts',(58.8608466520749,249.064623598917,24.6964388264282)) ;
#113466=CARTESIAN_POINT('Ctrl Pts',(58.8636361722326,249.005763473434,24.7324326202669)) ;
#113467=CARTESIAN_POINT('Ctrl Pts',(58.8664256923903,248.945034970413,24.7653014287764)) ;
#113468=CARTESIAN_POINT('Ctrl Pts',(58.869215212548,248.88280672345,24.7948636545263)) ;
#113469=CARTESIAN_POINT('Ctrl Pts',(58.8720064029805,248.820541216217,24.8244435811847)) ;
#113470=CARTESIAN_POINT('Ctrl Pts',(58.874797593413,248.756774631668,24.8507127976591)) ;
#113471=CARTESIAN_POINT('Ctrl Pts',(58.8775887838455,248.69189474994,24.8735382193687)) ;
#113472=CARTESIAN_POINT('Ctrl Pts',(58.8803847395139,248.626904102592,24.8964026095829)) ;
#113473=CARTESIAN_POINT('Ctrl Pts',(58.8831806951822,248.560796835394,24.9158113328648)) ;
#113474=CARTESIAN_POINT('Ctrl Pts',(58.8859766508506,248.493974153722,24.9316816579805)) ;
#113475=CARTESIAN_POINT('Ctrl Pts',(58.8872372537713,248.463846040947,24.9388370569093)) ;
#113476=CARTESIAN_POINT('Ctrl Pts',(58.8884978566921,248.433572608176,24.9452738653903)) ;
#113477=CARTESIAN_POINT('Ctrl Pts',(58.8897584596129,248.403190980567,24.9509879472846)) ;
#113478=CARTESIAN_POINT('Ctrl Pts',(58.8925547989444,248.335796768767,24.9636632407346)) ;
#113479=CARTESIAN_POINT('Ctrl Pts',(58.8953511382759,248.267605562946,24.9728285101274)) ;
#113480=CARTESIAN_POINT('Ctrl Pts',(58.8981474776075,248.199015467649,24.9783922822586)) ;
#113481=CARTESIAN_POINT('Ctrl Pts',(58.9009396365133,248.130527912052,24.9839477367528)) ;
#113482=CARTESIAN_POINT('Ctrl Pts',(58.9037317954192,248.061643135884,24.9859123407114)) ;
#113483=CARTESIAN_POINT('Ctrl Pts',(58.9065239543251,247.992768554336,24.9842457948721)) ;
#113484=CARTESIAN_POINT('Ctrl Pts',(58.9093128585551,247.923974256343,24.9825811916395)) ;
#113485=CARTESIAN_POINT('Ctrl Pts',(58.9121017627851,247.855190617769,24.9772938568925)) ;
#113486=CARTESIAN_POINT('Ctrl Pts',(58.9148906670151,247.78682746458,24.9683954861789)) ;
#113487=CARTESIAN_POINT('Ctrl Pts',(58.9176778406036,247.718506733826,24.9595026373076)) ;
#113488=CARTESIAN_POINT('Ctrl Pts',(58.9204650141921,247.650606456473,24.9470032610063)) ;
#113489=CARTESIAN_POINT('Ctrl Pts',(58.9232521877806,247.5835321864,24.9309609611948)) ;
#113490=CARTESIAN_POINT('Ctrl Pts',(58.9260385832719,247.516476641499,24.9149231399236)) ;
#113491=CARTESIAN_POINT('Ctrl Pts',(58.9288249787631,247.450247123213,24.895344472897)) ;
#113492=CARTESIAN_POINT('Ctrl Pts',(58.9316113742544,247.385238052294,24.8723394700339)) ;
#113493=CARTESIAN_POINT('Ctrl Pts',(58.9343979430379,247.320224938315,24.849333036438)) ;
#113494=CARTESIAN_POINT('Ctrl Pts',(58.9371845118213,247.256432884241,24.822900010107)) ;
#113495=CARTESIAN_POINT('Ctrl Pts',(58.9399710806048,247.194238517168,24.7932038775334)) ;
#113496=CARTESIAN_POINT('Ctrl Pts',(58.9427606000104,247.131978294167,24.7634763005301)) ;
#113497=CARTESIAN_POINT('Ctrl Pts',(58.945550119416,247.071319578055,24.7304789337767)) ;
#113498=CARTESIAN_POINT('Ctrl Pts',(58.9483396388216,247.012615552558,24.6944218472468)) ;
#113499=CARTESIAN_POINT('Ctrl Pts',(58.951130828549,246.953876375983,24.6583431702813)) ;
#113500=CARTESIAN_POINT('Ctrl Pts',(58.9539220182765,246.897094623642,24.6192014057697)) ;
#113501=CARTESIAN_POINT('Ctrl Pts',(58.9567132080039,246.842593243395,24.577249119322)) ;
#113502=CARTESIAN_POINT('Ctrl Pts',(58.9595091630472,246.787998814549,24.535225208974)) ;
#113503=CARTESIAN_POINT('Ctrl Pts',(58.9623051180904,246.735692900195,24.4903815195425)) ;
#113504=CARTESIAN_POINT('Ctrl Pts',(58.9651010731337,246.685963550708,24.4430093188615)) ;
#113505=CARTESIAN_POINT('Ctrl Pts',(58.9663616839553,246.663542104317,24.4216506389487)) ;
#113506=CARTESIAN_POINT('Ctrl Pts',(58.9676222947768,246.641643905704,24.3997784272724)) ;
#113507=CARTESIAN_POINT('Ctrl Pts',(58.9688829055984,246.620292659259,24.3774215549088)) ;
#113508=CARTESIAN_POINT('Ctrl Pts',(58.9716792401988,246.572930516895,24.3278286951007)) ;
#113509=CARTESIAN_POINT('Ctrl Pts',(58.9744755747991,246.528076671213,24.2756543986102)) ;
#113510=CARTESIAN_POINT('Ctrl Pts',(58.9772719093995,246.486024812183,24.2211825662849)) ;
#113511=CARTESIAN_POINT('Ctrl Pts',(58.9800640634739,246.444035820768,24.1667921694607)) ;
#113512=CARTESIAN_POINT('Ctrl Pts',(58.9828562175483,246.404840799509,24.1101114395027)) ;
#113513=CARTESIAN_POINT('Ctrl Pts',(58.9856483716227,246.368695610334,24.0514599773901)) ;
#113514=CARTESIAN_POINT('Ctrl Pts',(58.9884372708968,246.332592555428,23.9928768849977)) ;
#113515=CARTESIAN_POINT('Ctrl Pts',(58.991226170171,246.299532527978,23.9323280389777)) ;
#113516=CARTESIAN_POINT('Ctrl Pts',(58.9940150694451,246.269729112615,23.8701634031445)) ;
#113517=CARTESIAN_POINT('Ctrl Pts',(58.9968022380036,246.239944192449,23.8080373450087)) ;
#113518=CARTESIAN_POINT('Ctrl Pts',(58.999589406562,246.213412086901,23.7442979278645)) ;
#113519=CARTESIAN_POINT('Ctrl Pts',(59.0023765751204,246.190300533026,23.6793198284634)) ;
#113520=CARTESIAN_POINT('Ctrl Pts',(59.0051629655152,246.167195431783,23.6143598706264)) ;
#113521=CARTESIAN_POINT('Ctrl Pts',(59.0079493559099,246.147509150645,23.5481623793557)) ;
#113522=CARTESIAN_POINT('Ctrl Pts',(59.0107357463047,246.131360679587,23.4811204457802)) ;
#113523=CARTESIAN_POINT('Ctrl Pts',(59.0135223099329,246.115211204558,23.4140743441216)) ;
#113524=CARTESIAN_POINT('Ctrl Pts',(59.0163088735611,246.102600088724,23.3461841737032)) ;
#113525=CARTESIAN_POINT('Ctrl Pts',(59.0190954371893,246.093595562003,23.2778548042511)) ;
#113526=CARTESIAN_POINT('Ctrl Pts',(59.0218849513863,246.084581500788,23.2094530838579)) ;
#113527=CARTESIAN_POINT('Ctrl Pts',(59.0246744655832,246.079181714025,23.1406117238914)) ;
#113528=CARTESIAN_POINT('Ctrl Pts',(59.0274639797802,246.077412598308,23.0717413315915)) ;
#113529=CARTESIAN_POINT('Ctrl Pts',(59.030255164261,246.075642423292,23.0028297016082)) ;
#113530=CARTESIAN_POINT('Ctrl Pts',(59.0330463487418,246.077507232746,22.9338894953879)) ;
#113531=CARTESIAN_POINT('Ctrl Pts',(59.0358375332225,246.082971314618,22.8653291347449)) ;
#113532=CARTESIAN_POINT('Ctrl Pts',(59.0386334830153,246.088444725166,22.796651722896)) ;
#113533=CARTESIAN_POINT('Ctrl Pts',(59.0414294328081,246.097529607418,22.7283559371215)) ;
#113534=CARTESIAN_POINT('Ctrl Pts',(59.0442253826009,246.110138780026,22.6608420378504)) ;
#113535=CARTESIAN_POINT('Ctrl Pts',(59.0454860389286,246.115824087135,22.630400924587)) ;
#113536=CARTESIAN_POINT('Ctrl Pts',(59.0467466952562,246.12222519591,22.6001185853171)) ;
#113537=CARTESIAN_POINT('Ctrl Pts',(59.0480073515839,246.129330820986,22.5700306344666)) ;
#113538=CARTESIAN_POINT('Ctrl Pts',(59.05080368882,246.145092233156,22.503290750269)) ;
#113539=CARTESIAN_POINT('Ctrl Pts',(59.0536000260561,246.164385113101,22.4372466801164)) ;
#113540=CARTESIAN_POINT('Ctrl Pts',(59.0563963632922,246.187131528414,22.3722993985944)) ;
#113541=CARTESIAN_POINT('Ctrl Pts',(59.0591885200428,246.209843938151,22.3074492123594)) ;
#113542=CARTESIAN_POINT('Ctrl Pts',(59.0619806767934,246.235999475072,22.2436930199692)) ;
#113543=CARTESIAN_POINT('Ctrl Pts',(59.064772833544,246.265469657009,22.1814195411433)) ;
#113544=CARTESIAN_POINT('Ctrl Pts',(59.0675617355409,246.294905486223,22.1192186530988)) ;
#113545=CARTESIAN_POINT('Ctrl Pts',(59.0703506375377,246.32764807756,22.0584974874983)) ;
#113546=CARTESIAN_POINT('Ctrl Pts',(59.0731395395346,246.363520448566,21.9996258697678)) ;
#113547=CARTESIAN_POINT('Ctrl Pts',(59.0759267108429,246.399370558517,21.9407907855667)) ;
#113548=CARTESIAN_POINT('Ctrl Pts',(59.0787138821512,246.438346340316,21.8838033905302)) ;
#113549=CARTESIAN_POINT('Ctrl Pts',(59.0815010534596,246.480225101903,21.8290085428787)) ;
#113550=CARTESIAN_POINT('Ctrl Pts',(59.0842874466271,246.522092171501,21.7742289932125)) ;
#113551=CARTESIAN_POINT('Ctrl Pts',(59.0870738397947,246.566860313932,21.721641165454)) ;
#113552=CARTESIAN_POINT('Ctrl Pts',(59.0898602329622,246.614264827651,21.671559086502)) ;
#113553=CARTESIAN_POINT('Ctrl Pts',(59.0926467993818,246.661672288883,21.6214738935511)) ;
#113554=CARTESIAN_POINT('Ctrl Pts',(59.0954333658015,246.711716107579,21.5738951134208)) ;
#113555=CARTESIAN_POINT('Ctrl Pts',(59.0982199322211,246.76409403878,21.5291006370043)) ;
#113556=CARTESIAN_POINT('Ctrl Pts',(59.1010094492184,246.816527430763,21.4842587296061)) ;
#113557=CARTESIAN_POINT('Ctrl Pts',(59.1037989662157,246.871299493763,21.4422073290616)) ;
#113558=CARTESIAN_POINT('Ctrl Pts',(59.106588483213,246.928074919113,21.4031839975677)) ;
#113559=CARTESIAN_POINT('Ctrl Pts',(59.1093796705032,246.984884340167,21.3641372998798)) ;
#113560=CARTESIAN_POINT('Ctrl Pts',(59.1121708577934,247.043699092379,21.3281225361713)) ;
#113561=CARTESIAN_POINT('Ctrl Pts',(59.1149620450837,247.10415729574,21.2953323904655)) ;
#113562=CARTESIAN_POINT('Ctrl Pts',(59.1177579976706,247.164718717282,21.262486263288)) ;
#113563=CARTESIAN_POINT('Ctrl Pts',(59.1205539502575,247.226928746853,21.2328759522659)) ;
#113564=CARTESIAN_POINT('Ctrl Pts',(59.1233499028444,247.290404291723,21.2066465418713)) ;
#113565=CARTESIAN_POINT('Ctrl Pts',(59.1246105344194,247.319023974504,21.1948202959282)) ;
#113566=CARTESIAN_POINT('Ctrl Pts',(59.1258711659944,247.347900705571,21.183680683096)) ;
#113567=CARTESIAN_POINT('Ctrl Pts',(59.1271317975694,247.376998477152,21.1732376542062)) ;
#113568=CARTESIAN_POINT('Ctrl Pts',(59.1299281344919,247.441543245541,21.1500728946957)) ;
#113569=CARTESIAN_POINT('Ctrl Pts',(59.1327244714143,247.507429602488,21.1302481286355)) ;
#113570=CARTESIAN_POINT('Ctrl Pts',(59.1355208083368,247.574278898709,21.1139165837462)) ;
#113571=CARTESIAN_POINT('Ctrl Pts',(59.1383129647749,247.641028256174,21.0976094542866)) ;
#113572=CARTESIAN_POINT('Ctrl Pts',(59.141105121213,247.708737222676,21.0847852965806)) ;
#113573=CARTESIAN_POINT('Ctrl Pts',(59.1438972776511,247.777009869317,21.0755482784352)) ;
#113574=CARTESIAN_POINT('Ctrl Pts',(59.1466861793387,247.845202932154,21.0663220276625)) ;
#113575=CARTESIAN_POINT('Ctrl Pts',(59.1494750810264,247.913957885993,21.0606746771762)) ;
#113576=CARTESIAN_POINT('Ctrl Pts',(59.152263982714,247.982868205832,21.0586594340681)) ;
#113577=CARTESIAN_POINT('Ctrl Pts',(59.1550511537154,248.051735762549,21.0566454415432)) ;
#113578=CARTESIAN_POINT('Ctrl Pts',(59.1578383247167,248.120758004461,21.0582590993305)) ;
#113579=CARTESIAN_POINT('Ctrl Pts',(59.1606254957181,248.189524423037,21.0635016832106)) ;
#113580=CARTESIAN_POINT('Ctrl Pts',(59.1634118885814,248.258271643017,21.0687428034366)) ;
#113581=CARTESIAN_POINT('Ctrl Pts',(59.1661982814448,248.326762692275,21.0776108010526)) ;
#113582=CARTESIAN_POINT('Ctrl Pts',(59.1689846743081,248.39459001199,21.0900549262074)) ;
#113583=CARTESIAN_POINT('Ctrl Pts',(59.1717712404267,248.462421549146,21.1024998251265)) ;
#113584=CARTESIAN_POINT('Ctrl Pts',(59.1745578065454,248.529588792526,21.1185212019465)) ;
#113585=CARTESIAN_POINT('Ctrl Pts',(59.177344372664,248.595694014761,21.1380171339577)) ;
#113586=CARTESIAN_POINT('Ctrl Pts',(59.1801338893674,248.6618692332,21.1575337094402)) ;
#113587=CARTESIAN_POINT('Ctrl Pts',(59.1829234060707,248.726979714662,21.1805320431338)) ;
#113588=CARTESIAN_POINT('Ctrl Pts',(59.185712922774,248.790643520116,21.2068605098048)) ;
#113589=CARTESIAN_POINT('Ctrl Pts',(59.1885041097738,248.854345445948,21.2332047413381)) ;
#113590=CARTESIAN_POINT('Ctrl Pts',(59.1912952967737,248.916598528649,21.2628828631803)) ;
#113591=CARTESIAN_POINT('Ctrl Pts',(59.1940864837735,248.97704397061,21.2956965108062)) ;
#113592=CARTESIAN_POINT('Ctrl Pts',(59.1968824360786,249.037592609161,21.3285661801345)) ;
#113593=CARTESIAN_POINT('Ctrl Pts',(59.1996783883837,249.09632702957,21.3645818026303)) ;
#113594=CARTESIAN_POINT('Ctrl Pts',(59.2024743406888,249.152916778104,21.4035012836708)) ;
#113595=CARTESIAN_POINT('Ctrl Pts',(59.2037349749775,249.178431869066,21.4210492340455)) ;
#113596=CARTESIAN_POINT('Ctrl Pts',(59.2049956092663,249.203511410583,21.4391869641449)) ;
#113597=CARTESIAN_POINT('Ctrl Pts',(59.206256243555,249.228127432623,21.4578897095905)) ;
#113598=CARTESIAN_POINT('Ctrl Pts',(59.2090240914643,249.282174356261,21.4989534465851)) ;
#113599=CARTESIAN_POINT('Ctrl Pts',(59.2117919393736,249.334206058704,21.5429118444611)) ;
#113600=CARTESIAN_POINT('Ctrl Pts',(59.2145597872828,249.38389135594,21.5895379734799)) ;
#113601=CARTESIAN_POINT('Ctrl Pts',(59.2173229304128,249.433492198262,21.6360848475491)) ;
#113602=CARTESIAN_POINT('Ctrl Pts',(59.2200860735428,249.480754191283,21.68529010922)) ;
#113603=CARTESIAN_POINT('Ctrl Pts',(59.2228492166728,249.525377669804,21.7368854763372)) ;
#113604=CARTESIAN_POINT('Ctrl Pts',(59.2256097351383,249.569958761213,21.7884318338591)) ;
#113605=CARTESIAN_POINT('Ctrl Pts',(59.2283702536038,249.6119059787,21.8423634196678)) ;
#113606=CARTESIAN_POINT('Ctrl Pts',(59.2311307720693,249.650956196326,21.8983749008513)) ;
#113607=CARTESIAN_POINT('Ctrl Pts',(59.2338896588018,249.689983331501,21.9543532738406)) ;
#113608=CARTESIAN_POINT('Ctrl Pts',(59.2366485455343,249.726116575792,22.0124086935422)) ;
#113609=CARTESIAN_POINT('Ctrl Pts',(59.2394074322669,249.759134070949,22.072204050645)) ;
#113610=CARTESIAN_POINT('Ctrl Pts',(59.2421656779635,249.792143894389,22.1319855141116)) ;
#113611=CARTESIAN_POINT('Ctrl Pts',(59.2449239236602,249.822039163659,22.1935056729784)) ;
#113612=CARTESIAN_POINT('Ctrl Pts',(59.2476821693568,249.848643235575,22.2564015263404)) ;
#113613=CARTESIAN_POINT('Ctrl Pts',(59.2504425590596,249.875267987045,22.3193462691449)) ;
#113614=CARTESIAN_POINT('Ctrl Pts',(59.2532029487623,249.898596232054,22.3836683803723)) ;
#113615=CARTESIAN_POINT('Ctrl Pts',(59.2559633384651,249.918499395345,22.4489845932885)) ;
#113616=CARTESIAN_POINT('Ctrl Pts',(59.2587247477834,249.938409910342,22.5143249322992)) ;
#113617=CARTESIAN_POINT('Ctrl Pts',(59.2614861571016,249.95489270078,22.5806596168693)) ;
#113618=CARTESIAN_POINT('Ctrl Pts',(59.2642475664199,249.967869816684,22.6475927205034)) ;
#113619=CARTESIAN_POINT('Ctrl Pts',(59.2670136854443,249.980869065635,22.7146399815153)) ;
#113620=CARTESIAN_POINT('Ctrl Pts',(59.2697798044686,249.990350625957,22.7822872022128)) ;
#113621=CARTESIAN_POINT('Ctrl Pts',(59.272545923493,249.9962882853,22.8501316201319)) ;
#113622=CARTESIAN_POINT('Ctrl Pts',(59.2748813912895,250.001301523002,22.907413483937)) ;
#113623=CARTESIAN_POINT('Ctrl Pts',(59.277216859086,250.003789358227,22.9648356828553)) ;
#113624=CARTESIAN_POINT('Ctrl Pts',(59.2795523268825,250.003764929479,23.0221571305627)) ;
#113625=CARTESIAN_POINT('',(59.7795523268953,250.003764314891,23.0195557760669)) ;
#113626=CARTESIAN_POINT('Ctrl Pts',(59.2795523269168,250.003764929478,23.0221571314038)) ;
#113627=CARTESIAN_POINT('Ctrl Pts',(59.281495114458,250.003744608104,23.0698406809764)) ;
#113628=CARTESIAN_POINT('Ctrl Pts',(59.2834379019993,250.001987440133,23.1174851609697)) ;
#113629=CARTESIAN_POINT('Ctrl Pts',(59.2853806895405,249.998501062365,23.1650012267499)) ;
#113630=CARTESIAN_POINT('Ctrl Pts',(59.2881770263262,249.993482970476,23.2333931223291)) ;
#113631=CARTESIAN_POINT('Ctrl Pts',(59.2909733631119,249.984867830952,23.3016559393838)) ;
#113632=CARTESIAN_POINT('Ctrl Pts',(59.2937696998977,249.972669240583,23.3693814266331)) ;
#113633=CARTESIAN_POINT('Ctrl Pts',(59.2965618561942,249.960488886956,23.4370056651103)) ;
#113634=CARTESIAN_POINT('Ctrl Pts',(59.2993540124907,249.944735801524,23.5040936889007)) ;
#113635=CARTESIAN_POINT('Ctrl Pts',(59.3021461687872,249.925475432185,23.5702413604475)) ;
#113636=CARTESIAN_POINT('Ctrl Pts',(59.3049350703268,249.906237514246,23.6363119250666)) ;
#113637=CARTESIAN_POINT('Ctrl Pts',(59.3077239718664,249.883500568894,23.7014438454418)) ;
#113638=CARTESIAN_POINT('Ctrl Pts',(59.310512873406,249.857380920474,23.7652439775968)) ;
#113639=CARTESIAN_POINT('Ctrl Pts',(59.3133000442554,249.831277480952,23.8290045177253)) ;
#113640=CARTESIAN_POINT('Ctrl Pts',(59.3160872151048,249.801795688275,23.8914344559288)) ;
#113641=CARTESIAN_POINT('Ctrl Pts',(59.3188743859541,249.769100947178,23.9521580793838)) ;
#113642=CARTESIAN_POINT('Ctrl Pts',(59.3216607786618,249.736415334026,24.0128647495953)) ;
#113643=CARTESIAN_POINT('Ctrl Pts',(59.3244471713694,249.700518785888,24.0718656188556)) ;
#113644=CARTESIAN_POINT('Ctrl Pts',(59.327233564077,249.661623060812,24.1288087805911)) ;
#113645=CARTESIAN_POINT('Ctrl Pts',(59.3300201300365,249.622724917285,24.185755482929)) ;
#113646=CARTESIAN_POINT('Ctrl Pts',(59.332806695996,249.580827505552,24.2406438198851)) ;
#113647=CARTESIAN_POINT('Ctrl Pts',(59.3355932619555,249.536185365182,24.2931516348526)) ;
#113648=CARTESIAN_POINT('Ctrl Pts',(59.3383827784955,249.491495955079,24.3457150481933)) ;
#113649=CARTESIAN_POINT('Ctrl Pts',(59.3411722950355,249.444056334951,24.3958925345985)) ;
#113650=CARTESIAN_POINT('Ctrl Pts',(59.3439618115755,249.394160064921,24.4433965352748)) ;
#113651=CARTESIAN_POINT('Ctrl Pts',(59.3467529984094,249.344233918232,24.4909289801784)) ;
#113652=CARTESIAN_POINT('Ctrl Pts',(59.3495441852432,249.291848566881,24.5357844340582)) ;
#113653=CARTESIAN_POINT('Ctrl Pts',(59.3523353720771,249.237330899584,24.5777154540976)) ;
#113654=CARTESIAN_POINT('Ctrl Pts',(59.3551313242139,249.182720156039,24.6197180616105)) ;
#113655=CARTESIAN_POINT('Ctrl Pts',(59.3579272763508,249.125970235061,24.6587859926092)) ;
#113656=CARTESIAN_POINT('Ctrl Pts',(59.3607232284876,249.067436492644,24.6947154541444)) ;
#113657=CARTESIAN_POINT('Ctrl Pts',(59.3619838641671,249.041044866274,24.7109152883828)) ;
#113658=CARTESIAN_POINT('Ctrl Pts',(59.3632444998465,249.014290925836,24.7264777260704)) ;
#113659=CARTESIAN_POINT('Ctrl Pts',(59.364505135526,248.987208654823,24.7413872517713)) ;
#113660=CARTESIAN_POINT('Ctrl Pts',(59.3673014722637,248.927134875691,24.7744594986845)) ;
#113661=CARTESIAN_POINT('Ctrl Pts',(59.3700978090013,248.865208620798,24.8044456889588)) ;
#113662=CARTESIAN_POINT('Ctrl Pts',(59.372894145739,248.801779571836,24.8311346906801)) ;
#113663=CARTESIAN_POINT('Ctrl Pts',(59.3756863019872,248.738445348532,24.8577837926679)) ;
#113664=CARTESIAN_POINT('Ctrl Pts',(59.3784784582354,248.673613239039,24.8811453005798)) ;
#113665=CARTESIAN_POINT('Ctrl Pts',(59.3812706144836,248.607657739388,24.9010537958351)) ;
#113666=CARTESIAN_POINT('Ctrl Pts',(59.3840595159747,248.541779122659,24.9209390841812)) ;
#113667=CARTESIAN_POINT('Ctrl Pts',(59.3868484174658,248.474780184297,24.9373792129642)) ;
#113668=CARTESIAN_POINT('Ctrl Pts',(59.3896373189569,248.40705393545,24.9502574098997)) ;
#113669=CARTESIAN_POINT('Ctrl Pts',(59.3924244897578,248.339369715037,24.963127615097)) ;
#113670=CARTESIAN_POINT('Ctrl Pts',(59.3952116605586,248.270959560639,24.9724401819621)) ;
#113671=CARTESIAN_POINT('Ctrl Pts',(59.3979988313594,248.202228622381,24.9781289877402)) ;
#113672=CARTESIAN_POINT('Ctrl Pts',(59.4007852240185,248.133516872904,24.983816205278)) ;
#113673=CARTESIAN_POINT('Ctrl Pts',(59.4035716166776,248.064485006299,24.9858816298161)) ;
#113674=CARTESIAN_POINT('Ctrl Pts',(59.4063580093366,247.995543480419,24.9843109767633)) ;
#113675=CARTESIAN_POINT('Ctrl Pts',(59.4091445752477,247.926597667901,24.9827402260507)) ;
#113676=CARTESIAN_POINT('Ctrl Pts',(59.4119311411587,247.857742697894,24.9775329626426)) ;
#113677=CARTESIAN_POINT('Ctrl Pts',(59.4147177070697,247.789387405947,24.9687269854092)) ;
#113678=CARTESIAN_POINT('Ctrl Pts',(59.4175072235617,247.72095973537,24.9599116838858)) ;
#113679=CARTESIAN_POINT('Ctrl Pts',(59.4202967400537,247.653033286443,24.9474901268922)) ;
#113680=CARTESIAN_POINT('Ctrl Pts',(59.4230862565456,247.586009158029,24.9315516861228)) ;
#113681=CARTESIAN_POINT('Ctrl Pts',(59.4258774433317,247.51894489721,24.9156037018057)) ;
#113682=CARTESIAN_POINT('Ctrl Pts',(59.4286686301177,247.452784503118,24.8961347811677)) ;
#113683=CARTESIAN_POINT('Ctrl Pts',(59.4314598169038,247.387913609002,24.8732841045535)) ;
#113684=CARTESIAN_POINT('Ctrl Pts',(59.4342557689936,247.322931962888,24.8503944157113)) ;
#113685=CARTESIAN_POINT('Ctrl Pts',(59.4370517210834,247.259244663932,24.8241116352296)) ;
#113686=CARTESIAN_POINT('Ctrl Pts',(59.4398476731733,247.197216267198,24.7946226027313)) ;
#113687=CARTESIAN_POINT('Ctrl Pts',(59.441108309286,247.169248965032,24.7813266169264)) ;
#113688=CARTESIAN_POINT('Ctrl Pts',(59.4423689453988,247.141618552985,24.7673794386527)) ;
#113689=CARTESIAN_POINT('Ctrl Pts',(59.4436295815115,247.114356562801,24.7528011018482)) ;
#113690=CARTESIAN_POINT('Ctrl Pts',(59.4464259182225,247.053884152725,24.7204635081688)) ;
#113691=CARTESIAN_POINT('Ctrl Pts',(59.4492222549335,246.994989280571,24.6848906733036)) ;
#113692=CARTESIAN_POINT('Ctrl Pts',(59.4520185916445,246.938039561295,24.6462606792835)) ;
#113693=CARTESIAN_POINT('Ctrl Pts',(59.4548107478652,246.881174981174,24.6076884366464)) ;
#113694=CARTESIAN_POINT('Ctrl Pts',(59.457602904086,246.826250185303,24.5660683793279)) ;
#113695=CARTESIAN_POINT('Ctrl Pts',(59.4603950603067,246.773607989323,24.5216243108435)) ;
#113696=CARTESIAN_POINT('Ctrl Pts',(59.4631839617694,246.721027157251,24.4772320498805)) ;
#113697=CARTESIAN_POINT('Ctrl Pts',(59.465972863232,246.670724013783,24.4300226309442)) ;
#113698=CARTESIAN_POINT('Ctrl Pts',(59.4687617646946,246.623010682701,24.3802618965991)) ;
#113699=CARTESIAN_POINT('Ctrl Pts',(59.4715489354664,246.575326960779,24.3305320419574)) ;
#113700=CARTESIAN_POINT('Ctrl Pts',(59.4743361062381,246.530230201944,24.2782543662651)) ;
#113701=CARTESIAN_POINT('Ctrl Pts',(59.4771232770098,246.487996683113,24.2237324974251)) ;
#113702=CARTESIAN_POINT('Ctrl Pts',(59.4799096696393,246.445774955338,24.1692258503911)) ;
#113703=CARTESIAN_POINT('Ctrl Pts',(59.4826960622687,246.406415180982,24.1124766419585)) ;
#113704=CARTESIAN_POINT('Ctrl Pts',(59.4854824548981,246.370153069959,24.0538212060807)) ;
#113705=CARTESIAN_POINT('Ctrl Pts',(59.488269020779,246.333888704243,23.9951621231441)) ;
#113706=CARTESIAN_POINT('Ctrl Pts',(59.4910555866598,246.30072264016,23.934596996283)) ;
#113707=CARTESIAN_POINT('Ctrl Pts',(59.4938421525407,246.270846037523,23.8724891892)) ;
#113708=CARTESIAN_POINT('Ctrl Pts',(59.4966316690019,246.240937799777,23.8103156187065)) ;
#113709=CARTESIAN_POINT('Ctrl Pts',(59.4994211854631,246.214326187638,23.7465965512806)) ;
#113710=CARTESIAN_POINT('Ctrl Pts',(59.5022107019243,246.191154906077,23.681716975847)) ;
#113711=CARTESIAN_POINT('Ctrl Pts',(59.5050018886792,246.167969750124,23.6167985521223)) ;
#113712=CARTESIAN_POINT('Ctrl Pts',(59.5077930754341,246.148229165143,23.5507187077312)) ;
#113713=CARTESIAN_POINT('Ctrl Pts',(59.5105842621891,246.132026667399,23.4838766154112)) ;
#113714=CARTESIAN_POINT('Ctrl Pts',(59.5133802142475,246.115796507651,23.4169204057341)) ;
#113715=CARTESIAN_POINT('Ctrl Pts',(59.5161761663059,246.103116580869,23.3491998330277)) ;
#113716=CARTESIAN_POINT('Ctrl Pts',(59.5189721183643,246.09402895728,23.2811223767758)) ;
#113717=CARTESIAN_POINT('Ctrl Pts',(59.5202327547419,246.089931537638,23.2504276738445)) ;
#113718=CARTESIAN_POINT('Ctrl Pts',(59.5214933911195,246.086563699403,23.2196604587693)) ;
#113719=CARTESIAN_POINT('Ctrl Pts',(59.522754027497,246.083925833939,23.1888580873807)) ;
#113720=CARTESIAN_POINT('Ctrl Pts',(59.525550364206,246.078074535212,23.1205324358522)) ;
#113721=CARTESIAN_POINT('Ctrl Pts',(59.528346700915,246.075795493367,23.0517658849627)) ;
#113722=CARTESIAN_POINT('Ctrl Pts',(59.531143037624,246.077139788722,22.9829637059369)) ;
#113723=CARTESIAN_POINT('Ctrl Pts',(59.5339351938432,246.078482074372,22.9142643853419)) ;
#113724=CARTESIAN_POINT('Ctrl Pts',(59.5367273500625,246.083436936639,22.8455300291764)) ;
#113725=CARTESIAN_POINT('Ctrl Pts',(59.5395195062817,246.09200360609,22.7771700394243)) ;
#113726=CARTESIAN_POINT('Ctrl Pts',(59.5423084077435,246.100560289555,22.7088897354664)) ;
#113727=CARTESIAN_POINT('Ctrl Pts',(59.5450973092052,246.112720357553,22.6409834159562)) ;
#113728=CARTESIAN_POINT('Ctrl Pts',(59.547886210667,246.128431066251,22.573857666201)) ;
#113729=CARTESIAN_POINT('Ctrl Pts',(59.5506733814383,246.144132025457,22.5067735722365)) ;
#113730=CARTESIAN_POINT('Ctrl Pts',(59.5534605522096,246.163379142651,22.4404695639475)) ;
#113731=CARTESIAN_POINT('Ctrl Pts',(59.5562477229809,246.186068455924,22.3753427694719)) ;
#113732=CARTESIAN_POINT('Ctrl Pts',(59.5590341156103,246.208751434635,22.3102341575516)) ;
#113733=CARTESIAN_POINT('Ctrl Pts',(59.5618205082397,246.234874540101,22.2463025702368)) ;
#113734=CARTESIAN_POINT('Ctrl Pts',(59.5646069008691,246.264284277843,22.1839289525864)) ;
#113735=CARTESIAN_POINT('Ctrl Pts',(59.5673934667504,246.293695844219,22.12155145668)) ;
#113736=CARTESIAN_POINT('Ctrl Pts',(59.5701800326316,246.326394236939,22.0607325656101)) ;
#113737=CARTESIAN_POINT('Ctrl Pts',(59.5729665985129,246.36217901674,22.0018306079372)) ;
#113738=CARTESIAN_POINT('Ctrl Pts',(59.5757561149751,246.398001687586,21.9428662813831)) ;
#113739=CARTESIAN_POINT('Ctrl Pts',(59.5785456314373,246.436917012061,21.8858233591829)) ;
#113740=CARTESIAN_POINT('Ctrl Pts',(59.5813351478996,246.478680553845,21.8310321721944)) ;
#113741=CARTESIAN_POINT('Ctrl Pts',(59.5841263346559,246.520469102614,21.7762081775863)) ;
#113742=CARTESIAN_POINT('Ctrl Pts',(59.5869175214122,246.565108945219,21.7236389757832)) ;
#113743=CARTESIAN_POINT('Ctrl Pts',(59.5897087081685,246.612316396838,21.6736205517286)) ;
#113744=CARTESIAN_POINT('Ctrl Pts',(59.5925046602289,246.659604444231,21.6235167328156)) ;
#113745=CARTESIAN_POINT('Ctrl Pts',(59.5953006122892,246.709468494342,21.5759727215004)) ;
#113746=CARTESIAN_POINT('Ctrl Pts',(59.5980965643495,246.761589855718,21.5312458991949)) ;
#113747=CARTESIAN_POINT('Ctrl Pts',(59.5993572007272,246.785090288768,21.5110795093427)) ;
#113748=CARTESIAN_POINT('Ctrl Pts',(59.6006178371049,246.80904919775,21.4914852618308)) ;
#113749=CARTESIAN_POINT('Ctrl Pts',(59.6018784734826,246.833435477553,21.4724838468335)) ;
#113750=CARTESIAN_POINT('Ctrl Pts',(59.604674810223,246.887528990464,21.4303350116772)) ;
#113751=CARTESIAN_POINT('Ctrl Pts',(59.6074711469633,246.943939325071,21.3909407634578)) ;
#113752=CARTESIAN_POINT('Ctrl Pts',(59.6102674837036,247.002354552538,21.3545648338025)) ;
#113753=CARTESIAN_POINT('Ctrl Pts',(59.6130596399539,247.060682449938,21.318243285728)) ;
#113754=CARTESIAN_POINT('Ctrl Pts',(59.6158517962042,247.121008877979,21.2849313577405)) ;
#113755=CARTESIAN_POINT('Ctrl Pts',(59.6186439524545,247.182990182206,21.2548515632037)) ;
#113756=CARTESIAN_POINT('Ctrl Pts',(59.6214328539467,247.244899236126,21.224806832053)) ;
#113757=CARTESIAN_POINT('Ctrl Pts',(59.624221755439,247.308458895413,21.1979869647537)) ;
#113758=CARTESIAN_POINT('Ctrl Pts',(59.6270106569312,247.373299536651,21.1745693649704)) ;
#113759=CARTESIAN_POINT('Ctrl Pts',(59.6297978277326,247.438099940145,21.151166297298)) ;
#113760=CARTESIAN_POINT('Ctrl Pts',(59.632584998534,247.504179287979,21.1311614750551)) ;
#113761=CARTESIAN_POINT('Ctrl Pts',(59.6353721693355,247.571147967304,21.1146842066668)) ;
#113762=CARTESIAN_POINT('Ctrl Pts',(59.6381585619946,247.638097949833,21.0982115385202)) ;
#113763=CARTESIAN_POINT('Ctrl Pts',(59.6409449546537,247.705936294524,21.0852645862101)) ;
#113764=CARTESIAN_POINT('Ctrl Pts',(59.6437313473128,247.774259956716,21.075922309839)) ;
#113765=CARTESIAN_POINT('Ctrl Pts',(59.6465179132233,247.842587867113,21.0665794525869)) ;
#113766=CARTESIAN_POINT('Ctrl Pts',(59.6493044791337,247.911400668276,21.0608417801967)) ;
#113767=CARTESIAN_POINT('Ctrl Pts',(59.6520910450442,247.980288687947,21.0587365672425)) ;
#113768=CARTESIAN_POINT('Ctrl Pts',(59.6548805615348,248.04924965031,21.0566291251647)) ;
#113769=CARTESIAN_POINT('Ctrl Pts',(59.6576700780254,248.118285498609,21.0581618333255)) ;
#113770=CARTESIAN_POINT('Ctrl Pts',(59.660459594516,248.186986051253,21.063309818882)) ;
#113771=CARTESIAN_POINT('Ctrl Pts',(59.6632507813002,248.255727740091,21.0684608869251)) ;
#113772=CARTESIAN_POINT('Ctrl Pts',(59.6660419680844,248.324133246809,21.0772314783119)) ;
#113773=CARTESIAN_POINT('Ctrl Pts',(59.6688331548686,248.391799791067,21.0895450935756)) ;
#113774=CARTESIAN_POINT('Ctrl Pts',(59.6716291069559,248.45958186023,21.1018797314769)) ;
#113775=CARTESIAN_POINT('Ctrl Pts',(59.6744250590431,248.526621971747,21.1177693524047)) ;
#113776=CARTESIAN_POINT('Ctrl Pts',(59.6772210111303,248.592530628211,21.1370870658179)) ;
#113777=CARTESIAN_POINT('Ctrl Pts',(59.6784816472429,248.622247458071,21.1457970173412)) ;
#113778=CARTESIAN_POINT('Ctrl Pts',(59.6797422833555,248.65173452234,21.1552032118979)) ;
#113779=CARTESIAN_POINT('Ctrl Pts',(59.6810029194681,248.680957519887,21.1652908494308)) ;
#113780=CARTESIAN_POINT('Ctrl Pts',(59.6837992562552,248.745779828445,21.1876671970908)) ;
#113781=CARTESIAN_POINT('Ctrl Pts',(59.6865955930423,248.809555604496,21.2134874063395)) ;
#113782=CARTESIAN_POINT('Ctrl Pts',(59.6893919298294,248.871893712924,21.2426337176708)) ;
#113783=CARTESIAN_POINT('Ctrl Pts',(59.692184086127,248.934138626638,21.2717364556212)) ;
#113784=CARTESIAN_POINT('Ctrl Pts',(59.6949762424246,248.994949697429,21.3041552202896)) ;
#113785=CARTESIAN_POINT('Ctrl Pts',(59.6977683987222,249.053953053683,21.3397231865858)) ;
#113786=CARTESIAN_POINT('Ctrl Pts',(59.7005573002624,249.112887630976,21.3752496920575)) ;
#113787=CARTESIAN_POINT('Ctrl Pts',(59.7033462018026,249.170018260476,21.4139178560407)) ;
#113788=CARTESIAN_POINT('Ctrl Pts',(59.7061351033428,249.224994734446,21.4555144929788)) ;
#113789=CARTESIAN_POINT('Ctrl Pts',(59.7089222741924,249.279937092024,21.4970853165624)) ;
#113790=CARTESIAN_POINT('Ctrl Pts',(59.7117094450421,249.332727555446,21.5415807124321)) ;
#113791=CARTESIAN_POINT('Ctrl Pts',(59.7144966158918,249.383045343216,21.5887445203175)) ;
#113792=CARTESIAN_POINT('Ctrl Pts',(59.7172830085995,249.433349082911,21.6358951606779)) ;
#113793=CARTESIAN_POINT('Ctrl Pts',(59.7200694013071,249.48118115955,21.6857123985147)) ;
#113794=CARTESIAN_POINT('Ctrl Pts',(59.7228557940148,249.526255681274,21.7379013685143)) ;
#113795=CARTESIAN_POINT('Ctrl Pts',(59.725642359974,249.571333005628,21.7900935835056)) ;
#113796=CARTESIAN_POINT('Ctrl Pts',(59.7284289259332,249.61365211579,21.8446574502999)) ;
#113797=CARTESIAN_POINT('Ctrl Pts',(59.7312154918924,249.652966839496,21.9012643741811)) ;
#113798=CARTESIAN_POINT('Ctrl Pts',(59.7340050084317,249.692323191944,21.957931236805)) ;
#113799=CARTESIAN_POINT('Ctrl Pts',(59.7367945249709,249.72866852883,22.0166450698258)) ;
#113800=CARTESIAN_POINT('Ctrl Pts',(59.7395840415102,249.761800119688,22.0770484267928)) ;
#113801=CARTESIAN_POINT('Ctrl Pts',(59.7423752283431,249.794951548925,22.137487951799)) ;
#113802=CARTESIAN_POINT('Ctrl Pts',(59.745166415176,249.824885189213,22.1996185719547)) ;
#113803=CARTESIAN_POINT('Ctrl Pts',(59.7479576020089,249.851445627197,22.263060905038)) ;
#113804=CARTESIAN_POINT('Ctrl Pts',(59.7507535541444,249.878051410953,22.3266115511548)) ;
#113805=CARTESIAN_POINT('Ctrl Pts',(59.7535495062799,249.901272333448,22.3914779178315)) ;
#113806=CARTESIAN_POINT('Ctrl Pts',(59.7563454584154,249.921002468584,22.4572642916478)) ;
#113807=CARTESIAN_POINT('Ctrl Pts',(59.7576060940948,249.929898369196,22.4869259761237)) ;
#113808=CARTESIAN_POINT('Ctrl Pts',(59.7588667297742,249.938085311495,22.5167745401338)) ;
#113809=CARTESIAN_POINT('Ctrl Pts',(59.7601273654536,249.945557006586,22.5467731590084)) ;
#113810=CARTESIAN_POINT('Ctrl Pts',(59.7637661613916,249.967123882878,22.633363483467)) ;
#113811=CARTESIAN_POINT('Ctrl Pts',(59.7674049573295,249.982796529675,22.7214759039678)) ;
#113812=CARTESIAN_POINT('Ctrl Pts',(59.7710437532675,249.992405426665,22.8104165137978)) ;
#113813=CARTESIAN_POINT('Ctrl Pts',(59.7738799444767,249.999894901106,22.879739603097)) ;
#113814=CARTESIAN_POINT('Ctrl Pts',(59.776716135686,250.003701415725,22.9495655586124)) ;
#113815=CARTESIAN_POINT('Ctrl Pts',(59.7795523268953,250.003764314891,23.019555776067)) ;
#113816=CARTESIAN_POINT('',(60.2795523269397,250.003764993893,23.0219891156808)) ;
#113817=CARTESIAN_POINT('Ctrl Pts',(59.7795523269168,250.003764314891,23.0195557765974)) ;
#113818=CARTESIAN_POINT('Ctrl Pts',(59.7823087837182,250.003825445742,23.0875783451414)) ;
#113819=CARTESIAN_POINT('Ctrl Pts',(59.7850652405196,250.000347506381,23.1556930422578)) ;
#113820=CARTESIAN_POINT('Ctrl Pts',(59.787821697321,249.993328455219,23.2234980152068)) ;
#113821=CARTESIAN_POINT('Ctrl Pts',(59.7905763409642,249.98631402109,23.2912583870053)) ;
#113822=CARTESIAN_POINT('Ctrl Pts',(59.7933309846074,249.97576314405,23.3587089388388)) ;
#113823=CARTESIAN_POINT('Ctrl Pts',(59.7960856282505,249.961725799627,23.4254503470355)) ;
#113824=CARTESIAN_POINT('Ctrl Pts',(59.7988394545505,249.947692620291,23.4921719520753)) ;
#113825=CARTESIAN_POINT('Ctrl Pts',(59.8015932808504,249.930175129706,23.5581843383787)) ;
#113826=CARTESIAN_POINT('Ctrl Pts',(59.8043471071503,249.909274517264,23.6230977752439)) ;
#113827=CARTESIAN_POINT('Ctrl Pts',(59.8071011106438,249.888372559981,23.6880153889329)) ;
#113828=CARTESIAN_POINT('Ctrl Pts',(59.8098551141374,249.864087206595,23.7518334345976)) ;
#113829=CARTESIAN_POINT('Ctrl Pts',(59.8126091176309,249.836569075627,23.8141786569548)) ;
#113830=CARTESIAN_POINT('Ctrl Pts',(59.8153659991076,249.809022187717,23.8765890311893)) ;
#113831=CARTESIAN_POINT('Ctrl Pts',(59.8181228805843,249.778235988887,23.9375230514109)) ;
#113832=CARTESIAN_POINT('Ctrl Pts',(59.8208797620609,249.744408177207,23.9966298579936)) ;
#113833=CARTESIAN_POINT('Ctrl Pts',(59.8236383977984,249.71055884019,24.0557742754617)) ;
#113834=CARTESIAN_POINT('Ctrl Pts',(59.8263970335359,249.673664315791,24.1130887454574)) ;
#113835=CARTESIAN_POINT('Ctrl Pts',(59.8291556692733,249.633965373405,24.1682517771538)) ;
#113836=CARTESIAN_POINT('Ctrl Pts',(59.8319188058152,249.594201660896,24.2235048091405)) ;
#113837=CARTESIAN_POINT('Ctrl Pts',(59.8346819423571,249.551624723831,24.2765990144869)) ;
#113838=CARTESIAN_POINT('Ctrl Pts',(59.837445078899,249.50651445534,24.3272472560621)) ;
#113839=CARTESIAN_POINT('Ctrl Pts',(59.838047323079,249.496682369141,24.3382863807149)) ;
#113840=CARTESIAN_POINT('Ctrl Pts',(59.8386495672591,249.486730067739,24.3492094562372)) ;
#113841=CARTESIAN_POINT('Ctrl Pts',(59.8392518114391,249.476660661121,24.3600137604257)) ;
#113842=CARTESIAN_POINT('Ctrl Pts',(59.8420481483943,249.429906446177,24.4101802478372)) ;
#113843=CARTESIAN_POINT('Ctrl Pts',(59.8448444853495,249.380429270683,24.4579928233434)) ;
#113844=CARTESIAN_POINT('Ctrl Pts',(59.8476408223046,249.328495473826,24.5031417815248)) ;
#113845=CARTESIAN_POINT('Ctrl Pts',(59.850432978768,249.276639317402,24.5482232425296)) ;
#113846=CARTESIAN_POINT('Ctrl Pts',(59.8532251352314,249.222334196329,24.5906486701504)) ;
#113847=CARTESIAN_POINT('Ctrl Pts',(59.8560172916948,249.165884289625,24.6301440466038)) ;
#113848=CARTESIAN_POINT('Ctrl Pts',(59.8588061933965,249.109500185461,24.6695933840776)) ;
#113849=CARTESIAN_POINT('Ctrl Pts',(59.8615950950983,249.050976661485,24.7061191738545)) ;
#113850=CARTESIAN_POINT('Ctrl Pts',(59.8643839968001,248.990650667072,24.7394878379269)) ;
#113851=CARTESIAN_POINT('Ctrl Pts',(59.8671711678087,248.930362108825,24.7728357945933)) ;
#113852=CARTESIAN_POINT('Ctrl Pts',(59.8699583388173,248.868273727674,24.8030302751666)) ;
#113853=CARTESIAN_POINT('Ctrl Pts',(59.8727455098259,248.804749810678,24.8298820342529)) ;
#113854=CARTESIAN_POINT('Ctrl Pts',(59.8755319026895,248.741243628803,24.8567262966479)) ;
#113855=CARTESIAN_POINT('Ctrl Pts',(59.8783182955532,248.676303158655,24.8802294993315)) ;
#113856=CARTESIAN_POINT('Ctrl Pts',(59.8811046884168,248.610313905732,24.9002499904492)) ;
#113857=CARTESIAN_POINT('Ctrl Pts',(59.8838912545289,248.544320549821,24.920271726373)) ;
#113858=CARTESIAN_POINT('Ctrl Pts',(59.886677820641,248.477278752097,24.9368101807817)) ;
#113859=CARTESIAN_POINT('Ctrl Pts',(59.8894643867531,248.409588729042,24.9497736908776)) ;
#113860=CARTESIAN_POINT('Ctrl Pts',(59.8922539034395,248.34182703195,24.9627509274737)) ;
#113861=CARTESIAN_POINT('Ctrl Pts',(59.8950434201259,248.273416222728,24.9721455730314)) ;
#113862=CARTESIAN_POINT('Ctrl Pts',(59.8978329368124,248.204765260421,24.9779173766206)) ;
#113863=CARTESIAN_POINT('Ctrl Pts',(59.9006241237894,248.136073191688,24.9836926362169)) ;
#113864=CARTESIAN_POINT('Ctrl Pts',(59.9034153107664,248.067141174311,24.9858407211747)) ;
#113865=CARTESIAN_POINT('Ctrl Pts',(59.9062064977434,247.998379016395,24.9843735281035)) ;
#113866=CARTESIAN_POINT('Ctrl Pts',(59.9090024500169,247.929499463239,24.9829038301446)) ;
#113867=CARTESIAN_POINT('Ctrl Pts',(59.9117984022903,247.86079083748,24.9778065719949)) ;
#113868=CARTESIAN_POINT('Ctrl Pts',(59.9145943545638,247.792657793264,24.969145507119)) ;
#113869=CARTESIAN_POINT('Ctrl Pts',(59.9158549888508,247.761938080188,24.9652404206667)) ;
#113870=CARTESIAN_POINT('Ctrl Pts',(59.9171156231378,247.731335235253,24.960611534983)) ;
#113871=CARTESIAN_POINT('Ctrl Pts',(59.9183762574247,247.700885467052,24.9552680443662)) ;
#113872=CARTESIAN_POINT('Ctrl Pts',(59.9211725946597,247.633341833265,24.943415120857)) ;
#113873=CARTESIAN_POINT('Ctrl Pts',(59.9239689318947,247.566287434072,24.9279962372579)) ;
#113874=CARTESIAN_POINT('Ctrl Pts',(59.9267652691297,247.500127098043,24.9090658720751)) ;
#113875=CARTESIAN_POINT('Ctrl Pts',(59.9295574258795,247.434065670794,24.8901638075247)) ;
#113876=CARTESIAN_POINT('Ctrl Pts',(59.9323495826293,247.368896122028,24.8677608145071)) ;
#113877=CARTESIAN_POINT('Ctrl Pts',(59.9351417393791,247.305013986331,24.8419625484971)) ;
#113878=CARTESIAN_POINT('Ctrl Pts',(59.9379306413755,247.241206316582,24.8161943549369)) ;
#113879=CARTESIAN_POINT('Ctrl Pts',(59.9407195433719,247.17868353234,24.787038931905)) ;
#113880=CARTESIAN_POINT('Ctrl Pts',(59.9435084453682,247.117825126815,24.7546514520054)) ;
#113881=CARTESIAN_POINT('Ctrl Pts',(59.9462956166763,247.057004487741,24.7222840705649)) ;
#113882=CARTESIAN_POINT('Ctrl Pts',(59.9490827879844,246.997846610751,24.6866888412325)) ;
#113883=CARTESIAN_POINT('Ctrl Pts',(59.9518699592925,246.940708722735,24.6480680210107)) ;
#113884=CARTESIAN_POINT('Ctrl Pts',(59.95465635246,246.883586786844,24.6094579831999)) ;
#113885=CARTESIAN_POINT('Ctrl Pts',(59.9574427456276,246.828484126762,24.5678243062383)) ;
#113886=CARTESIAN_POINT('Ctrl Pts',(59.9602291387951,246.775729633658,24.5234129787429)) ;
#113887=CARTESIAN_POINT('Ctrl Pts',(59.9630157052149,246.722971860386,24.4789988898405)) ;
#113888=CARTESIAN_POINT('Ctrl Pts',(59.9658022716348,246.672562917786,24.431807125583)) ;
#113889=CARTESIAN_POINT('Ctrl Pts',(59.9685888380547,246.624797805843,24.3821232562294)) ;
#113890=CARTESIAN_POINT('Ctrl Pts',(59.9713783550525,246.576982117431,24.3323867787157)) ;
#113891=CARTESIAN_POINT('Ctrl Pts',(59.9741678720504,246.531816187178,24.280153284517)) ;
#113892=CARTESIAN_POINT('Ctrl Pts',(59.9769573890482,246.489556677735,24.2257436972719)) ;
#113893=CARTESIAN_POINT('Ctrl Pts',(59.9797485763392,246.447271864352,24.1713015309245)) ;
#113894=CARTESIAN_POINT('Ctrl Pts',(59.9825397636302,246.407897215653,24.1146810812581)) ;
#113895=CARTESIAN_POINT('Ctrl Pts',(59.9853309509212,246.371646137567,24.0562324085314)) ;
#113896=CARTESIAN_POINT('Ctrl Pts',(59.9881269035092,246.335333169275,23.997683948419)) ;
#113897=CARTESIAN_POINT('Ctrl Pts',(59.9909228560971,246.302154650851,23.9373014657754)) ;
#113898=CARTESIAN_POINT('Ctrl Pts',(59.9937188086851,246.272277703052,23.8754589662088)) ;
#113899=CARTESIAN_POINT('Ctrl Pts',(59.9949794402601,246.258806865269,23.847575586509)) ;
#113900=CARTESIAN_POINT('Ctrl Pts',(59.9962400718352,246.246006547433,23.8193956568979)) ;
#113901=CARTESIAN_POINT('Ctrl Pts',(59.9975007034102,246.233888777856,23.7909545454175)) ;
#113902=CARTESIAN_POINT('Ctrl Pts',(60.0002970378614,246.207009127045,23.7278664382821)) ;
#113903=CARTESIAN_POINT('Ctrl Pts',(60.0030933723127,246.183385777887,23.663244750275)) ;
#113904=CARTESIAN_POINT('Ctrl Pts',(60.0058897067639,246.163193722276,23.59745857671)) ;
#113905=CARTESIAN_POINT('Ctrl Pts',(60.0086818607232,246.143031853584,23.531770752814)) ;
#113906=CARTESIAN_POINT('Ctrl Pts',(60.0114740146825,246.126291240063,23.4649223641062)) ;
#113907=CARTESIAN_POINT('Ctrl Pts',(60.0142661686418,246.113098901805,23.3973026097979)) ;
#113908=CARTESIAN_POINT('Ctrl Pts',(60.0170550678515,246.099921941553,23.3297616782809)) ;
#113909=CARTESIAN_POINT('Ctrl Pts',(60.0198439670612,246.090285135311,23.2614516464973)) ;
#113910=CARTESIAN_POINT('Ctrl Pts',(60.0226328662709,246.084265245048,23.1927752559079)) ;
#113911=CARTESIAN_POINT('Ctrl Pts',(60.0254200347964,246.078249090498,23.1241414832611)) ;
#113912=CARTESIAN_POINT('Ctrl Pts',(60.0282072033219,246.075845442013,23.0551422906988)) ;
#113913=CARTESIAN_POINT('Ctrl Pts',(60.0309943718473,246.077079449864,22.9861874169946)) ;
#113914=CARTESIAN_POINT('Ctrl Pts',(60.0337807622405,246.0783131132,22.9172517943728)) ;
#113915=CARTESIAN_POINT('Ctrl Pts',(60.0365671526338,246.083182407858,22.8483609565684)) ;
#113916=CARTESIAN_POINT('Ctrl Pts',(60.039353543027,246.091660374989,22.7799247236318)) ;
#113917=CARTESIAN_POINT('Ctrl Pts',(60.0421401066851,246.100138869301,22.7114842351551)) ;
#113918=CARTESIAN_POINT('Ctrl Pts',(60.0449266703432,246.112226418696,22.6434988944507)) ;
#113919=CARTESIAN_POINT('Ctrl Pts',(60.0477132340013,246.127844406267,22.5763716831496)) ;
#113920=CARTESIAN_POINT('Ctrl Pts',(60.0505027482751,246.143478931295,22.5091733926874)) ;
#113921=CARTESIAN_POINT('Ctrl Pts',(60.053292262549,246.16265124336,22.442835523928)) ;
#113922=CARTESIAN_POINT('Ctrl Pts',(60.0560817768228,246.185232188868,22.3777481877512)) ;
#113923=CARTESIAN_POINT('Ctrl Pts',(60.0588729614075,246.20782665544,22.3126218784513)) ;
#113924=CARTESIAN_POINT('Ctrl Pts',(60.0616641459922,246.233833632505,22.2487480466602)) ;
#113925=CARTESIAN_POINT('Ctrl Pts',(60.0644553305769,246.263075960335,22.1864964195009)) ;
#113926=CARTESIAN_POINT('Ctrl Pts',(60.0672512805139,246.2923682132,22.1241385109683)) ;
#113927=CARTESIAN_POINT('Ctrl Pts',(60.0700472304508,246.324906609224,22.0634087668915)) ;
#113928=CARTESIAN_POINT('Ctrl Pts',(60.0728431803877,246.36046868405,22.0046511619653)) ;
#113929=CARTESIAN_POINT('Ctrl Pts',(60.0741038367237,246.376503146741,21.978158145778)) ;
#113930=CARTESIAN_POINT('Ctrl Pts',(60.0753644930597,246.393151745223,21.9520656520359)) ;
#113931=CARTESIAN_POINT('Ctrl Pts',(60.0766251493957,246.4103913826,21.9264030453364)) ;
#113932=CARTESIAN_POINT('Ctrl Pts',(60.0794214890823,246.448631687118,21.8694792322975)) ;
#113933=CARTESIAN_POINT('Ctrl Pts',(60.082217828769,246.489932684402,21.8144495207951)) ;
#113934=CARTESIAN_POINT('Ctrl Pts',(60.0850141684556,246.534080315867,21.7616618094353)) ;
#113935=CARTESIAN_POINT('Ctrl Pts',(60.0878063276356,246.578161946956,21.7089530153048)) ;
#113936=CARTESIAN_POINT('Ctrl Pts',(60.0905984868155,246.62508145335,21.658479942422)) ;
#113937=CARTESIAN_POINT('Ctrl Pts',(60.0933906459954,246.674581773116,21.6105612289672)) ;
#113938=CARTESIAN_POINT('Ctrl Pts',(60.0961795503789,246.724024390776,21.5626983739544)) ;
#113939=CARTESIAN_POINT('Ctrl Pts',(60.0989684547623,246.776041495738,21.5173843043578)) ;
#113940=CARTESIAN_POINT('Ctrl Pts',(60.1017573591458,246.830337277652,21.4749029044874)) ;
#113941=CARTESIAN_POINT('Ctrl Pts',(60.1045445328128,246.884599365114,21.4324478673915)) ;
#113942=CARTESIAN_POINT('Ctrl Pts',(60.1073317064798,246.941136938552,21.3928223145322)) ;
#113943=CARTESIAN_POINT('Ctrl Pts',(60.1101188801468,246.999620188514,21.356270674032)) ;
#113944=CARTESIAN_POINT('Ctrl Pts',(60.1129052756417,247.058087110096,21.3197292386605)) ;
#113945=CARTESIAN_POINT('Ctrl Pts',(60.1156916711366,247.118498213693,21.28626027181)) ;
#113946=CARTESIAN_POINT('Ctrl Pts',(60.1184780666315,247.180495217874,21.2560645585811)) ;
#113947=CARTESIAN_POINT('Ctrl Pts',(60.1212646353438,247.242496076122,21.2258669682236)) ;
#113948=CARTESIAN_POINT('Ctrl Pts',(60.1240512040562,247.306082588296,21.1989432480789)) ;
#113949=CARTESIAN_POINT('Ctrl Pts',(60.1268377727685,247.370874048168,21.1754471465864)) ;
#113950=CARTESIAN_POINT('Ctrl Pts',(60.129627291991,247.435734111359,21.1519261666527)) ;
#113951=CARTESIAN_POINT('Ctrl Pts',(60.1324168112134,247.501801206085,21.1318402157681)) ;
#113952=CARTESIAN_POINT('Ctrl Pts',(60.1352063304359,247.568677869959,21.1152936577236)) ;
#113953=CARTESIAN_POINT('Ctrl Pts',(60.1379975199159,247.635594577025,21.0987371922322)) ;
#113954=CARTESIAN_POINT('Ctrl Pts',(60.1407887093959,247.703321335937,21.085724430048)) ;
#113955=CARTESIAN_POINT('Ctrl Pts',(60.143579898876,247.771451606222,21.0763083766615)) ;
#113956=CARTESIAN_POINT('Ctrl Pts',(60.146375853576,247.839698190977,21.0668762478468)) ;
#113957=CARTESIAN_POINT('Ctrl Pts',(60.1491718082761,247.90834917322,21.0610531242606)) ;
#113958=CARTESIAN_POINT('Ctrl Pts',(60.1519677629761,247.976994907934,21.0588399916043)) ;
#113959=CARTESIAN_POINT('Ctrl Pts',(60.1532283737778,248.007945178576,21.0578421575077)) ;
#113960=CARTESIAN_POINT('Ctrl Pts',(60.1544889845795,248.03889441398,21.0575774690528)) ;
#113961=CARTESIAN_POINT('Ctrl Pts',(60.1557495953812,248.069805409754,21.0580425688778)) ;
#113962=CARTESIAN_POINT('Ctrl Pts',(60.1585459356804,248.138373490443,21.0590742730182)) ;
#113963=CARTESIAN_POINT('Ctrl Pts',(60.1613422759796,248.207021923866,21.063704453176)) ;
#113964=CARTESIAN_POINT('Ctrl Pts',(60.1641386162787,248.275342358042,21.0719432798769)) ;
#113965=CARTESIAN_POINT('Ctrl Pts',(60.166930776137,248.343560655314,21.0801697897905)) ;
#113966=CARTESIAN_POINT('Ctrl Pts',(60.1697229359952,248.411451443118,21.0919941806046)) ;
#113967=CARTESIAN_POINT('Ctrl Pts',(60.1725150958534,248.478607460541,21.1073746202483)) ;
#113968=CARTESIAN_POINT('Ctrl Pts',(60.1753040010076,248.545685197001,21.1227371315563)) ;
#113969=CARTESIAN_POINT('Ctrl Pts',(60.1780929061617,248.612029387947,21.1416473499608)) ;
#113970=CARTESIAN_POINT('Ctrl Pts',(60.1808818113159,248.677240788408,21.164012013665)) ;
#113971=CARTESIAN_POINT('Ctrl Pts',(60.1836689858104,248.742411721828,21.1863627989404)) ;
#113972=CARTESIAN_POINT('Ctrl Pts',(60.1864561603049,248.806450796026,21.2121636180408)) ;
#113973=CARTESIAN_POINT('Ctrl Pts',(60.1892433347993,248.868973313096,21.2412711980438)) ;
#113974=CARTESIAN_POINT('Ctrl Pts',(60.1920297311767,248.93147837527,21.2703706518581)) ;
#113975=CARTESIAN_POINT('Ctrl Pts',(60.1948161275541,248.992467276113,21.3027748267235)) ;
#113976=CARTESIAN_POINT('Ctrl Pts',(60.1976025239315,249.051576387676,21.3382927902592)) ;
#113977=CARTESIAN_POINT('Ctrl Pts',(60.2003890935795,249.110689174908,21.3738129624615)) ;
#113978=CARTESIAN_POINT('Ctrl Pts',(60.2031756632276,249.167921521403,21.4124470527529)) ;
#113979=CARTESIAN_POINT('Ctrl Pts',(60.2059622328756,249.222937010551,21.4539596893355)) ;
#113980=CARTESIAN_POINT('Ctrl Pts',(60.2087517531066,249.278010753319,21.4955162819267)) ;
#113981=CARTESIAN_POINT('Ctrl Pts',(60.2115412733376,249.330862561746,21.539957207296)) ;
#113982=CARTESIAN_POINT('Ctrl Pts',(60.2143307935686,249.381188288939,21.5870061268527)) ;
#113983=CARTESIAN_POINT('Ctrl Pts',(60.2171219841002,249.431544150019,21.6340832182205)) ;
#113984=CARTESIAN_POINT('Ctrl Pts',(60.2199131746318,249.479370579081,21.6837710581063)) ;
#113985=CARTESIAN_POINT('Ctrl Pts',(60.2227043651634,249.524401538805,21.7357577024867)) ;
#113986=CARTESIAN_POINT('Ctrl Pts',(60.2255003209692,249.569509377863,21.7878331013293)) ;
#113987=CARTESIAN_POINT('Ctrl Pts',(60.2282962767749,249.611811921378,21.8422147502424)) ;
#113988=CARTESIAN_POINT('Ctrl Pts',(60.2310922325807,249.651085052258,21.8985597473098)) ;
#113989=CARTESIAN_POINT('Ctrl Pts',(60.2323528355094,249.668791993013,21.9239638213565)) ;
#113990=CARTESIAN_POINT('Ctrl Pts',(60.2336134384381,249.685883721363,21.9497666479969)) ;
#113991=CARTESIAN_POINT('Ctrl Pts',(60.2348740413668,249.702342772904,21.975935206342)) ;
#113992=CARTESIAN_POINT('Ctrl Pts',(60.2377412276648,249.739778166702,22.0354544492515)) ;
#113993=CARTESIAN_POINT('Ctrl Pts',(60.2406084139629,249.774078324787,22.0970909793996)) ;
#113994=CARTESIAN_POINT('Ctrl Pts',(60.2434756002609,249.805004331575,22.1604906728236)) ;
#113995=CARTESIAN_POINT('Ctrl Pts',(60.2464819941489,249.837431857423,22.2269685472966)) ;
#113996=CARTESIAN_POINT('Ctrl Pts',(60.2494883880369,249.866148909367,22.2953847829146)) ;
#113997=CARTESIAN_POINT('Ctrl Pts',(60.2524947819249,249.890931274391,22.3652967237239)) ;
#113998=CARTESIAN_POINT('Ctrl Pts',(60.2553516150131,249.9144807769,22.4317307151471)) ;
#113999=CARTESIAN_POINT('Ctrl Pts',(60.2582084481014,249.934477515015,22.4995146613668)) ;
#114000=CARTESIAN_POINT('Ctrl Pts',(60.2610652811897,249.950776875416,22.5682452551403)) ;
#114001=CARTESIAN_POINT('Ctrl Pts',(60.2639190906064,249.967058984577,22.6369031044661)) ;
#114002=CARTESIAN_POINT('Ctrl Pts',(60.266772900023,249.979651385476,22.7065051674995)) ;
#114003=CARTESIAN_POINT('Ctrl Pts',(60.2696267094397,249.988459223616,22.7766329163271)) ;
#114004=CARTESIAN_POINT('Ctrl Pts',(60.2724778878943,249.997258941702,22.846696013518)) ;
#114005=CARTESIAN_POINT('Ctrl Pts',(60.2753290663488,250.002280980204,22.917283379616)) ;
#114006=CARTESIAN_POINT('Ctrl Pts',(60.2781802448034,250.003481818976,22.9879677588878)) ;
#114007=CARTESIAN_POINT('Ctrl Pts',(60.2786376055079,250.003674446858,22.9993063187197)) ;
#114008=CARTESIAN_POINT('Ctrl Pts',(60.2790949662123,250.003768856915,23.0106473625013)) ;
#114009=CARTESIAN_POINT('Ctrl Pts',(60.2795523269168,250.003764993894,23.0219891151141)) ;
#114010=CARTESIAN_POINT('',(60.7795523268794,250.003764678819,23.02261824718)) ;
#114011=CARTESIAN_POINT('Ctrl Pts',(60.2795523269397,250.003764993893,23.0219891156808)) ;
#114012=CARTESIAN_POINT('Ctrl Pts',(60.2825667509946,250.00373953304,23.0967416065853)) ;
#114013=CARTESIAN_POINT('Ctrl Pts',(60.2855811750496,249.999440984289,23.1713682677577)) ;
#114014=CARTESIAN_POINT('Ctrl Pts',(60.2885955991045,249.99093752082,23.2453948557862)) ;
#114015=CARTESIAN_POINT('Ctrl Pts',(60.2916177917231,249.982412142817,23.3196122199815)) ;
#114016=CARTESIAN_POINT('Ctrl Pts',(60.2946399843418,249.969660279399,23.3932260736516)) ;
#114017=CARTESIAN_POINT('Ctrl Pts',(60.2976621769605,249.952801046831,23.4657734140421)) ;
#114018=CARTESIAN_POINT('Ctrl Pts',(60.3006968067865,249.935872433585,23.5386193079761)) ;
#114019=CARTESIAN_POINT('Ctrl Pts',(60.3037314366125,249.914802725252,23.6103895617087)) ;
#114020=CARTESIAN_POINT('Ctrl Pts',(60.3067660664385,249.889761187779,23.6806355186404)) ;
#114021=CARTESIAN_POINT('Ctrl Pts',(60.3091768734098,249.869867389664,23.7364411530614)) ;
#114022=CARTESIAN_POINT('Ctrl Pts',(60.311587680381,249.847467869694,23.7912851094937)) ;
#114023=CARTESIAN_POINT('Ctrl Pts',(60.3139984873523,249.822668197138,23.8449534397057)) ;
#114024=CARTESIAN_POINT('Ctrl Pts',(60.3167948593909,249.793902264516,23.9072050507863)) ;
#114025=CARTESIAN_POINT('Ctrl Pts',(60.3195912314296,249.761814742582,23.9680699192819)) ;
#114026=CARTESIAN_POINT('Ctrl Pts',(60.3223876034682,249.726562036934,24.0271706886639)) ;
#114027=CARTESIAN_POINT('Ctrl Pts',(60.3251797948775,249.691362034751,24.0861831012709)) ;
#114028=CARTESIAN_POINT('Ctrl Pts',(60.3279719862867,249.653006490149,24.1434362310788)) ;
#114029=CARTESIAN_POINT('Ctrl Pts',(60.3307641776959,249.611698894999,24.1985748200451)) ;
#114030=CARTESIAN_POINT('Ctrl Pts',(60.3335531139729,249.570439456177,24.2536491285323)) ;
#114031=CARTESIAN_POINT('Ctrl Pts',(60.3363420502498,249.526235094886,24.3066134011991)) ;
#114032=CARTESIAN_POINT('Ctrl Pts',(60.3391309865267,249.479333055782,24.357140575122)) ;
#114033=CARTESIAN_POINT('Ctrl Pts',(60.3419181918599,249.432460126269,24.4076363895265)) ;
#114034=CARTESIAN_POINT('Ctrl Pts',(60.344705397193,249.382893173611,24.4556977469108)) ;
#114035=CARTESIAN_POINT('Ctrl Pts',(60.3474926025261,249.330919248694,24.5010311729304)) ;
#114036=CARTESIAN_POINT('Ctrl Pts',(60.3502790294131,249.278959839716,24.5463519376537)) ;
#114037=CARTESIAN_POINT('Ctrl Pts',(60.3530654563001,249.224595162818,24.588945961132)) ;
#114038=CARTESIAN_POINT('Ctrl Pts',(60.355851883187,249.168147279082,24.6285583650342)) ;
#114039=CARTESIAN_POINT('Ctrl Pts',(60.3586384829702,249.111695892784,24.6681732268647)) ;
#114040=CARTESIAN_POINT('Ctrl Pts',(60.3614250827535,249.05316144625,24.704805821987)) ;
#114041=CARTESIAN_POINT('Ctrl Pts',(60.3642116825367,248.992895575888,24.7382441744978)) ;
#114042=CARTESIAN_POINT('Ctrl Pts',(60.3670012321378,248.932565909735,24.7717179239281)) ;
#114043=CARTESIAN_POINT('Ctrl Pts',(60.3697907817388,248.870501592039,24.8019904442138)) ;
#114044=CARTESIAN_POINT('Ctrl Pts',(60.3725803313399,248.807078608147,24.8288958760517)) ;
#114045=CARTESIAN_POINT('Ctrl Pts',(60.375371550846,248.743617657424,24.8558174142589)) ;
#114046=CARTESIAN_POINT('Ctrl Pts',(60.3781627703521,248.678796883113,24.8793676847712)) ;
#114047=CARTESIAN_POINT('Ctrl Pts',(60.3809539898581,248.613009350054,24.8994301068453)) ;
#114048=CARTESIAN_POINT('Ctrl Pts',(60.3837499737347,248.547109523362,24.9195267737398)) ;
#114049=CARTESIAN_POINT('Ctrl Pts',(60.3865459576112,248.480240120589,24.9361235922249)) ;
#114050=CARTESIAN_POINT('Ctrl Pts',(60.3893419414877,248.412805492076,24.9491548572234)) ;
#114051=CARTESIAN_POINT('Ctrl Pts',(60.3906022721044,248.382408347209,24.9550288904715)) ;
#114052=CARTESIAN_POINT('Ctrl Pts',(60.3918626027211,248.35189643516,24.9601791446228)) ;
#114053=CARTESIAN_POINT('Ctrl Pts',(60.3931229333378,248.321306998146,24.9646030573876)) ;
#114054=CARTESIAN_POINT('Ctrl Pts',(60.3959192896097,248.253436740206,24.9744186058175)) ;
#114055=CARTESIAN_POINT('Ctrl Pts',(60.3987156458815,248.184918568129,24.9806935219423)) ;
#114056=CARTESIAN_POINT('Ctrl Pts',(60.4015120021534,248.116154103306,24.9833532460255)) ;
#114057=CARTESIAN_POINT('Ctrl Pts',(60.4043041784366,248.047492427488,24.9860089943578)) ;
#114058=CARTESIAN_POINT('Ctrl Pts',(60.4070963547199,247.978585676197,24.9850602573779)) ;
#114059=CARTESIAN_POINT('Ctrl Pts',(60.4098885310032,247.909842609292,24.980483997236)) ;
#114060=CARTESIAN_POINT('Ctrl Pts',(60.4126774531614,247.84117965858,24.9759130704688)) ;
#114061=CARTESIAN_POINT('Ctrl Pts',(60.4154663753196,247.772680500832,24.9677230495881)) ;
#114062=CARTESIAN_POINT('Ctrl Pts',(60.4182552974779,247.70475410613,24.9559429470064)) ;
#114063=CARTESIAN_POINT('Ctrl Pts',(60.4210424893246,247.636869854527,24.9441701530717)) ;
#114064=CARTESIAN_POINT('Ctrl Pts',(60.4238296811713,247.569558143552,24.9288117797785)) ;
#114065=CARTESIAN_POINT('Ctrl Pts',(60.426616873018,247.503221480302,24.9099485208826)) ;
#114066=CARTESIAN_POINT('Ctrl Pts',(60.4294032870659,247.436903329079,24.8910905260014)) ;
#114067=CARTESIAN_POINT('Ctrl Pts',(60.4321897011139,247.371560157267,24.8687297214978)) ;
#114068=CARTESIAN_POINT('Ctrl Pts',(60.4349761151619,247.307581196557,24.8429971909249)) ;
#114069=CARTESIAN_POINT('Ctrl Pts',(60.4377627027695,247.243598250739,24.8172630575292)) ;
#114070=CARTESIAN_POINT('Ctrl Pts',(60.4405492903771,247.180980139128,24.7881569666392)) ;
#114071=CARTESIAN_POINT('Ctrl Pts',(60.4433358779846,247.120096245115,24.7558581823426)) ;
#114072=CARTESIAN_POINT('Ctrl Pts',(60.4461254164814,247.059147877398,24.723525194875)) ;
#114073=CARTESIAN_POINT('Ctrl Pts',(60.4489149549781,246.999937826622,24.6879929972857)) ;
#114074=CARTESIAN_POINT('Ctrl Pts',(60.4517044934749,246.942810084486,24.6494864044494)) ;
#114075=CARTESIAN_POINT('Ctrl Pts',(60.454495702473,246.885648131683,24.6109567521297)) ;
#114076=CARTESIAN_POINT('Ctrl Pts',(60.4572869114711,246.830571361334,24.5694494549501)) ;
#114077=CARTESIAN_POINT('Ctrl Pts',(60.4600781204692,246.777891759898,24.5252305072802)) ;
#114078=CARTESIAN_POINT('Ctrl Pts',(60.4628740948521,246.725122219454,24.4809360653353)) ;
#114079=CARTESIAN_POINT('Ctrl Pts',(60.465670069235,246.674758374516,24.4339210680221)) ;
#114080=CARTESIAN_POINT('Ctrl Pts',(60.4684660436179,246.62707570927,24.3844887021715)) ;
#114081=CARTESIAN_POINT('Ctrl Pts',(60.4697264888531,246.60558002298,24.362204238344)) ;
#114082=CARTESIAN_POINT('Ctrl Pts',(60.4709869340882,246.584628680812,24.3394289493908)) ;
#114083=CARTESIAN_POINT('Ctrl Pts',(60.4722473793233,246.564244136686,24.316192670422)) ;
#114084=CARTESIAN_POINT('Ctrl Pts',(60.4750435067742,246.519023779772,24.2646461250667)) ;
#114085=CARTESIAN_POINT('Ctrl Pts',(60.4778396342251,246.476418112565,24.2106267345541)) ;
#114086=CARTESIAN_POINT('Ctrl Pts',(60.480635761676,246.436708552273,24.1544304985185)) ;
#114087=CARTESIAN_POINT('Ctrl Pts',(60.483427708114,246.397058369168,24.0983182919802)) ;
#114088=CARTESIAN_POINT('Ctrl Pts',(60.486219654552,246.360295979102,24.0400360979995)) ;
#114089=CARTESIAN_POINT('Ctrl Pts',(60.4890116009901,246.326663499278,23.9799139891246)) ;
#114090=CARTESIAN_POINT('Ctrl Pts',(60.4918002929304,246.293070223941,23.9198619629935)) ;
#114091=CARTESIAN_POINT('Ctrl Pts',(60.4945889848707,246.262599851231,23.8579747080533)) ;
#114092=CARTESIAN_POINT('Ctrl Pts',(60.497377676811,246.235450977629,23.7946108488587)) ;
#114093=CARTESIAN_POINT('Ctrl Pts',(60.5001646383492,246.208318950086,23.7312863073662)) ;
#114094=CARTESIAN_POINT('Ctrl Pts',(60.5029515998873,246.184504525948,23.6664874294933)) ;
#114095=CARTESIAN_POINT('Ctrl Pts',(60.5057385614254,246.164159451687,23.6005955951925)) ;
#114096=CARTESIAN_POINT('Ctrl Pts',(60.5085247454293,246.143820053498,23.5347221440525)) ;
#114097=CARTESIAN_POINT('Ctrl Pts',(60.5113109294331,246.126948228345,23.4677568106951)) ;
#114098=CARTESIAN_POINT('Ctrl Pts',(60.5140971134369,246.113646241324,23.4000973140725)) ;
#114099=CARTESIAN_POINT('Ctrl Pts',(60.5168834716199,246.100343422724,23.3324335876949)) ;
#114100=CARTESIAN_POINT('Ctrl Pts',(60.5196698298029,246.090610977498,23.2640760940751)) ;
#114101=CARTESIAN_POINT('Ctrl Pts',(60.522456187986,246.084499958264,23.1954321751935)) ;
#114102=CARTESIAN_POINT('Ctrl Pts',(60.5252454995637,246.078382461667,23.1267154973289)) ;
#114103=CARTESIAN_POINT('Ctrl Pts',(60.5280348111414,246.075894094999,23.0577122782262)) ;
#114104=CARTESIAN_POINT('Ctrl Pts',(60.5308241227191,246.077033881316,22.9888334013953)) ;
#114105=CARTESIAN_POINT('Ctrl Pts',(60.5336151059076,246.078174350696,22.9199132460377)) ;
#114106=CARTESIAN_POINT('Ctrl Pts',(60.5364060890962,246.082947266486,22.8511180710345)) ;
#114107=CARTESIAN_POINT('Ctrl Pts',(60.5391970722847,246.091299682121,22.7828543720631)) ;
#114108=CARTESIAN_POINT('Ctrl Pts',(60.5419928249112,246.09966637098,22.7144740190451)) ;
#114109=CARTESIAN_POINT('Ctrl Pts',(60.5447885775378,246.111624682532,22.6466274378222)) ;
#114110=CARTESIAN_POINT('Ctrl Pts',(60.5475843301643,246.127070592193,22.579710792595)) ;
#114111=CARTESIAN_POINT('Ctrl Pts',(60.5488468285458,246.134045614146,22.5494927556)) ;
#114112=CARTESIAN_POINT('Ctrl Pts',(60.5501093269274,246.141731158904,22.5194641413635)) ;
#114113=CARTESIAN_POINT('Ctrl Pts',(60.5513718253089,246.150114385329,22.4896602111498)) ;
#114114=CARTESIAN_POINT('Ctrl Pts',(60.5541685645237,246.168685259107,22.4236372984863)) ;
#114115=CARTESIAN_POINT('Ctrl Pts',(60.5569653037384,246.190755923697,22.3584592614936)) ;
#114116=CARTESIAN_POINT('Ctrl Pts',(60.5597620429532,246.216231499799,22.2945235033544)) ;
#114117=CARTESIAN_POINT('Ctrl Pts',(60.5625546005643,246.241668985555,22.2306833401114)) ;
#114118=CARTESIAN_POINT('Ctrl Pts',(60.5653471581755,246.270501098344,22.1680822214019)) ;
#114119=CARTESIAN_POINT('Ctrl Pts',(60.5681397157866,246.302582973991,22.1071031637326)) ;
#114120=CARTESIAN_POINT('Ctrl Pts',(60.5709290150576,246.33462741669,22.0461952560776)) ;
#114121=CARTESIAN_POINT('Ctrl Pts',(60.5737183143286,246.36991386385,21.9869060827224)) ;
#114122=CARTESIAN_POINT('Ctrl Pts',(60.5765076135996,246.408249795115,21.929597728054)) ;
#114123=CARTESIAN_POINT('Ctrl Pts',(60.5792951797171,246.446561906041,21.8723249823906)) ;
#114124=CARTESIAN_POINT('Ctrl Pts',(60.5820827458347,246.487919469867,21.817031020669)) ;
#114125=CARTESIAN_POINT('Ctrl Pts',(60.5848703119522,246.532085354106,21.7640510483844)) ;
#114126=CARTESIAN_POINT('Ctrl Pts',(60.5876570968761,246.5762388612,21.7110859233243)) ;
#114127=CARTESIAN_POINT('Ctrl Pts',(60.5904438817999,246.623198812189,21.6604338769742)) ;
#114128=CARTESIAN_POINT('Ctrl Pts',(60.5932306667238,246.672687406079,21.6123975352432)) ;
#114129=CARTESIAN_POINT('Ctrl Pts',(60.5960176212559,246.722179011925,21.564358269943)) ;
#114130=CARTESIAN_POINT('Ctrl Pts',(60.5988045757879,246.774199212344,21.5189353652299)) ;
#114131=CARTESIAN_POINT('Ctrl Pts',(60.60159153032,246.82843422262,21.4763937576798)) ;
#114132=CARTESIAN_POINT('Ctrl Pts',(60.6043814273241,246.882726494326,21.4338072346176)) ;
#114133=CARTESIAN_POINT('Ctrl Pts',(60.6071713243282,246.939237855736,21.3941083830617)) ;
#114134=CARTESIAN_POINT('Ctrl Pts',(60.6099612213323,246.997623190867,21.3575204508188)) ;
#114135=CARTESIAN_POINT('Ctrl Pts',(60.612752784535,247.056043395231,21.3209106673166)) ;
#114136=CARTESIAN_POINT('Ctrl Pts',(60.6155443477377,247.116339371843,21.2874157392378)) ;
#114137=CARTESIAN_POINT('Ctrl Pts',(60.6183359109405,247.178141348584,21.2572129562899)) ;
#114138=CARTESIAN_POINT('Ctrl Pts',(60.6211322292867,247.240048598697,21.2269587259782)) ;
#114139=CARTESIAN_POINT('Ctrl Pts',(60.6239285476329,247.303466517481,21.2000080246737)) ;
#114140=CARTESIAN_POINT('Ctrl Pts',(60.6267248659792,247.3680061454,21.1764896907646)) ;
#114141=CARTESIAN_POINT('Ctrl Pts',(60.6279820010843,247.397021093585,21.1659166016136)) ;
#114142=CARTESIAN_POINT('Ctrl Pts',(60.6292391361893,247.426262562519,21.1560365558167)) ;
#114143=CARTESIAN_POINT('Ctrl Pts',(60.6304962712944,247.455694464905,21.1468579103587)) ;
#114144=CARTESIAN_POINT('Ctrl Pts',(60.6332926395102,247.521162715715,21.1264409541228)) ;
#114145=CARTESIAN_POINT('Ctrl Pts',(60.636089007726,247.587830124222,21.1094179783846)) ;
#114146=CARTESIAN_POINT('Ctrl Pts',(60.6388853759418,247.655311867762,21.095926032517)) ;
#114147=CARTESIAN_POINT('Ctrl Pts',(60.6416775684694,247.722692843916,21.0824542335521)) ;
#114148=CARTESIAN_POINT('Ctrl Pts',(60.6444697609971,247.79088526415,21.0725030948673)) ;
#114149=CARTESIAN_POINT('Ctrl Pts',(60.6472619535248,247.85948912198,21.0661599171608)) ;
#114150=CARTESIAN_POINT('Ctrl Pts',(60.650050898095,247.928013177859,21.0598241180184)) ;
#114151=CARTESIAN_POINT('Ctrl Pts',(60.6528398426652,247.996947234345,21.0570879894057)) ;
#114152=CARTESIAN_POINT('Ctrl Pts',(60.6556287872354,248.065882857958,21.0579874678413)) ;
#114153=CARTESIAN_POINT('Ctrl Pts',(60.658416005296,248.13477580664,21.0588863894505)) ;
#114154=CARTESIAN_POINT('Ctrl Pts',(60.6612032233566,248.203669830839,21.0634164468891)) ;
#114155=CARTESIAN_POINT('Ctrl Pts',(60.6639904414172,248.27215471858,21.0715615229857)) ;
#114156=CARTESIAN_POINT('Ctrl Pts',(60.6667768854009,248.340620586436,21.0797043370005)) ;
#114157=CARTESIAN_POINT('Ctrl Pts',(60.6695633293846,248.408677056274,21.0914601185186)) ;
#114158=CARTESIAN_POINT('Ctrl Pts',(60.6723497733684,248.475919068293,21.1067608964036)) ;
#114159=CARTESIAN_POINT('Ctrl Pts',(60.6751363945573,248.543165356601,21.1220626473492)) ;
#114160=CARTESIAN_POINT('Ctrl Pts',(60.6779230157463,248.609596606267,21.1409097308469)) ;
#114161=CARTESIAN_POINT('Ctrl Pts',(60.6807096369353,248.674819748712,21.16318346548)) ;
#114162=CARTESIAN_POINT('Ctrl Pts',(60.6834992141911,248.740112080312,21.1854808282428)) ;
#114163=CARTESIAN_POINT('Ctrl Pts',(60.6862887914468,248.804193281804,21.2112119374179)) ;
#114164=CARTESIAN_POINT('Ctrl Pts',(60.6890783687026,248.86668816404,21.2402091224139)) ;
#114165=CARTESIAN_POINT('Ctrl Pts',(60.6918696194718,248.929220537989,21.2692237033)) ;
#114166=CARTESIAN_POINT('Ctrl Pts',(60.694660870241,248.990164264906,21.3015080298612)) ;
#114167=CARTESIAN_POINT('Ctrl Pts',(60.6974521210102,249.049169256588,21.3368487146709)) ;
#114168=CARTESIAN_POINT('Ctrl Pts',(60.7002481412775,249.108275071955,21.3722497872205)) ;
#114169=CARTESIAN_POINT('Ctrl Pts',(60.7030441615447,249.165435133589,21.4107173671274)) ;
#114170=CARTESIAN_POINT('Ctrl Pts',(60.7058401818119,249.220329523796,21.45199557664)) ;
#114171=CARTESIAN_POINT('Ctrl Pts',(60.7071003603012,249.2450706641,21.4705998451125)) ;
#114172=CARTESIAN_POINT('Ctrl Pts',(60.7083605387906,249.269352034815,21.4897745194347)) ;
#114173=CARTESIAN_POINT('Ctrl Pts',(60.7096207172799,249.293146769467,21.509493702763)) ;
#114174=CARTESIAN_POINT('Ctrl Pts',(60.7123779967535,249.345209817673,21.5526394157617)) ;
#114175=CARTESIAN_POINT('Ctrl Pts',(60.7151352762271,249.395157754924,21.5985742313354)) ;
#114176=CARTESIAN_POINT('Ctrl Pts',(60.7178925557008,249.442670499818,21.6470600456544)) ;
#114177=CARTESIAN_POINT('Ctrl Pts',(60.7206451164748,249.490101933272,21.6954628832595)) ;
#114178=CARTESIAN_POINT('Ctrl Pts',(60.7233976772489,249.535106096424,21.7464076952068)) ;
#114179=CARTESIAN_POINT('Ctrl Pts',(60.726150238023,249.577396023049,21.7996162880111)) ;
#114180=CARTESIAN_POINT('Ctrl Pts',(60.7289001789681,249.619645699019,21.8527742380057)) ;
#114181=CARTESIAN_POINT('Ctrl Pts',(60.7316501199133,249.659185944413,21.9081913054828)) ;
#114182=CARTESIAN_POINT('Ctrl Pts',(60.7344000608584,249.695767790971,21.9655537424747)) ;
#114183=CARTESIAN_POINT('Ctrl Pts',(60.7371483861221,249.732328144482,22.0228824771329)) ;
#114184=CARTESIAN_POINT('Ctrl Pts',(60.7398967113857,249.765933273921,22.0821538895004)) ;
#114185=CARTESIAN_POINT('Ctrl Pts',(60.7426450366494,249.796376751589,22.1430241836579)) ;
#114186=CARTESIAN_POINT('Ctrl Pts',(60.7453927480107,249.826813428999,22.2038808810211)) ;
#114187=CARTESIAN_POINT('Ctrl Pts',(60.7481404593721,249.854089631235,22.2663352984914)) ;
#114188=CARTESIAN_POINT('Ctrl Pts',(60.7508881707335,249.878045195176,22.3300196850955)) ;
#114189=CARTESIAN_POINT('Ctrl Pts',(60.7536378075823,249.902017546229,22.3937486991993)) ;
#114190=CARTESIAN_POINT('Ctrl Pts',(60.7563874444311,249.922664433148,22.4587089295423)) ;
#114191=CARTESIAN_POINT('Ctrl Pts',(60.7591370812799,249.939874614559,22.5245145748941)) ;
#114192=CARTESIAN_POINT('Ctrl Pts',(60.7618877928552,249.957091522762,22.5903459411223)) ;
#114193=CARTESIAN_POINT('Ctrl Pts',(60.7646385044305,249.970868947996,22.6570228845858)) ;
#114194=CARTESIAN_POINT('Ctrl Pts',(60.7673892160059,249.981146754236,22.724149206885)) ;
#114195=CARTESIAN_POINT('Ctrl Pts',(60.7701439626157,249.99143963705,22.7913739971708)) ;
#114196=CARTESIAN_POINT('Ctrl Pts',(60.7728987092256,249.998222606019,22.8590489785077)) ;
#114197=CARTESIAN_POINT('Ctrl Pts',(60.7756534558355,250.001487481974,22.9267737995547)) ;
#114198=CARTESIAN_POINT('Ctrl Pts',(60.7769530795168,250.003027772502,22.9587247532035)) ;
#114199=CARTESIAN_POINT('Ctrl Pts',(60.7782527031981,250.003785785992,22.9906868126438)) ;
#114200=CARTESIAN_POINT('Ctrl Pts',(60.7795523268794,250.003764678819,23.02261824718)) ;
#114201=CARTESIAN_POINT('',(60.9402651077866,247.187596811119,24.7900173288734)) ;
#114202=CARTESIAN_POINT('Ctrl Pts',(60.7795523269168,250.003764678818,23.0226182480982)) ;
#114203=CARTESIAN_POINT('Ctrl Pts',(60.7826166056997,250.003714911868,23.0979068249079)) ;
#114204=CARTESIAN_POINT('Ctrl Pts',(60.7856808844825,249.999334962485,23.1730560108799)) ;
#114205=CARTESIAN_POINT('Ctrl Pts',(60.7887451632653,249.990671827291,23.247695868984)) ;
#114206=CARTESIAN_POINT('Ctrl Pts',(60.7915457584845,249.982754161592,23.3159129094631)) ;
#114207=CARTESIAN_POINT('Ctrl Pts',(60.7943463537037,249.971237999381,23.3838458374833)) ;
#114208=CARTESIAN_POINT('Ctrl Pts',(60.7971469489229,249.956154825269,23.4510863734446)) ;
#114209=CARTESIAN_POINT('Ctrl Pts',(60.7999433589634,249.941094191287,23.518226425889)) ;
#114210=CARTESIAN_POINT('Ctrl Pts',(60.802739769004,249.922477232334,23.5846756664621)) ;
#114211=CARTESIAN_POINT('Ctrl Pts',(60.8055361790446,249.900387055117,23.6500321941365)) ;
#114212=CARTESIAN_POINT('Ctrl Pts',(60.8083293066438,249.878322807471,23.7153120059637)) ;
#114213=CARTESIAN_POINT('Ctrl Pts',(60.8111224342431,249.852793595527,23.7795011913223)) ;
#114214=CARTESIAN_POINT('Ctrl Pts',(60.8139155618424,249.823932876028,23.8422110442841)) ;
#114215=CARTESIAN_POINT('Ctrl Pts',(60.8167069388807,249.795090244656,23.9048815945579)) ;
#114216=CARTESIAN_POINT('Ctrl Pts',(60.819498315919,249.762920452405,23.9660742085282)) ;
#114217=CARTESIAN_POINT('Ctrl Pts',(60.8222896929573,249.727605241829,24.0254197022134)) ;
#114218=CARTESIAN_POINT('Ctrl Pts',(60.825080265588,249.692300208244,24.0847480939579)) ;
#114219=CARTESIAN_POINT('Ctrl Pts',(60.8278708382187,249.653851806104,24.1422300021104)) ;
#114220=CARTESIAN_POINT('Ctrl Pts',(60.8306614108495,249.612487076523,24.1975219976233)) ;
#114221=CARTESIAN_POINT('Ctrl Pts',(60.8334521240458,249.571120263334,24.2528167782825)) ;
#114222=CARTESIAN_POINT('Ctrl Pts',(60.8362428372421,249.526837126104,24.3059210371075)) ;
#114223=CARTESIAN_POINT('Ctrl Pts',(60.8390335504385,249.479906196998,24.3565228691157)) ;
#114224=CARTESIAN_POINT('Ctrl Pts',(60.8418271369309,249.432926948183,24.407176800366)) ;
#114225=CARTESIAN_POINT('Ctrl Pts',(60.8446207234232,249.38329480011,24.4553228035038)) ;
#114226=CARTESIAN_POINT('Ctrl Pts',(60.8474143099156,249.331315818112,24.5006851779959)) ;
#114227=CARTESIAN_POINT('Ctrl Pts',(60.8502095281215,249.27930647557,24.5460740483204)) ;
#114228=CARTESIAN_POINT('Ctrl Pts',(60.8530047463274,249.224947955461,24.5886757515398)) ;
#114229=CARTESIAN_POINT('Ctrl Pts',(60.8557999645333,249.16857797034,24.6282560405289)) ;
#114230=CARTESIAN_POINT('Ctrl Pts',(60.8585998475443,249.112113912064,24.6679023831583)) ;
#114231=CARTESIAN_POINT('Ctrl Pts',(60.8613997305554,249.053632103304,24.704516988195)) ;
#114232=CARTESIAN_POINT('Ctrl Pts',(60.8641996135665,248.993496900582,24.7379103933977)) ;
#114233=CARTESIAN_POINT('Ctrl Pts',(60.8654229454614,248.967222477255,24.7525007236018)) ;
#114234=CARTESIAN_POINT('Ctrl Pts',(60.8666462773563,248.940632700595,24.7664767340529)) ;
#114235=CARTESIAN_POINT('Ctrl Pts',(60.8678696092512,248.913759119968,24.7798255214544)) ;
#114236=CARTESIAN_POINT('Ctrl Pts',(60.8706315295515,248.853086551723,24.8099631211221)) ;
#114237=CARTESIAN_POINT('Ctrl Pts',(60.8733934498519,248.790720386366,24.8370223887974)) ;
#114238=CARTESIAN_POINT('Ctrl Pts',(60.8761553701522,248.727009736357,24.8608077898689)) ;
#114239=CARTESIAN_POINT('Ctrl Pts',(60.878912687101,248.663405274249,24.8845535473044)) ;
#114240=CARTESIAN_POINT('Ctrl Pts',(60.8816700040498,248.598461244098,24.905036095618)) ;
#114241=CARTESIAN_POINT('Ctrl Pts',(60.8844273209986,248.532549844046,24.9221064936684)) ;
#114242=CARTESIAN_POINT('Ctrl Pts',(60.8871820798996,248.466699592027,24.9391610549855)) ;
#114243=CARTESIAN_POINT('Ctrl Pts',(60.8899368388007,248.39988423402,24.9528096133014)) ;
#114244=CARTESIAN_POINT('Ctrl Pts',(60.8926915977017,248.332492926079,24.9629524282286)) ;
#114245=CARTESIAN_POINT('Ctrl Pts',(60.8954447975409,248.265139758393,24.9730895028078)) ;
#114246=CARTESIAN_POINT('Ctrl Pts',(60.8981979973802,248.197211784568,24.9797246929004)) ;
#114247=CARTESIAN_POINT('Ctrl Pts',(60.9009511972195,248.129108262437,24.9828093554767)) ;
#114248=CARTESIAN_POINT('Ctrl Pts',(60.9037038347724,248.061018649097,24.9858933880721)) ;
#114249=CARTESIAN_POINT('Ctrl Pts',(60.9064564723254,247.992754062083,24.9854283104596)) ;
#114250=CARTESIAN_POINT('Ctrl Pts',(60.9092091098783,247.924716804232,24.9814174940973)) ;
#114251=CARTESIAN_POINT('Ctrl Pts',(60.911963958828,247.856624887036,24.9774034555504)) ;
#114252=CARTESIAN_POINT('Ctrl Pts',(60.9147188077776,247.7887611682,24.9698380167252)) ;
#114253=CARTESIAN_POINT('Ctrl Pts',(60.9174736567273,247.721524649355,24.9587766063328)) ;
#114254=CARTESIAN_POINT('Ctrl Pts',(60.920229606145,247.654261271819,24.947710777285)) ;
#114255=CARTESIAN_POINT('Ctrl Pts',(60.9229855555627,247.587626086452,24.9331463029519)) ;
#114256=CARTESIAN_POINT('Ctrl Pts',(60.9257415049803,247.522006821555,24.9151895572998)) ;
#114257=CARTESIAN_POINT('Ctrl Pts',(60.9285021102181,247.456276701397,24.8972024760485)) ;
#114258=CARTESIAN_POINT('Ctrl Pts',(60.9312627154558,247.391566408411,24.8758118376269)) ;
#114259=CARTESIAN_POINT('Ctrl Pts',(60.9340233206936,247.328246605691,24.8511733165261)) ;
#114260=CARTESIAN_POINT('Ctrl Pts',(60.9361039163912,247.28052413262,24.8326039099705)) ;
#114261=CARTESIAN_POINT('Ctrl Pts',(60.9381845120889,247.233591139334,24.8121906608919)) ;
#114262=CARTESIAN_POINT('Ctrl Pts',(60.9402651077866,247.187596811119,24.7900173288734)) ;
#114263=CARTESIAN_POINT('',(60.9402651077866,247.14398687089,24.7683227969256)) ;
#114264=CARTESIAN_POINT('Ctrl Pts',(60.9402651077866,247.187596811119,24.7900173288734)) ;
#114265=CARTESIAN_POINT('Ctrl Pts',(60.9402651077866,247.173060164376,24.7827858182242)) ;
#114266=CARTESIAN_POINT('Ctrl Pts',(60.9402651077866,247.158523517633,24.7755543075749)) ;
#114267=CARTESIAN_POINT('Ctrl Pts',(60.9402651077866,247.14398687089,24.7683227969256)) ;
#114268=CARTESIAN_POINT('',(60.9402651077866,248.892162375845,24.7903888257488)) ;
#114269=CARTESIAN_POINT('Origin',(60.9402651077866,248.040265107786,23.0213203435596)) ;
#114270=CARTESIAN_POINT('',(60.8509778886564,250.003885734109,23.0224059228657)) ;
#114271=CARTESIAN_POINT('Ctrl Pts',(60.9402651077866,248.892162375845,24.7903888257488)) ;
#114272=CARTESIAN_POINT('Ctrl Pts',(60.9138902924581,249.4784948342,24.5080396547159)) ;
#114273=CARTESIAN_POINT('Ctrl Pts',(60.8841278860814,249.963363030827,23.8364478392611)) ;
#114274=CARTESIAN_POINT('Ctrl Pts',(60.8543654797046,250.005755321297,23.1056824073686)) ;
#114275=CARTESIAN_POINT('Ctrl Pts',(60.8509778886564,250.005100724118,23.0224065945677)) ;
#114276=CARTESIAN_POINT('',(60.3509778886947,250.003765030662,23.0218706758452)) ;
#114277=CARTESIAN_POINT('Ctrl Pts',(60.8509778886564,250.003764807726,23.022405856012)) ;
#114278=CARTESIAN_POINT('Ctrl Pts',(60.8481044856214,250.003803831657,22.9518184785068)) ;
#114279=CARTESIAN_POINT('Ctrl Pts',(60.8452310825863,250.000031341811,22.8810740559555)) ;
#114280=CARTESIAN_POINT('Ctrl Pts',(60.8423576795513,249.992428256182,22.8106279325778)) ;
#114281=CARTESIAN_POINT('Ctrl Pts',(60.8396190931482,249.985181898232,22.7434870570089)) ;
#114282=CARTESIAN_POINT('Ctrl Pts',(60.8368805067451,249.97445637034,22.6766177015196)) ;
#114283=CARTESIAN_POINT('Ctrl Pts',(60.8341419203419,249.960288344394,22.6104152196129)) ;
#114284=CARTESIAN_POINT('Ctrl Pts',(60.8314053936341,249.946130974243,22.5442625286998)) ;
#114285=CARTESIAN_POINT('Ctrl Pts',(60.8286688669262,249.928536341561,22.478776215336)) ;
#114286=CARTESIAN_POINT('Ctrl Pts',(60.8259323402184,249.907592640746,22.414344121084)) ;
#114287=CARTESIAN_POINT('Ctrl Pts',(60.8231968585997,249.886656938403,22.3499366336765)) ;
#114288=CARTESIAN_POINT('Ctrl Pts',(60.8204613769811,249.862374861438,22.2865830523612)) ;
#114289=CARTESIAN_POINT('Ctrl Pts',(60.8177258953625,249.834884627419,22.2246566568309)) ;
#114290=CARTESIAN_POINT('Ctrl Pts',(60.8149904459441,249.807394716997,22.1627309902567)) ;
#114291=CARTESIAN_POINT('Ctrl Pts',(60.8122549965257,249.776696934551,22.1022329415506)) ;
#114292=CARTESIAN_POINT('Ctrl Pts',(60.8095195471073,249.742977034958,22.0435144614604)) ;
#114293=CARTESIAN_POINT('Ctrl Pts',(60.8067813717529,249.709223532737,21.9847374671022)) ;
#114294=CARTESIAN_POINT('Ctrl Pts',(60.8040431963985,249.672442161198,21.9277440220705)) ;
#114295=CARTESIAN_POINT('Ctrl Pts',(60.8013050210441,249.632863245043,21.8728590149956)) ;
#114296=CARTESIAN_POINT('Ctrl Pts',(60.7985652476696,249.593261230329,21.8179419766104)) ;
#114297=CARTESIAN_POINT('Ctrl Pts',(60.7958254742951,249.550858746639,21.765136218727)) ;
#114298=CARTESIAN_POINT('Ctrl Pts',(60.7930857009206,249.50592592897,21.7147329537355)) ;
#114299=CARTESIAN_POINT('Ctrl Pts',(60.7903413487892,249.460918018793,21.6642454539302)) ;
#114300=CARTESIAN_POINT('Ctrl Pts',(60.7875969966577,249.413371702513,21.6161688131355)) ;
#114301=CARTESIAN_POINT('Ctrl Pts',(60.7848526445263,249.36359248379,21.570756003064)) ;
#114302=CARTESIAN_POINT('Ctrl Pts',(60.7839071682894,249.346442691731,21.5551105134491)) ;
#114303=CARTESIAN_POINT('Ctrl Pts',(60.7829616920525,249.329028140442,21.5397808315764)) ;
#114304=CARTESIAN_POINT('Ctrl Pts',(60.7820162158156,249.311362119412,21.5247761119928)) ;
#114305=CARTESIAN_POINT('Ctrl Pts',(60.7792207997854,249.259130369472,21.4804128249879)) ;
#114306=CARTESIAN_POINT('Ctrl Pts',(60.7764253837552,249.204468501124,21.4386982606199)) ;
#114307=CARTESIAN_POINT('Ctrl Pts',(60.773629967725,249.14767608081,21.3999094805068)) ;
#114308=CARTESIAN_POINT('Ctrl Pts',(60.7708388225159,249.090970427642,21.3611799616775)) ;
#114309=CARTESIAN_POINT('Ctrl Pts',(60.7680476773068,249.032141085041,21.3253676305957)) ;
#114310=CARTESIAN_POINT('Ctrl Pts',(60.7652565320977,248.971521162682,21.2927098003142)) ;
#114311=CARTESIAN_POINT('Ctrl Pts',(60.7624687690074,248.910974695395,21.2600915425557)) ;
#114312=CARTESIAN_POINT('Ctrl Pts',(60.759681005917,248.848642388168,21.2306204256485)) ;
#114313=CARTESIAN_POINT('Ctrl Pts',(60.7568932428266,248.784885296644,21.2044898549489)) ;
#114314=CARTESIAN_POINT('Ctrl Pts',(60.7541072886962,248.721169576652,21.1783762401944)) ;
#114315=CARTESIAN_POINT('Ctrl Pts',(60.7513213345658,248.656031359958,21.1555990575248)) ;
#114316=CARTESIAN_POINT('Ctrl Pts',(60.7485353804355,248.589853819179,21.1363045615809)) ;
#114317=CARTESIAN_POINT('Ctrl Pts',(60.7457502803917,248.523696566371,21.1170159807276)) ;
#114318=CARTESIAN_POINT('Ctrl Pts',(60.742965180348,248.456501093471,21.1012081045428)) ;
#114319=CARTESIAN_POINT('Ctrl Pts',(60.7401800803043,248.388666233287,21.0889774894704)) ;
#114320=CARTESIAN_POINT('Ctrl Pts',(60.73739488071,248.320828948416,21.0767464372273)) ;
#114321=CARTESIAN_POINT('Ctrl Pts',(60.7346096811158,248.252352714911,21.0680929846255)) ;
#114322=CARTESIAN_POINT('Ctrl Pts',(60.7318244815215,248.183645280938,21.0630623483131)) ;
#114323=CARTESIAN_POINT('Ctrl Pts',(60.7290364322837,248.114867549779,21.0580265649656)) ;
#114324=CARTESIAN_POINT('Ctrl Pts',(60.7262483830459,248.045858637042,21.0566210313713)) ;
#114325=CARTESIAN_POINT('Ctrl Pts',(60.7234603338081,247.97702909406,21.0588388897445)) ;
#114326=CARTESIAN_POINT('Ctrl Pts',(60.7206706740539,247.9081597917,21.0610580292635)) ;
#114327=CARTESIAN_POINT('Ctrl Pts',(60.7178810142997,247.839470555038,21.0669046851393)) ;
#114328=CARTESIAN_POINT('Ctrl Pts',(60.7150913545455,247.77136682293,21.0763200961557)) ;
#114329=CARTESIAN_POINT('Ctrl Pts',(60.7122970046519,247.703148590836,21.0857513369128)) ;
#114330=CARTESIAN_POINT('Ctrl Pts',(60.7095026547583,247.635518310246,21.098763215029)) ;
#114331=CARTESIAN_POINT('Ctrl Pts',(60.7067083048646,247.56887036202,21.1152460418431)) ;
#114332=CARTESIAN_POINT('Ctrl Pts',(60.7054361265197,247.538527677785,21.12275014696)) ;
#114333=CARTESIAN_POINT('Ctrl Pts',(60.7041639481749,247.508388377401,21.1309729915753)) ;
#114334=CARTESIAN_POINT('Ctrl Pts',(60.70289176983,247.4784883761,21.1399008917264)) ;
#114335=CARTESIAN_POINT('Ctrl Pts',(60.7000915271226,247.4126742857,21.1595524503236)) ;
#114336=CARTESIAN_POINT('Ctrl Pts',(60.6972912844152,247.347767441634,21.1826988792258)) ;
#114337=CARTESIAN_POINT('Ctrl Pts',(60.6944910417078,247.284164349133,21.2092375935824)) ;
#114338=CARTESIAN_POINT('Ctrl Pts',(60.6916949036419,247.220654487084,21.2357374070584)) ;
#114339=CARTESIAN_POINT('Ctrl Pts',(60.688898765576,247.15844503129,21.2656194488466)) ;
#114340=CARTESIAN_POINT('Ctrl Pts',(60.68610262751,247.09791714036,21.2987314319828)) ;
#114341=CARTESIAN_POINT('Ctrl Pts',(60.6833096520937,247.037457711181,21.331805962891)) ;
#114342=CARTESIAN_POINT('Ctrl Pts',(60.6805166766774,246.9786764964,21.3681029451052)) ;
#114343=CARTESIAN_POINT('Ctrl Pts',(60.6777237012611,246.921932836441,21.4074228310548)) ;
#114344=CARTESIAN_POINT('Ctrl Pts',(60.6749324018922,246.865223228005,21.4467191213821)) ;
#114345=CARTESIAN_POINT('Ctrl Pts',(60.6721411025233,246.810549149747,21.4890344383072)) ;
#114346=CARTESIAN_POINT('Ctrl Pts',(60.6693498031544,246.758242239952,21.5341251255906)) ;
#114347=CARTESIAN_POINT('Ctrl Pts',(60.6665592337996,246.705949010089,21.5792040202154)) ;
#114348=CARTESIAN_POINT('Ctrl Pts',(60.6637686644449,246.656022089808,21.6270565246742)) ;
#114349=CARTESIAN_POINT('Ctrl Pts',(60.6609780950902,246.608759804541,21.6773989110412)) ;
#114350=CARTESIAN_POINT('Ctrl Pts',(60.6581873108187,246.561493879352,21.7277451745457)) ;
#114351=CARTESIAN_POINT('Ctrl Pts',(60.6553965265472,246.516893329597,21.7805813422929)) ;
#114352=CARTESIAN_POINT('Ctrl Pts',(60.6526057422757,246.475218158088,21.8355883775404)) ;
#114353=CARTESIAN_POINT('Ctrl Pts',(60.6498119735595,246.433498419448,21.8906542369183)) ;
#114354=CARTESIAN_POINT('Ctrl Pts',(60.6470182048433,246.394710598093,21.9478952060108)) ;
#114355=CARTESIAN_POINT('Ctrl Pts',(60.6442244361271,246.359072471378,22.0069616450271)) ;
#114356=CARTESIAN_POINT('Ctrl Pts',(60.6414289717839,246.323412714753,22.0660639333415)) ;
#114357=CARTESIAN_POINT('Ctrl Pts',(60.6386335074407,246.290906688001,22.1269934651638)) ;
#114358=CARTESIAN_POINT('Ctrl Pts',(60.6358380430975,246.261725797918,22.189376731736)) ;
#114359=CARTESIAN_POINT('Ctrl Pts',(60.6330378190237,246.232495222646,22.2518662159187)) ;
#114360=CARTESIAN_POINT('Ctrl Pts',(60.6302375949499,246.206601267018,22.3158139217921)) ;
#114361=CARTESIAN_POINT('Ctrl Pts',(60.6274373708761,246.184166573019,22.3808279710544)) ;
#114362=CARTESIAN_POINT('Ctrl Pts',(60.6262140218656,246.17436540712,22.4092310097893)) ;
#114363=CARTESIAN_POINT('Ctrl Pts',(60.624990672855,246.165223824895,22.4378374014921)) ;
#114364=CARTESIAN_POINT('Ctrl Pts',(60.6237673238445,246.156748995185,22.4666138413696)) ;
#114365=CARTESIAN_POINT('Ctrl Pts',(60.6209728463264,246.137390070716,22.5323474248334)) ;
#114366=CARTESIAN_POINT('Ctrl Pts',(60.6181783688083,246.121437928544,22.5992261940902)) ;
#114367=CARTESIAN_POINT('Ctrl Pts',(60.6153838912903,246.109023833977,22.6668638690292)) ;
#114368=CARTESIAN_POINT('Ctrl Pts',(60.6125936203238,246.096628426456,22.7343997283795)) ;
#114369=CARTESIAN_POINT('Ctrl Pts',(60.6098033493574,246.087760584623,22.8026917465618)) ;
#114370=CARTESIAN_POINT('Ctrl Pts',(60.607013078391,246.082501613517,22.871339176387)) ;
#114371=CARTESIAN_POINT('Ctrl Pts',(60.6042260913646,246.077248831826,22.9399058133263)) ;
#114372=CARTESIAN_POINT('Ctrl Pts',(60.6014391043382,246.075596522822,23.0088265433377)) ;
#114373=CARTESIAN_POINT('Ctrl Pts',(60.5986521173118,246.077574510736,23.0776929455325)) ;
#114374=CARTESIAN_POINT('Ctrl Pts',(60.5958668779608,246.079551258286,23.1465161627001)) ;
#114375=CARTESIAN_POINT('Ctrl Pts',(60.5930816386097,246.085153772792,23.2152846293504)) ;
#114376=CARTESIAN_POINT('Ctrl Pts',(60.5902963992586,246.094359805167,23.2835889143811)) ;
#114377=CARTESIAN_POINT('Ctrl Pts',(60.5875119520576,246.103563219255,23.3518737729869)) ;
#114378=CARTESIAN_POINT('Ctrl Pts',(60.5847275048566,246.116368051003,23.4196942250991)) ;
#114379=CARTESIAN_POINT('Ctrl Pts',(60.5819430576555,246.132700280669,23.4866467669927)) ;
#114380=CARTESIAN_POINT('Ctrl Pts',(60.5791584482503,246.149033461747,23.553603209116)) ;
#114381=CARTESIAN_POINT('Ctrl Pts',(60.5763738388451,246.168894329681,23.6196911636752)) ;
#114382=CARTESIAN_POINT('Ctrl Pts',(60.5735892294399,246.192158342209,23.6845198859525)) ;
#114383=CARTESIAN_POINT('Ctrl Pts',(60.5708016727571,246.215446977761,23.7494172240416)) ;
#114384=CARTESIAN_POINT('Ctrl Pts',(60.5680141160744,246.242145779759,23.8130522064917)) ;
#114385=CARTESIAN_POINT('Ctrl Pts',(60.5652265593917,246.272081496719,23.8750527182253)) ;
#114386=CARTESIAN_POINT('Ctrl Pts',(60.56243733713,246.302035100417,23.9370902755716)) ;
#114387=CARTESIAN_POINT('Ctrl Pts',(60.5596481148684,246.335229231385,23.9974909877557)) ;
#114388=CARTESIAN_POINT('Ctrl Pts',(60.5568588926067,246.371445317106,24.0559085496765)) ;
#114389=CARTESIAN_POINT('Ctrl Pts',(60.5540648918213,246.407723448592,24.1144261931551)) ;
#114390=CARTESIAN_POINT('Ctrl Pts',(60.5512708910359,246.447033586875,24.170953502343)) ;
#114391=CARTESIAN_POINT('Ctrl Pts',(60.5484768902505,246.489115146096,24.225175005198)) ;
#114392=CARTESIAN_POINT('Ctrl Pts',(60.54719888612,246.508363675582,24.2499764673062)) ;
#114393=CARTESIAN_POINT('Ctrl Pts',(60.5459208819895,246.528191518457,24.2742959840743)) ;
#114394=CARTESIAN_POINT('Ctrl Pts',(60.544642877859,246.548571183694,24.2981059507884)) ;
#114395=CARTESIAN_POINT('Ctrl Pts',(60.541846472607,246.593163999588,24.350204621192)) ;
#114396=CARTESIAN_POINT('Ctrl Pts',(60.539050067355,246.640576967329,24.4000665435235)) ;
#114397=CARTESIAN_POINT('Ctrl Pts',(60.5362536621031,246.690557083637,24.4473710087)) ;
#114398=CARTESIAN_POINT('Ctrl Pts',(60.5334614409992,246.740462416718,24.4946046941182)) ;
#114399=CARTESIAN_POINT('Ctrl Pts',(60.5306692198953,246.792926921071,24.5392881825583)) ;
#114400=CARTESIAN_POINT('Ctrl Pts',(60.5278769987914,246.847658276922,24.5811348187384)) ;
#114401=CARTESIAN_POINT('Ctrl Pts',(60.525088038235,246.902325721579,24.622932589538)) ;
#114402=CARTESIAN_POINT('Ctrl Pts',(60.5222990776787,246.959254372302,24.6618997906813)) ;
#114403=CARTESIAN_POINT('Ctrl Pts',(60.5195101171224,247.018117457038,24.6977887834864)) ;
#114404=CARTESIAN_POINT('Ctrl Pts',(60.5167228909016,247.076943937332,24.7336554584578)) ;
#114405=CARTESIAN_POINT('Ctrl Pts',(60.5139356646809,247.137702047111,24.7664474675678)) ;
#114406=CARTESIAN_POINT('Ctrl Pts',(60.5111484384601,247.200035823984,24.7959603072259)) ;
#114407=CARTESIAN_POINT('Ctrl Pts',(60.5083619941295,247.262352114596,24.8254648677579)) ;
#114408=CARTESIAN_POINT('Ctrl Pts',(60.5055755497989,247.326242751377,24.8516918751861)) ;
#114409=CARTESIAN_POINT('Ctrl Pts',(60.5027891054682,247.391328556904,24.8744834780218)) ;
#114410=CARTESIAN_POINT('Ctrl Pts',(60.500002491741,247.4564183192,24.8972764664297)) ;
#114411=CARTESIAN_POINT('Ctrl Pts',(60.4972158780138,247.522702930432,24.9166334758251)) ;
#114412=CARTESIAN_POINT('Ctrl Pts',(60.4944292642866,247.589786397934,24.9324459757382)) ;
#114413=CARTESIAN_POINT('Ctrl Pts',(60.4916397061812,247.656940746841,24.9482751833776)) ;
#114414=CARTESIAN_POINT('Ctrl Pts',(60.4888501480758,247.724895157914,24.9605522946353)) ;
#114415=CARTESIAN_POINT('Ctrl Pts',(60.4860605899705,247.793242726614,24.9692197745365)) ;
#114416=CARTESIAN_POINT('Ctrl Pts',(60.4832693650643,247.861631133963,24.9778924333808)) ;
#114417=CARTESIAN_POINT('Ctrl Pts',(60.4804781401581,247.93041267696,24.9829511322373)) ;
#114418=CARTESIAN_POINT('Ctrl Pts',(60.4776869152519,247.999177392859,24.9843904008123)) ;
#114419=CARTESIAN_POINT('Ctrl Pts',(60.4748909308483,248.068059363904,24.9858321235768)) ;
#114420=CARTESIAN_POINT('Ctrl Pts',(60.4720949464448,248.136923960343,24.9836421141915)) ;
#114421=CARTESIAN_POINT('Ctrl Pts',(60.4692989620412,248.205364171719,24.9778669310674)) ;
#114422=CARTESIAN_POINT('Ctrl Pts',(60.4680387853186,248.236210824925,24.9752640011897)) ;
#114423=CARTESIAN_POINT('Ctrl Pts',(60.4667786085961,248.266971381999,24.9719334791067)) ;
#114424=CARTESIAN_POINT('Ctrl Pts',(60.4655184318735,248.297609316392,24.9678830084377)) ;
#114425=CARTESIAN_POINT('Ctrl Pts',(60.4627217313374,248.365603849224,24.9588938299453)) ;
#114426=CARTESIAN_POINT('Ctrl Pts',(60.4599250308014,248.433259765759,24.9463201701829)) ;
#114427=CARTESIAN_POINT('Ctrl Pts',(60.4571283302653,248.500170205801,24.9301994782405)) ;
#114428=CARTESIAN_POINT('Ctrl Pts',(60.454335802507,248.566980813061,24.9141028389498)) ;
#114429=CARTESIAN_POINT('Ctrl Pts',(60.4515432747487,248.633047678172,24.8944697854931)) ;
#114430=CARTESIAN_POINT('Ctrl Pts',(60.4487507469903,248.697971081105,24.8713892889397)) ;
#114431=CARTESIAN_POINT('Ctrl Pts',(60.4459614644379,248.762819036333,24.8483356143094)) ;
#114432=CARTESIAN_POINT('Ctrl Pts',(60.4431721818855,248.826525708382,24.8218426171166)) ;
#114433=CARTESIAN_POINT('Ctrl Pts',(60.4403828993332,248.888705325434,24.7920494157437)) ;
#114434=CARTESIAN_POINT('Ctrl Pts',(60.4375953417695,248.950846488462,24.7622746395159)) ;
#114435=CARTESIAN_POINT('Ctrl Pts',(60.4348077842058,249.011462028446,24.7292039195699)) ;
#114436=CARTESIAN_POINT('Ctrl Pts',(60.4320202266421,249.070186442763,24.6930243525755)) ;
#114437=CARTESIAN_POINT('Ctrl Pts',(60.4292334421206,249.128894571694,24.6568548188564)) ;
#114438=CARTESIAN_POINT('Ctrl Pts',(60.4264466575992,249.185712198593,24.6175784069928)) ;
#114439=CARTESIAN_POINT('Ctrl Pts',(60.4236598730777,249.240300293076,24.5754270979577)) ;
#114440=CARTESIAN_POINT('Ctrl Pts',(60.4208729108012,249.294891869461,24.5332731003019)) ;
#114441=CARTESIAN_POINT('Ctrl Pts',(60.4180859485247,249.347253244298,24.4882441433253)) ;
#114442=CARTESIAN_POINT('Ctrl Pts',(60.4152989862482,249.397077582791,24.4406131807398)) ;
#114443=CARTESIAN_POINT('Ctrl Pts',(60.412509069306,249.446954743765,24.3929317210332)) ;
#114444=CARTESIAN_POINT('Ctrl Pts',(60.4097191523638,249.494289145367,24.3426430902747)) ;
#114445=CARTESIAN_POINT('Ctrl Pts',(60.4069292354216,249.538810766896,24.2900571789836)) ;
#114446=CARTESIAN_POINT('Ctrl Pts',(60.4041376452774,249.583359089459,24.237439730248)) ;
#114447=CARTESIAN_POINT('Ctrl Pts',(60.4013460551333,249.625090977645,24.1825226496002)) ;
#114448=CARTESIAN_POINT('Ctrl Pts',(60.3985544649891,249.663778400683,24.1256467616923)) ;
#114449=CARTESIAN_POINT('Ctrl Pts',(60.3957581092698,249.702531867736,24.068673779906)) ;
#114450=CARTESIAN_POINT('Ctrl Pts',(60.3929617535506,249.738230242976,24.0097357365423)) ;
#114451=CARTESIAN_POINT('Ctrl Pts',(60.3901653978313,249.770690729435,23.9491993324047)) ;
#114452=CARTESIAN_POINT('Ctrl Pts',(60.3889082605168,249.785283754383,23.9219844212257)) ;
#114453=CARTESIAN_POINT('Ctrl Pts',(60.3876511232024,249.799223023744,23.8944467542978)) ;
#114454=CARTESIAN_POINT('Ctrl Pts',(60.3863939858879,249.812495138397,23.8666208632575)) ;
#114455=CARTESIAN_POINT('Ctrl Pts',(60.3833813626935,249.844300638067,23.7999384700241)) ;
#114456=CARTESIAN_POINT('Ctrl Pts',(60.3803687394992,249.872381270698,23.7313699924473)) ;
#114457=CARTESIAN_POINT('Ctrl Pts',(60.3773561163049,249.896528208531,23.6613356174494)) ;
#114458=CARTESIAN_POINT('Ctrl Pts',(60.3743507893122,249.92061666546,23.5914708570667)) ;
#114459=CARTESIAN_POINT('Ctrl Pts',(60.3713454623195,249.940790267254,23.520147609701)) ;
#114460=CARTESIAN_POINT('Ctrl Pts',(60.3683401353268,249.956887480057,23.4478070750172)) ;
#114461=CARTESIAN_POINT('Ctrl Pts',(60.3653462472982,249.972923423175,23.3757418850056)) ;
#114462=CARTESIAN_POINT('Ctrl Pts',(60.3623523592696,249.984913803617,23.3026674779063)) ;
#114463=CARTESIAN_POINT('Ctrl Pts',(60.359358471241,249.992746915436,23.2290390013499)) ;
#114464=CARTESIAN_POINT('Ctrl Pts',(60.3565649437256,250.000055810489,23.1603379767246)) ;
#114465=CARTESIAN_POINT('Ctrl Pts',(60.3537714162101,250.003745611572,23.0911549666261)) ;
#114466=CARTESIAN_POINT('Ctrl Pts',(60.3509778886947,250.003765030662,23.0218706758452)) ;
#114467=CARTESIAN_POINT('',(59.8509778886854,250.003764316488,23.0195575538546)) ;
#114468=CARTESIAN_POINT('Ctrl Pts',(60.3509778886564,250.003765030662,23.0218706748954)) ;
#114469=CARTESIAN_POINT('Ctrl Pts',(60.3481156163826,250.003784927595,22.9508813957776)) ;
#114470=CARTESIAN_POINT('Ctrl Pts',(60.3452533441087,249.999950618947,22.8799290676602)) ;
#114471=CARTESIAN_POINT('Ctrl Pts',(60.3423910718349,249.992300212387,22.8094449075012)) ;
#114472=CARTESIAN_POINT('Ctrl Pts',(60.3394642775072,249.984477348459,22.7373718758636)) ;
#114473=CARTESIAN_POINT('Ctrl Pts',(60.3365374831795,249.972664300783,22.665788871538)) ;
#114474=CARTESIAN_POINT('Ctrl Pts',(60.3336106888518,249.956957141299,22.5951467889264)) ;
#114475=CARTESIAN_POINT('Ctrl Pts',(60.3307403892547,249.941553170779,22.5258682819477)) ;
#114476=CARTESIAN_POINT('Ctrl Pts',(60.3278700896576,249.922404298269,22.4574951094046)) ;
#114477=CARTESIAN_POINT('Ctrl Pts',(60.3249997900605,249.899651448691,22.3904362929958)) ;
#114478=CARTESIAN_POINT('Ctrl Pts',(60.3220447483675,249.876226848971,22.3213976467955)) ;
#114479=CARTESIAN_POINT('Ctrl Pts',(60.3190897066745,249.848982314889,22.253752671223)) ;
#114480=CARTESIAN_POINT('Ctrl Pts',(60.3161346649815,249.818123636963,22.1879228992188)) ;
#114481=CARTESIAN_POINT('Ctrl Pts',(60.3131796232885,249.787264959037,22.1220931272147)) ;
#114482=CARTESIAN_POINT('Ctrl Pts',(60.3102245815955,249.75279244704,22.0580789757814)) ;
#114483=CARTESIAN_POINT('Ctrl Pts',(60.3072695399025,249.7149604943,21.9962702899579)) ;
#114484=CARTESIAN_POINT('Ctrl Pts',(60.3044731809281,249.679160078756,21.9377806673909)) ;
#114485=CARTESIAN_POINT('Ctrl Pts',(60.3016768219538,249.640221610421,21.8810541208869)) ;
#114486=CARTESIAN_POINT('Ctrl Pts',(60.2988804629795,249.598344256327,21.8264472888461)) ;
#114487=CARTESIAN_POINT('Ctrl Pts',(60.2960882846115,249.556529509622,21.7719220949892)) ;
#114488=CARTESIAN_POINT('Ctrl Pts',(60.2932961062435,249.511784893843,21.7195107122991)) ;
#114489=CARTESIAN_POINT('Ctrl Pts',(60.2905039278755,249.464353777528,21.6695423622655)) ;
#114490=CARTESIAN_POINT('Ctrl Pts',(60.2877150045518,249.416977955098,21.6196322639534)) ;
#114491=CARTESIAN_POINT('Ctrl Pts',(60.2849260812282,249.366922188642,21.5721598961588)) ;
#114492=CARTESIAN_POINT('Ctrl Pts',(60.2821371579046,249.314470029272,21.5274213951497)) ;
#114493=CARTESIAN_POINT('Ctrl Pts',(60.279349965464,249.262050423165,21.4827106600924)) ;
#114494=CARTESIAN_POINT('Ctrl Pts',(60.2765627730233,249.207237747198,21.4407307436908)) ;
#114495=CARTESIAN_POINT('Ctrl Pts',(60.2737755805827,249.150351188822,21.4017397982671)) ;
#114496=CARTESIAN_POINT('Ctrl Pts',(60.2709891665113,249.093480516952,21.362759741705)) ;
#114497=CARTESIAN_POINT('Ctrl Pts',(60.2682027524399,249.034537517161,21.326767276302)) ;
#114498=CARTESIAN_POINT('Ctrl Pts',(60.2654163383685,248.973871668104,21.2939781537975)) ;
#114499=CARTESIAN_POINT('Ctrl Pts',(60.2626297513077,248.913202052718,21.2611869956402)) ;
#114500=CARTESIAN_POINT('Ctrl Pts',(60.2598431642469,248.850809808714,21.2315998063246)) ;
#114501=CARTESIAN_POINT('Ctrl Pts',(60.2570565771861,248.787068807701,21.2053862908493)) ;
#114502=CARTESIAN_POINT('Ctrl Pts',(60.2542670400896,248.723260326928,21.1791450242923)) ;
#114503=CARTESIAN_POINT('Ctrl Pts',(60.2514775029931,248.658100694404,21.1562847461771)) ;
#114504=CARTESIAN_POINT('Ctrl Pts',(60.2486879658967,248.591982610388,21.1369265292726)) ;
#114505=CARTESIAN_POINT('Ctrl Pts',(60.2458967587889,248.52582494348,21.1175567231909)) ;
#114506=CARTESIAN_POINT('Ctrl Pts',(60.2431055516812,248.458708160783,21.1016932639497)) ;
#114507=CARTESIAN_POINT('Ctrl Pts',(60.2403143445735,248.391036203635,21.0894062957001)) ;
#114508=CARTESIAN_POINT('Ctrl Pts',(60.2375183728113,248.323248728905,21.0770983533139)) ;
#114509=CARTESIAN_POINT('Ctrl Pts',(60.234722401049,248.254904674889,21.0683791485604)) ;
#114510=CARTESIAN_POINT('Ctrl Pts',(60.2319264292868,248.186413283751,21.0632669835456)) ;
#114511=CARTESIAN_POINT('Ctrl Pts',(60.2306659841635,248.155536848906,21.0609623810638)) ;
#114512=CARTESIAN_POINT('Ctrl Pts',(60.2294055390402,248.124630469464,21.0593901220682)) ;
#114513=CARTESIAN_POINT('Ctrl Pts',(60.2281450939169,248.093731443593,21.0585484258536)) ;
#114514=CARTESIAN_POINT('Ctrl Pts',(60.2253487256112,248.025180219086,21.056681075523)) ;
#114515=CARTESIAN_POINT('Ctrl Pts',(60.2225523573054,247.956396648871,21.0584056752074)) ;
#114516=CARTESIAN_POINT('Ctrl Pts',(60.2197559889997,247.887788298727,21.063749636612)) ;
#114517=CARTESIAN_POINT('Ctrl Pts',(60.2169638004718,247.819282498616,21.0690856103094)) ;
#114518=CARTESIAN_POINT('Ctrl Pts',(60.2141716119439,247.750951884224,21.0780301705784)) ;
#114519=CARTESIAN_POINT('Ctrl Pts',(60.2113794234159,247.683205127758,21.0905587268232)) ;
#114520=CARTESIAN_POINT('Ctrl Pts',(60.208590488753,247.615537319686,21.1030726829685)) ;
#114521=CARTESIAN_POINT('Ctrl Pts',(60.20580155409,247.548452498587,21.1191622511027)) ;
#114522=CARTESIAN_POINT('Ctrl Pts',(60.2030126194271,247.48235350046,21.1387511181628)) ;
#114523=CARTESIAN_POINT('Ctrl Pts',(60.2002254149202,247.416295507804,21.1583278329855)) ;
#114524=CARTESIAN_POINT('Ctrl Pts',(60.1974382104132,247.351222594435,21.1813994010614)) ;
#114525=CARTESIAN_POINT('Ctrl Pts',(60.1946510059063,247.287525174951,21.2078389282935)) ;
#114526=CARTESIAN_POINT('Ctrl Pts',(60.1918645790591,247.223845527724,21.2342710786165)) ;
#114527=CARTESIAN_POINT('Ctrl Pts',(60.1890781522118,247.16154106557,21.264069134426)) ;
#114528=CARTESIAN_POINT('Ctrl Pts',(60.1862917253646,247.10098316542,21.2970576945569)) ;
#114529=CARTESIAN_POINT('Ctrl Pts',(60.183505124835,247.040421490602,21.3300483109162)) ;
#114530=CARTESIAN_POINT('Ctrl Pts',(60.1807185243054,246.981607023702,21.3662295893756)) ;
#114531=CARTESIAN_POINT('Ctrl Pts',(60.1779319237758,246.924885832193,21.4053805793426)) ;
#114532=CARTESIAN_POINT('Ctrl Pts',(60.1751423722518,246.868104573257,21.4445730299903)) ;
#114533=CARTESIAN_POINT('Ctrl Pts',(60.1723528207277,246.813421418289,21.4867411889387)) ;
#114534=CARTESIAN_POINT('Ctrl Pts',(60.1695632692037,246.761151924879,21.5316218118715)) ;
#114535=CARTESIAN_POINT('Ctrl Pts',(60.1667720470989,246.7088511288,21.5765293124957)) ;
#114536=CARTESIAN_POINT('Ctrl Pts',(60.1639808249941,246.658967226175,21.6241521711496)) ;
#114537=CARTESIAN_POINT('Ctrl Pts',(60.1611896028893,246.611779203611,21.6741899595309)) ;
#114538=CARTESIAN_POINT('Ctrl Pts',(60.1583936154072,246.564510618226,21.7243131760609)) ;
#114539=CARTESIAN_POINT('Ctrl Pts',(60.1555976279252,246.519947415956,21.7768591767358)) ;
#114540=CARTESIAN_POINT('Ctrl Pts',(60.1528016404432,246.478328008864,21.8314948315574)) ;
#114541=CARTESIAN_POINT('Ctrl Pts',(60.1515413096059,246.459567473446,21.8561226244312)) ;
#114542=CARTESIAN_POINT('Ctrl Pts',(60.1502809787687,246.441404490081,21.8811746272296)) ;
#114543=CARTESIAN_POINT('Ctrl Pts',(60.1490206479314,246.423857890794,21.9066186081808)) ;
#114544=CARTESIAN_POINT('Ctrl Pts',(60.1462243320115,246.384926974025,21.9630715702901)) ;
#114545=CARTESIAN_POINT('Ctrl Pts',(60.1434280160915,246.348880673387,22.0216771985092)) ;
#114546=CARTESIAN_POINT('Ctrl Pts',(60.1406317001716,246.315964132663,22.0821087608005)) ;
#114547=CARTESIAN_POINT('Ctrl Pts',(60.1378395650777,246.283096806096,22.1424499706933)) ;
#114548=CARTESIAN_POINT('Ctrl Pts',(60.1350474299839,246.253350185016,22.2046112686915)) ;
#114549=CARTESIAN_POINT('Ctrl Pts',(60.13225529489,246.226926419963,22.2682366475178)) ;
#114550=CARTESIAN_POINT('Ctrl Pts',(60.129466414945,246.200533460472,22.3317878501041)) ;
#114551=CARTESIAN_POINT('Ctrl Pts',(60.126677535,246.177455850471,22.3967992923198)) ;
#114552=CARTESIAN_POINT('Ctrl Pts',(60.1238886550551,246.157849197065,22.4628916649776)) ;
#114553=CARTESIAN_POINT('Ctrl Pts',(60.1211015060306,246.138254712543,22.528943017354)) ;
#114554=CARTESIAN_POINT('Ctrl Pts',(60.118314357006,246.122127050301,22.5960734997507)) ;
#114555=CARTESIAN_POINT('Ctrl Pts',(60.1155272079815,246.109572641203,22.6638866441411)) ;
#114556=CARTESIAN_POINT('Ctrl Pts',(60.1127408372949,246.097021738043,22.7316808510648)) ;
#114557=CARTESIAN_POINT('Ctrl Pts',(60.1099544666084,246.088042196262,22.80015685909)) ;
#114558=CARTESIAN_POINT('Ctrl Pts',(60.1071680959218,246.082689402512,22.8689077190084)) ;
#114559=CARTESIAN_POINT('Ctrl Pts',(60.1043815521456,246.077336276246,22.9376628497352)) ;
#114560=CARTESIAN_POINT('Ctrl Pts',(60.1015950083695,246.075610380834,23.0066923767052)) ;
#114561=CARTESIAN_POINT('Ctrl Pts',(60.0988084645933,246.077515119444,23.0755857401096)) ;
#114562=CARTESIAN_POINT('Ctrl Pts',(60.0960189703294,246.079421874856,23.1445520501628)) ;
#114563=CARTESIAN_POINT('Ctrl Pts',(60.0932294760654,246.084966922447,23.2133814173607)) ;
#114564=CARTESIAN_POINT('Ctrl Pts',(60.0904399818014,246.094101576605,23.2816658061659)) ;
#114565=CARTESIAN_POINT('Ctrl Pts',(60.0876488173283,246.103241700135,23.3499910802353)) ;
#114566=CARTESIAN_POINT('Ctrl Pts',(60.0848576528552,246.115975617192,23.4177702440408)) ;
#114567=CARTESIAN_POINT('Ctrl Pts',(60.0820664883821,246.132203533377,23.4846056533459)) ;
#114568=CARTESIAN_POINT('Ctrl Pts',(60.0792705585032,246.148459155778,23.5515551719592)) ;
#114569=CARTESIAN_POINT('Ctrl Pts',(60.0764746286243,246.168220542193,23.6175572503759)) ;
#114570=CARTESIAN_POINT('Ctrl Pts',(60.0736786987453,246.19133836498,23.6822304355829)) ;
#114571=CARTESIAN_POINT('Ctrl Pts',(60.0724178664789,246.20176341073,23.7113949862754)) ;
#114572=CARTESIAN_POINT('Ctrl Pts',(60.0711570342124,246.212870371109,23.7402895834809)) ;
#114573=CARTESIAN_POINT('Ctrl Pts',(60.0698962019459,246.224642467898,23.7688808290893)) ;
#114574=CARTESIAN_POINT('Ctrl Pts',(60.0670998615051,246.250751246359,23.8322920047631)) ;
#114575=CARTESIAN_POINT('Ctrl Pts',(60.0643035210644,246.280237194779,23.8944581076416)) ;
#114576=CARTESIAN_POINT('Ctrl Pts',(60.0615071806236,246.312960002354,23.9549955133845)) ;
#114577=CARTESIAN_POINT('Ctrl Pts',(60.0587150206563,246.345633889981,24.0154424169087)) ;
#114578=CARTESIAN_POINT('Ctrl Pts',(60.0559228606889,246.38153480094,24.0742650275334)) ;
#114579=CARTESIAN_POINT('Ctrl Pts',(60.0531307007216,246.420474446045,24.1310998091008)) ;
#114580=CARTESIAN_POINT('Ctrl Pts',(60.0503417955066,246.459368700161,24.187868339758)) ;
#114581=CARTESIAN_POINT('Ctrl Pts',(60.0475528902916,246.501294377167,24.2426532404599)) ;
#114582=CARTESIAN_POINT('Ctrl Pts',(60.0447639850766,246.546018282303,24.2951172954059)) ;
#114583=CARTESIAN_POINT('Ctrl Pts',(60.0419768105513,246.590714433464,24.3475487931324)) ;
#114584=CARTESIAN_POINT('Ctrl Pts',(60.039189636026,246.638205050219,24.3976619295297)) ;
#114585=CARTESIAN_POINT('Ctrl Pts',(60.0364024615007,246.688215747403,24.4451513648145)) ;
#114586=CARTESIAN_POINT('Ctrl Pts',(60.0336160651225,246.738212482176,24.4926275415953)) ;
#114587=CARTESIAN_POINT('Ctrl Pts',(60.0308296687442,246.790727544799,24.5374811336974)) ;
#114588=CARTESIAN_POINT('Ctrl Pts',(60.028043272366,246.845449939911,24.5794438831465)) ;
#114589=CARTESIAN_POINT('Ctrl Pts',(60.025256702747,246.900175737319,24.6214092415769)) ;
#114590=CARTESIAN_POINT('Ctrl Pts',(60.0224701331281,246.957108748631,24.6604831038896)) ;
#114591=CARTESIAN_POINT('Ctrl Pts',(60.0196835635092,247.015906616421,24.6964388262848)) ;
#114592=CARTESIAN_POINT('Ctrl Pts',(60.0168940433521,247.074766741887,24.7324326201246)) ;
#114593=CARTESIAN_POINT('Ctrl Pts',(60.014104523195,247.135495244891,24.7653014286367)) ;
#114594=CARTESIAN_POINT('Ctrl Pts',(60.0113150030379,247.197723491837,24.7948636543907)) ;
#114595=CARTESIAN_POINT('Ctrl Pts',(60.0085238126059,247.259988999052,24.8244435810532)) ;
#114596=CARTESIAN_POINT('Ctrl Pts',(60.005732622174,247.323755583584,24.8507127975332)) ;
#114597=CARTESIAN_POINT('Ctrl Pts',(60.0029414317421,247.388635465295,24.8735382192499)) ;
#114598=CARTESIAN_POINT('Ctrl Pts',(60.0001454760743,247.453626112625,24.8964026094713)) ;
#114599=CARTESIAN_POINT('Ctrl Pts',(59.9973495204066,247.519733379805,24.9158113327619)) ;
#114600=CARTESIAN_POINT('Ctrl Pts',(59.9945535647388,247.58655606146,24.9316816578878)) ;
#114601=CARTESIAN_POINT('Ctrl Pts',(59.9932929618127,247.616684174362,24.9388370568535)) ;
#114602=CARTESIAN_POINT('Ctrl Pts',(59.9920323588865,247.646957607263,24.9452738653652)) ;
#114603=CARTESIAN_POINT('Ctrl Pts',(59.9907717559603,247.677339235002,24.950987947284)) ;
#114604=CARTESIAN_POINT('Ctrl Pts',(59.9879754166289,247.744733446798,24.9636632407334)) ;
#114605=CARTESIAN_POINT('Ctrl Pts',(59.9851790772975,247.812924652615,24.972828510126)) ;
#114606=CARTESIAN_POINT('Ctrl Pts',(59.9823827379661,247.881514747908,24.9783922822575)) ;
#114607=CARTESIAN_POINT('Ctrl Pts',(59.9795905790604,247.950002303501,24.9839477367518)) ;
#114608=CARTESIAN_POINT('Ctrl Pts',(59.9767984201546,248.018887079666,24.9859123407111)) ;
#114609=CARTESIAN_POINT('Ctrl Pts',(59.9740062612489,248.087761661209,24.9842457948727)) ;
#114610=CARTESIAN_POINT('Ctrl Pts',(59.9712173570191,248.156555959199,24.9825811916411)) ;
#114611=CARTESIAN_POINT('Ctrl Pts',(59.9684284527892,248.22533959777,24.9772938568956)) ;
#114612=CARTESIAN_POINT('Ctrl Pts',(59.9656395485594,248.293702750956,24.9683954861837)) ;
#114613=CARTESIAN_POINT('Ctrl Pts',(59.962852374971,248.362023481706,24.9595026373141)) ;
#114614=CARTESIAN_POINT('Ctrl Pts',(59.9600652013827,248.429923759056,24.9470032610149)) ;
#114615=CARTESIAN_POINT('Ctrl Pts',(59.9572780277943,248.496998029126,24.9309609612058)) ;
#114616=CARTESIAN_POINT('Ctrl Pts',(59.9544916323032,248.564053574025,24.914923139937)) ;
#114617=CARTESIAN_POINT('Ctrl Pts',(59.9517052368121,248.630283092308,24.895344472913)) ;
#114618=CARTESIAN_POINT('Ctrl Pts',(59.948918841321,248.695292163224,24.8723394700529)) ;
#114619=CARTESIAN_POINT('Ctrl Pts',(59.9461322725377,248.760305277201,24.84933303646)) ;
#114620=CARTESIAN_POINT('Ctrl Pts',(59.9433457037544,248.824097331273,24.8229000101322)) ;
#114621=CARTESIAN_POINT('Ctrl Pts',(59.9405591349711,248.886291698344,24.793203877562)) ;
#114622=CARTESIAN_POINT('Ctrl Pts',(59.9377696155656,248.948551921344,24.7634763005621)) ;
#114623=CARTESIAN_POINT('Ctrl Pts',(59.9349800961602,249.009210637454,24.7304789338125)) ;
#114624=CARTESIAN_POINT('Ctrl Pts',(59.9321905767547,249.067914662949,24.6944218472864)) ;
#114625=CARTESIAN_POINT('Ctrl Pts',(59.9293993870275,249.126653839523,24.6583431703248)) ;
#114626=CARTESIAN_POINT('Ctrl Pts',(59.9266081973002,249.183435591863,24.6192014058172)) ;
#114627=CARTESIAN_POINT('Ctrl Pts',(59.9238170075729,249.23793697211,24.5772491193738)) ;
#114628=CARTESIAN_POINT('Ctrl Pts',(59.9210210525298,249.292531400955,24.53522520903)) ;
#114629=CARTESIAN_POINT('Ctrl Pts',(59.9182250974867,249.344837315308,24.4903815196029)) ;
#114630=CARTESIAN_POINT('Ctrl Pts',(59.9154291424436,249.394566664796,24.4430093189264)) ;
#114631=CARTESIAN_POINT('Ctrl Pts',(59.9141685316206,249.416988111212,24.4216506389915)) ;
#114632=CARTESIAN_POINT('Ctrl Pts',(59.9129079207977,249.43888630985,24.399778427292)) ;
#114633=CARTESIAN_POINT('Ctrl Pts',(59.9116473099748,249.460237556318,24.3774215549041)) ;
#114634=CARTESIAN_POINT('Ctrl Pts',(59.9088873770359,249.506983155628,24.3284742768134)) ;
#114635=CARTESIAN_POINT('Ctrl Pts',(59.9061274440971,249.551298080798,24.2769988443449)) ;
#114636=CARTESIAN_POINT('Ctrl Pts',(59.9033675111582,249.592892025422,24.2232695540639)) ;
#114637=CARTESIAN_POINT('Ctrl Pts',(59.900611316268,249.634429635276,24.1696130346455)) ;
#114638=CARTESIAN_POINT('Ctrl Pts',(59.8978551213778,249.673253261259,24.1137091011783)) ;
#114639=CARTESIAN_POINT('Ctrl Pts',(59.8950989264875,249.709109865646,24.0558682758293)) ;
#114640=CARTESIAN_POINT('Ctrl Pts',(59.8923454648814,249.744930911485,23.9980848105057)) ;
#114641=CARTESIAN_POINT('Ctrl Pts',(59.8895920032753,249.77779050426,23.9383686876626)) ;
#114642=CARTESIAN_POINT('Ctrl Pts',(59.8868385416692,249.807477523031,23.8770612677907)) ;
#114643=CARTESIAN_POINT('Ctrl Pts',(59.8840868124706,249.83714586349,23.8157924209773)) ;
#114644=CARTESIAN_POINT('Ctrl Pts',(59.881335083272,249.863645370605,23.7529347165331)) ;
#114645=CARTESIAN_POINT('Ctrl Pts',(59.8785833540734,249.886810688586,23.6888543636881)) ;
#114646=CARTESIAN_POINT('Ctrl Pts',(59.8758314591609,249.909977401622,23.6247701518134)) ;
#114647=CARTESIAN_POINT('Ctrl Pts',(59.8730795642484,249.929809339602,23.5594636142436)) ;
#114648=CARTESIAN_POINT('Ctrl Pts',(59.870327669336,249.94618977602,23.4933197175161)) ;
#114649=CARTESIAN_POINT('Ctrl Pts',(59.8675756586827,249.962570901377,23.427173038871)) ;
#114650=CARTESIAN_POINT('Ctrl Pts',(59.8648236480295,249.975500126689,23.360189423837)) ;
#114651=CARTESIAN_POINT('Ctrl Pts',(59.8620716373762,249.984911569834,23.292765342855)) ;
#114652=CARTESIAN_POINT('Ctrl Pts',(59.8593172440457,249.994331161361,23.2252828864359)) ;
#114653=CARTESIAN_POINT('Ctrl Pts',(59.8565628507152,250.000226840174,23.1573597050943)) ;
#114654=CARTESIAN_POINT('Ctrl Pts',(59.8538084573847,250.002584597775,23.0893972795253)) ;
#114655=CARTESIAN_POINT('Ctrl Pts',(59.8528649344849,250.003392252319,23.0661166158163)) ;
#114656=CARTESIAN_POINT('Ctrl Pts',(59.8519214115852,250.003785211226,23.0428313468794)) ;
#114657=CARTESIAN_POINT('Ctrl Pts',(59.8509778886854,250.003764316488,23.0195575538546)) ;
#114658=CARTESIAN_POINT('',(59.3509778886203,250.003764873166,23.0222802139838)) ;
#114659=CARTESIAN_POINT('Ctrl Pts',(59.8509778886564,250.003764316487,23.0195575531404)) ;
#114660=CARTESIAN_POINT('Ctrl Pts',(59.8472606717211,250.003681997014,22.927865303171)) ;
#114661=CARTESIAN_POINT('Ctrl Pts',(59.8435434547858,249.997173150939,22.8364543306825)) ;
#114662=CARTESIAN_POINT('Ctrl Pts',(59.8398262378505,249.984377212935,22.7460743215828)) ;
#114663=CARTESIAN_POINT('Ctrl Pts',(59.8373917798968,249.975996972128,22.6868831751301)) ;
#114664=CARTESIAN_POINT('Ctrl Pts',(59.834957321943,249.964921092644,22.6281335842206)) ;
#114665=CARTESIAN_POINT('Ctrl Pts',(59.8325228639892,249.951199394586,22.570030634469)) ;
#114666=CARTESIAN_POINT('Ctrl Pts',(59.8297265267532,249.935437982417,22.5032907502732)) ;
#114667=CARTESIAN_POINT('Ctrl Pts',(59.8269301895171,249.916145102473,22.4372466801222)) ;
#114668=CARTESIAN_POINT('Ctrl Pts',(59.8241338522811,249.893398687161,22.3722993986017)) ;
#114669=CARTESIAN_POINT('Ctrl Pts',(59.8213416955306,249.870686277425,22.3074492123683)) ;
#114670=CARTESIAN_POINT('Ctrl Pts',(59.81854953878,249.844530740505,22.2436930199796)) ;
#114671=CARTESIAN_POINT('Ctrl Pts',(59.8157573820295,249.815060558569,22.1814195411551)) ;
#114672=CARTESIAN_POINT('Ctrl Pts',(59.8129684800327,249.785624729356,22.1192186531119)) ;
#114673=CARTESIAN_POINT('Ctrl Pts',(59.8101795780359,249.752882138021,22.0584974875127)) ;
#114674=CARTESIAN_POINT('Ctrl Pts',(59.8073906760391,249.717009767016,21.9996258697832)) ;
#114675=CARTESIAN_POINT('Ctrl Pts',(59.8046035047309,249.681159657066,21.9407907855831)) ;
#114676=CARTESIAN_POINT('Ctrl Pts',(59.8018163334226,249.642183875268,21.8838033905476)) ;
#114677=CARTESIAN_POINT('Ctrl Pts',(59.7990291621144,249.600305113683,21.8290085428969)) ;
#114678=CARTESIAN_POINT('Ctrl Pts',(59.7962427689469,249.558438044086,21.7742289932315)) ;
#114679=CARTESIAN_POINT('Ctrl Pts',(59.7934563757794,249.513669901657,21.7216411654736)) ;
#114680=CARTESIAN_POINT('Ctrl Pts',(59.790669982612,249.46626538794,21.6715590865221)) ;
#114681=CARTESIAN_POINT('Ctrl Pts',(59.7878834161924,249.41885792671,21.6214738935717)) ;
#114682=CARTESIAN_POINT('Ctrl Pts',(59.7850968497728,249.368814108016,21.5738951134417)) ;
#114683=CARTESIAN_POINT('Ctrl Pts',(59.7823102833533,249.316436176817,21.5291006370254)) ;
#114684=CARTESIAN_POINT('Ctrl Pts',(59.7795207663561,249.264002784835,21.4842587296273)) ;
#114685=CARTESIAN_POINT('Ctrl Pts',(59.7767312493589,249.209230721837,21.4422073290829)) ;
#114686=CARTESIAN_POINT('Ctrl Pts',(59.7739417323616,249.152455296489,21.4031839975887)) ;
#114687=CARTESIAN_POINT('Ctrl Pts',(59.7711505450715,249.095645875438,21.3641372999007)) ;
#114688=CARTESIAN_POINT('Ctrl Pts',(59.7683593577814,249.036831123228,21.3281225361919)) ;
#114689=CARTESIAN_POINT('Ctrl Pts',(59.7655681704912,248.976372919869,21.2953323904856)) ;
#114690=CARTESIAN_POINT('Ctrl Pts',(59.7627722179044,248.915811498329,21.2624862633075)) ;
#114691=CARTESIAN_POINT('Ctrl Pts',(59.7599762653176,248.853601468761,21.2328759522848)) ;
#114692=CARTESIAN_POINT('Ctrl Pts',(59.7571803127307,248.790125923892,21.2066465418893)) ;
#114693=CARTESIAN_POINT('Ctrl Pts',(59.7559196811551,248.761506241098,21.1948202959398)) ;
#114694=CARTESIAN_POINT('Ctrl Pts',(59.7546590495795,248.732629510017,21.1836806831018)) ;
#114695=CARTESIAN_POINT('Ctrl Pts',(59.7533984180038,248.703531738422,21.1732376542069)) ;
#114696=CARTESIAN_POINT('Ctrl Pts',(59.7506020810814,248.638986970034,21.1500728946966)) ;
#114697=CARTESIAN_POINT('Ctrl Pts',(59.747805744159,248.573100613088,21.1302481286367)) ;
#114698=CARTESIAN_POINT('Ctrl Pts',(59.7450094072366,248.506251316868,21.1139165837474)) ;
#114699=CARTESIAN_POINT('Ctrl Pts',(59.7422172507985,248.439501959404,21.0976094542878)) ;
#114700=CARTESIAN_POINT('Ctrl Pts',(59.7394250943605,248.371792992903,21.0847852965818)) ;
#114701=CARTESIAN_POINT('Ctrl Pts',(59.7366329379224,248.303520346263,21.0755482784363)) ;
#114702=CARTESIAN_POINT('Ctrl Pts',(59.7338440362348,248.235327283426,21.0663220276634)) ;
#114703=CARTESIAN_POINT('Ctrl Pts',(59.7310551345472,248.166572329588,21.0606746771768)) ;
#114704=CARTESIAN_POINT('Ctrl Pts',(59.7282662328596,248.09766200975,21.0586594340684)) ;
#114705=CARTESIAN_POINT('Ctrl Pts',(59.7254790618583,248.028794453035,21.0566454415431)) ;
#114706=CARTESIAN_POINT('Ctrl Pts',(59.7226918908569,247.959772211123,21.05825909933)) ;
#114707=CARTESIAN_POINT('Ctrl Pts',(59.7199047198556,247.891005792548,21.0635016832096)) ;
#114708=CARTESIAN_POINT('Ctrl Pts',(59.7171183269923,247.822258572568,21.0687428034351)) ;
#114709=CARTESIAN_POINT('Ctrl Pts',(59.714331934129,247.753767523312,21.0776108010505)) ;
#114710=CARTESIAN_POINT('Ctrl Pts',(59.7115455412657,247.685940203597,21.0900549262046)) ;
#114711=CARTESIAN_POINT('Ctrl Pts',(59.7087589751471,247.618108666442,21.102499825123)) ;
#114712=CARTESIAN_POINT('Ctrl Pts',(59.7059724090285,247.550941423062,21.1185212019422)) ;
#114713=CARTESIAN_POINT('Ctrl Pts',(59.7031858429099,247.484836200829,21.1380171339526)) ;
#114714=CARTESIAN_POINT('Ctrl Pts',(59.7003963262066,247.41866098239,21.1575337094343)) ;
#114715=CARTESIAN_POINT('Ctrl Pts',(59.6976068095033,247.353550500928,21.1805320431269)) ;
#114716=CARTESIAN_POINT('Ctrl Pts',(59.6948172928,247.289886695475,21.206860509797)) ;
#114717=CARTESIAN_POINT('Ctrl Pts',(59.6920261058002,247.226184769644,21.2332047413293)) ;
#114718=CARTESIAN_POINT('Ctrl Pts',(59.6892349188004,247.163931686943,21.2628828631704)) ;
#114719=CARTESIAN_POINT('Ctrl Pts',(59.6864437318006,247.103486244982,21.2956965107952)) ;
#114720=CARTESIAN_POINT('Ctrl Pts',(59.6836477794956,247.042937606431,21.3285661801224)) ;
#114721=CARTESIAN_POINT('Ctrl Pts',(59.6808518271905,246.984203186022,21.3645818026171)) ;
#114722=CARTESIAN_POINT('Ctrl Pts',(59.6780558748854,246.927613437489,21.4035012836564)) ;
#114723=CARTESIAN_POINT('Ctrl Pts',(59.6767952405964,246.902098346519,21.4210492340356)) ;
#114724=CARTESIAN_POINT('Ctrl Pts',(59.6755346063073,246.877018804996,21.4391869641399)) ;
#114725=CARTESIAN_POINT('Ctrl Pts',(59.6742739720182,246.852402782949,21.4578897095906)) ;
#114726=CARTESIAN_POINT('Ctrl Pts',(59.6714776355049,246.797799571012,21.4993761029525)) ;
#114727=CARTESIAN_POINT('Ctrl Pts',(59.6686812989916,246.745265268268,21.5438078353552)) ;
#114728=CARTESIAN_POINT('Ctrl Pts',(59.6658849624783,246.695134733625,21.5909509763994)) ;
#114729=CARTESIAN_POINT('Ctrl Pts',(59.6630928064587,246.645079143604,21.6380236389441)) ;
#114730=CARTESIAN_POINT('Ctrl Pts',(59.6603006504391,246.597420544006,21.6877993313116)) ;
#114731=CARTESIAN_POINT('Ctrl Pts',(59.6575084944194,246.552462081674,21.740002894411)) ;
#114732=CARTESIAN_POINT('Ctrl Pts',(59.654719593162,246.507556026551,21.7921456048284)) ;
#114733=CARTESIAN_POINT('Ctrl Pts',(59.6519306919045,246.465344176247,21.8467101948815)) ;
#114734=CARTESIAN_POINT('Ctrl Pts',(59.6491417906471,246.426092728863,21.9033848440245)) ;
#114735=CARTESIAN_POINT('Ctrl Pts',(59.6463546200829,246.386865639535,21.9600243228888)) ;
#114736=CARTESIAN_POINT('Ctrl Pts',(59.6435674495187,246.350595587487,22.0187708605839)) ;
#114737=CARTESIAN_POINT('Ctrl Pts',(59.6407802789545,246.317507403936,22.0792809899092)) ;
#114738=CARTESIAN_POINT('Ctrl Pts',(59.6379938865347,246.284428458207,22.1397742255368)) ;
#114739=CARTESIAN_POINT('Ctrl Pts',(59.6352074941149,246.254529852721,22.202029644829)) ;
#114740=CARTESIAN_POINT('Ctrl Pts',(59.6324211016952,246.227991193536,22.2656778952236)) ;
#114741=CARTESIAN_POINT('Ctrl Pts',(59.6296345360257,246.201450884255,22.3293301030789)) ;
#114742=CARTESIAN_POINT('Ctrl Pts',(59.6268479703562,246.178271122553,22.3943748599644)) ;
#114743=CARTESIAN_POINT('Ctrl Pts',(59.6240614046867,246.158583253151,22.4604231623084)) ;
#114744=CARTESIAN_POINT('Ctrl Pts',(59.6212718884381,246.138874537077,22.5265414004688)) ;
#114745=CARTESIAN_POINT('Ctrl Pts',(59.6184823721895,246.122665232523,22.5936648334317)) ;
#114746=CARTESIAN_POINT('Ctrl Pts',(59.6156928559408,246.110036408564,22.6613906022208)) ;
#114747=CARTESIAN_POINT('Ctrl Pts',(59.6129016693994,246.097400022781,22.7291569235108)) ;
#114748=CARTESIAN_POINT('Ctrl Pts',(59.6101104828581,246.088348448924,22.7975258118115)) ;
#114749=CARTESIAN_POINT('Ctrl Pts',(59.6073192963167,246.082910956697,22.8660883326423)) ;
#114750=CARTESIAN_POINT('Ctrl Pts',(59.6045233444711,246.077464181212,22.9347679080891)) ;
#114751=CARTESIAN_POINT('Ctrl Pts',(59.6017273926255,246.075643814714,23.0036412854946)) ;
#114752=CARTESIAN_POINT('Ctrl Pts',(59.5989314407799,246.077427014612,23.0722994567796)) ;
#114753=CARTESIAN_POINT('Ctrl Pts',(59.5976708025309,246.078231023451,23.1032560403021)) ;
#114754=CARTESIAN_POINT('Ctrl Pts',(59.5964101642818,246.079766908328,23.1341689464842)) ;
#114755=CARTESIAN_POINT('Ctrl Pts',(59.5951495260327,246.082029153207,23.1650012267496)) ;
#114756=CARTESIAN_POINT('Ctrl Pts',(59.592353189247,246.087047245096,23.2333931223285)) ;
#114757=CARTESIAN_POINT('Ctrl Pts',(59.5895568524614,246.09566238462,23.3016559393828)) ;
#114758=CARTESIAN_POINT('Ctrl Pts',(59.5867605156757,246.107860974989,23.3693814266318)) ;
#114759=CARTESIAN_POINT('Ctrl Pts',(59.5839683593791,246.120041328615,23.4370056651086)) ;
#114760=CARTESIAN_POINT('Ctrl Pts',(59.5811762030826,246.135794414048,23.5040936888987)) ;
#114761=CARTESIAN_POINT('Ctrl Pts',(59.5783840467861,246.155054783387,23.5702413604452)) ;
#114762=CARTESIAN_POINT('Ctrl Pts',(59.5755951452465,246.174292701325,23.636311925064)) ;
#114763=CARTESIAN_POINT('Ctrl Pts',(59.572806243707,246.197029646677,23.7014438454389)) ;
#114764=CARTESIAN_POINT('Ctrl Pts',(59.5700173421674,246.223149295097,23.7652439775936)) ;
#114765=CARTESIAN_POINT('Ctrl Pts',(59.567230171318,246.249252734618,23.8290045177218)) ;
#114766=CARTESIAN_POINT('Ctrl Pts',(59.5644430004686,246.278734527295,23.8914344559251)) ;
#114767=CARTESIAN_POINT('Ctrl Pts',(59.5616558296193,246.311429268392,23.9521580793799)) ;
#114768=CARTESIAN_POINT('Ctrl Pts',(59.5588694369117,246.344114881543,24.0128647495911)) ;
#114769=CARTESIAN_POINT('Ctrl Pts',(59.556083044204,246.380011429681,24.0718656188513)) ;
#114770=CARTESIAN_POINT('Ctrl Pts',(59.5532966514964,246.418907154757,24.1288087805866)) ;
#114771=CARTESIAN_POINT('Ctrl Pts',(59.5505100855369,246.457805298284,24.1857554829242)) ;
#114772=CARTESIAN_POINT('Ctrl Pts',(59.5477235195775,246.499702710016,24.2406438198802)) ;
#114773=CARTESIAN_POINT('Ctrl Pts',(59.544936953618,246.544344850386,24.2931516348476)) ;
#114774=CARTESIAN_POINT('Ctrl Pts',(59.542147437078,246.589034260488,24.3457150481881)) ;
#114775=CARTESIAN_POINT('Ctrl Pts',(59.539357920538,246.636473880616,24.3958925345933)) ;
#114776=CARTESIAN_POINT('Ctrl Pts',(59.5365684039981,246.686370150645,24.4433965352695)) ;
#114777=CARTESIAN_POINT('Ctrl Pts',(59.5337772171642,246.736296297334,24.4909289801731)) ;
#114778=CARTESIAN_POINT('Ctrl Pts',(59.5309860303303,246.788681648685,24.5357844340528)) ;
#114779=CARTESIAN_POINT('Ctrl Pts',(59.5281948434965,246.843199315981,24.5777154540923)) ;
#114780=CARTESIAN_POINT('Ctrl Pts',(59.5253988913597,246.897810059526,24.6197180616052)) ;
#114781=CARTESIAN_POINT('Ctrl Pts',(59.5226029392228,246.954559980504,24.6587859926039)) ;
#114782=CARTESIAN_POINT('Ctrl Pts',(59.519806987086,247.01309372292,24.6947154541392)) ;
#114783=CARTESIAN_POINT('Ctrl Pts',(59.5185463514064,247.039485349293,24.7109152883797)) ;
#114784=CARTESIAN_POINT('Ctrl Pts',(59.5172857157268,247.066239289734,24.7264777260693)) ;
#114785=CARTESIAN_POINT('Ctrl Pts',(59.5160250800472,247.09332156075,24.741387251772)) ;
#114786=CARTESIAN_POINT('Ctrl Pts',(59.5132287433095,247.153395339883,24.774459498685)) ;
#114787=CARTESIAN_POINT('Ctrl Pts',(59.5104324065719,247.215321594776,24.8044456889594)) ;
#114788=CARTESIAN_POINT('Ctrl Pts',(59.5076360698342,247.278750643737,24.8311346906806)) ;
#114789=CARTESIAN_POINT('Ctrl Pts',(59.504843913586,247.342084867042,24.8577837926684)) ;
#114790=CARTESIAN_POINT('Ctrl Pts',(59.5020517573378,247.406916976534,24.8811453005803)) ;
#114791=CARTESIAN_POINT('Ctrl Pts',(59.4992596010895,247.472872476185,24.9010537958356)) ;
#114792=CARTESIAN_POINT('Ctrl Pts',(59.4964706995984,247.538751092915,24.9209390841816)) ;
#114793=CARTESIAN_POINT('Ctrl Pts',(59.4936817981073,247.605750031277,24.9373792129646)) ;
#114794=CARTESIAN_POINT('Ctrl Pts',(59.4908928966162,247.673476280123,24.9502574099)) ;
#114795=CARTESIAN_POINT('Ctrl Pts',(59.4881057258154,247.741160500536,24.9631276150973)) ;
#114796=CARTESIAN_POINT('Ctrl Pts',(59.4853185550146,247.809570654934,24.9724401819623)) ;
#114797=CARTESIAN_POINT('Ctrl Pts',(59.4825313842138,247.878301593193,24.9781289877404)) ;
#114798=CARTESIAN_POINT('Ctrl Pts',(59.4797449915547,247.947013342669,24.9838162052781)) ;
#114799=CARTESIAN_POINT('Ctrl Pts',(59.4769585988956,248.016045209274,24.9858816298161)) ;
#114800=CARTESIAN_POINT('Ctrl Pts',(59.4741722062365,248.084986735155,24.9843109767633)) ;
#114801=CARTESIAN_POINT('Ctrl Pts',(59.4713856403255,248.153932547673,24.9827402260506)) ;
#114802=CARTESIAN_POINT('Ctrl Pts',(59.4685990744145,248.22278751768,24.9775329626424)) ;
#114803=CARTESIAN_POINT('Ctrl Pts',(59.4658125085035,248.291142809627,24.968726985409)) ;
#114804=CARTESIAN_POINT('Ctrl Pts',(59.4630229920115,248.359570480204,24.9599116838855)) ;
#114805=CARTESIAN_POINT('Ctrl Pts',(59.4602334755195,248.42749692913,24.9474901268919)) ;
#114806=CARTESIAN_POINT('Ctrl Pts',(59.4574439590276,248.494521057544,24.9315516861224)) ;
#114807=CARTESIAN_POINT('Ctrl Pts',(59.4546527722415,248.561585318363,24.9156037018053)) ;
#114808=CARTESIAN_POINT('Ctrl Pts',(59.4518615854554,248.627745712456,24.8961347811673)) ;
#114809=CARTESIAN_POINT('Ctrl Pts',(59.4490703986694,248.692616606571,24.873284104553)) ;
#114810=CARTESIAN_POINT('Ctrl Pts',(59.4462744465796,248.757598252685,24.8503944157108)) ;
#114811=CARTESIAN_POINT('Ctrl Pts',(59.4434784944897,248.821285551641,24.8241116352291)) ;
#114812=CARTESIAN_POINT('Ctrl Pts',(59.4406825423999,248.883313948375,24.7946226027307)) ;
#114813=CARTESIAN_POINT('Ctrl Pts',(59.4394219062872,248.911281250542,24.7813266169258)) ;
#114814=CARTESIAN_POINT('Ctrl Pts',(59.4381612701744,248.938911662588,24.7673794386522)) ;
#114815=CARTESIAN_POINT('Ctrl Pts',(59.4369006340617,248.966173652772,24.7528011018477)) ;
#114816=CARTESIAN_POINT('Ctrl Pts',(59.4341042973507,249.026646062848,24.7204635081682)) ;
#114817=CARTESIAN_POINT('Ctrl Pts',(59.4313079606397,249.085540935002,24.6848906733029)) ;
#114818=CARTESIAN_POINT('Ctrl Pts',(59.4285116239287,249.142490654278,24.6462606792827)) ;
#114819=CARTESIAN_POINT('Ctrl Pts',(59.4257194677079,249.1993552344,24.6076884366455)) ;
#114820=CARTESIAN_POINT('Ctrl Pts',(59.4229273114872,249.25428003027,24.5660683793269)) ;
#114821=CARTESIAN_POINT('Ctrl Pts',(59.4201351552664,249.30692222625,24.5216243108424)) ;
#114822=CARTESIAN_POINT('Ctrl Pts',(59.4173462538038,249.359503058323,24.4772320498793)) ;
#114823=CARTESIAN_POINT('Ctrl Pts',(59.4145573523411,249.40980620179,24.4300226309428)) ;
#114824=CARTESIAN_POINT('Ctrl Pts',(59.4117684508785,249.457519532872,24.3802618965976)) ;
#114825=CARTESIAN_POINT('Ctrl Pts',(59.4089812801067,249.505203254795,24.3305320419557)) ;
#114826=CARTESIAN_POINT('Ctrl Pts',(59.406194109335,249.550300013629,24.2782543662633)) ;
#114827=CARTESIAN_POINT('Ctrl Pts',(59.4034069385633,249.59253353246,24.2237324974231)) ;
#114828=CARTESIAN_POINT('Ctrl Pts',(59.4006205459338,249.634755260235,24.169225850389)) ;
#114829=CARTESIAN_POINT('Ctrl Pts',(59.3978341533044,249.674115034592,24.1124766419563)) ;
#114830=CARTESIAN_POINT('Ctrl Pts',(59.3950477606749,249.710377145614,24.0538212060783)) ;
#114831=CARTESIAN_POINT('Ctrl Pts',(59.3922611947941,249.74664151133,23.9951621231416)) ;
#114832=CARTESIAN_POINT('Ctrl Pts',(59.3894746289132,249.779807575414,23.9345969962803)) ;
#114833=CARTESIAN_POINT('Ctrl Pts',(59.3866880630324,249.809684178051,23.8724891891972)) ;
#114834=CARTESIAN_POINT('Ctrl Pts',(59.3838985465712,249.839592415797,23.8103156187036)) ;
#114835=CARTESIAN_POINT('Ctrl Pts',(59.3811090301099,249.866204027935,23.7465965512774)) ;
#114836=CARTESIAN_POINT('Ctrl Pts',(59.3783195136487,249.889375309496,23.6817169758437)) ;
#114837=CARTESIAN_POINT('Ctrl Pts',(59.3755283268938,249.912560465449,23.6167985521189)) ;
#114838=CARTESIAN_POINT('Ctrl Pts',(59.3727371401388,249.93230105043,23.5507187077277)) ;
#114839=CARTESIAN_POINT('Ctrl Pts',(59.3699459533839,249.948503548174,23.4838766154075)) ;
#114840=CARTESIAN_POINT('Ctrl Pts',(59.3671500013255,249.964733707922,23.4169204057302)) ;
#114841=CARTESIAN_POINT('Ctrl Pts',(59.3643540492671,249.977413634704,23.3491998330237)) ;
#114842=CARTESIAN_POINT('Ctrl Pts',(59.3615580972086,249.986501258293,23.2811223767716)) ;
#114843=CARTESIAN_POINT('Ctrl Pts',(59.3602974608311,249.990598677934,23.2504276738417)) ;
#114844=CARTESIAN_POINT('Ctrl Pts',(59.3590368244536,249.993966516169,23.2196604587679)) ;
#114845=CARTESIAN_POINT('Ctrl Pts',(59.3577761880761,249.996604381633,23.1888580873807)) ;
#114846=CARTESIAN_POINT('Ctrl Pts',(59.3555100882696,250.001346166437,23.1334882368135)) ;
#114847=CARTESIAN_POINT('Ctrl Pts',(59.353243988463,250.003737676047,23.0779142731246)) ;
#114848=CARTESIAN_POINT('Ctrl Pts',(59.3509778886564,250.003764873166,23.0222802148703)) ;
#114849=CARTESIAN_POINT('',(58.8509778886861,250.003764876387,23.0222736029538)) ;
#114850=CARTESIAN_POINT('Ctrl Pts',(59.3509778886203,250.003764873166,23.0222802139838)) ;
#114851=CARTESIAN_POINT('Ctrl Pts',(59.3482144163914,250.003798039584,22.9544353756742)) ;
#114852=CARTESIAN_POINT('Ctrl Pts',(59.3454509441625,250.000310596167,22.8864497538944)) ;
#114853=CARTESIAN_POINT('Ctrl Pts',(59.3426874719336,249.993285064595,22.8187239509328)) ;
#114854=CARTESIAN_POINT('Ctrl Pts',(59.3399282395187,249.986270311835,22.751102055225)) ;
#114855=CARTESIAN_POINT('Ctrl Pts',(59.3371690071039,249.975728298068,22.6837396835978)) ;
#114856=CARTESIAN_POINT('Ctrl Pts',(59.334409774689,249.961693556368,22.6170370678999)) ;
#114857=CARTESIAN_POINT('Ctrl Pts',(59.3316528777829,249.947670694155,22.5503909115782)) ;
#114858=CARTESIAN_POINT('Ctrl Pts',(59.3288959808767,249.930161066131,22.4844038946956)) ;
#114859=CARTESIAN_POINT('Ctrl Pts',(59.3261390839706,249.909250777936,22.4194691868974)) ;
#114860=CARTESIAN_POINT('Ctrl Pts',(59.3233835269175,249.888350652149,22.354566037394)) ;
#114861=CARTESIAN_POINT('Ctrl Pts',(59.3206279698644,249.864053297393,22.2907146611191)) ;
#114862=CARTESIAN_POINT('Ctrl Pts',(59.3178724128113,249.836494990548,22.2282942038426)) ;
#114863=CARTESIAN_POINT('Ctrl Pts',(59.315117201858,249.808940145045,22.1658815866184)) ;
#114864=CARTESIAN_POINT('Ctrl Pts',(59.3123619909048,249.77812536494,22.1048999913118)) ;
#114865=CARTESIAN_POINT('Ctrl Pts',(59.3096067799515,249.744234736134,22.0457078407358)) ;
#114866=CARTESIAN_POINT('Ctrl Pts',(59.306849047208,249.710313087904,21.9864615127514)) ;
#114867=CARTESIAN_POINT('Ctrl Pts',(59.3040913144645,249.673310219145,21.9290083380907)) ;
#114868=CARTESIAN_POINT('Ctrl Pts',(59.301333581721,249.633455230042,21.8736803807023)) ;
#114869=CARTESIAN_POINT('Ctrl Pts',(59.2985745664988,249.593581706447,21.8183266931472)) ;
#114870=CARTESIAN_POINT('Ctrl Pts',(59.2958155512767,249.550853737858,21.7651005827768)) ;
#114871=CARTESIAN_POINT('Ctrl Pts',(59.2930565360545,249.5055408328,21.7143011012815)) ;
#114872=CARTESIAN_POINT('Ctrl Pts',(59.2902926206499,249.460147449205,21.6634113967496)) ;
#114873=CARTESIAN_POINT('Ctrl Pts',(59.2875287052452,249.412160316883,21.6149572842967)) ;
#114874=CARTESIAN_POINT('Ctrl Pts',(59.2847647898405,249.361885300937,21.5692004053125)) ;
#114875=CARTESIAN_POINT('Ctrl Pts',(59.2827271072572,249.324820300975,21.5354663788601)) ;
#114876=CARTESIAN_POINT('Ctrl Pts',(59.2806894246739,249.286512526135,21.5031975824389)) ;
#114877=CARTESIAN_POINT('Ctrl Pts',(59.2786517420906,249.24709473802,21.472483846834)) ;
#114878=CARTESIAN_POINT('Ctrl Pts',(59.2758554053502,249.193001225109,21.4303350116775)) ;
#114879=CARTESIAN_POINT('Ctrl Pts',(59.2730590686099,249.136590890501,21.390940763458)) ;
#114880=CARTESIAN_POINT('Ctrl Pts',(59.2702627318695,249.078175663034,21.3545648338026)) ;
#114881=CARTESIAN_POINT('Ctrl Pts',(59.2674705756192,249.019847765634,21.318243285728)) ;
#114882=CARTESIAN_POINT('Ctrl Pts',(59.264678419369,248.959521337593,21.2849313577405)) ;
#114883=CARTESIAN_POINT('Ctrl Pts',(59.2618862631187,248.897540033366,21.2548515632037)) ;
#114884=CARTESIAN_POINT('Ctrl Pts',(59.2590973616264,248.835630979446,21.224806832053)) ;
#114885=CARTESIAN_POINT('Ctrl Pts',(59.2563084601342,248.772071320159,21.1979869647537)) ;
#114886=CARTESIAN_POINT('Ctrl Pts',(59.2535195586419,248.707230678921,21.1745693649704)) ;
#114887=CARTESIAN_POINT('Ctrl Pts',(59.2507323878405,248.642430275427,21.1511662972978)) ;
#114888=CARTESIAN_POINT('Ctrl Pts',(59.2479452170391,248.576350927592,21.131161475055)) ;
#114889=CARTESIAN_POINT('Ctrl Pts',(59.2451580462377,248.509382248268,21.1146842066666)) ;
#114890=CARTESIAN_POINT('Ctrl Pts',(59.2423716535786,248.442432265739,21.09821153852)) ;
#114891=CARTESIAN_POINT('Ctrl Pts',(59.2395852609194,248.374593921047,21.08526458621)) ;
#114892=CARTESIAN_POINT('Ctrl Pts',(59.2367988682603,248.306270258855,21.0759223098388)) ;
#114893=CARTESIAN_POINT('Ctrl Pts',(59.2340123023499,248.237942348458,21.0665794525868)) ;
#114894=CARTESIAN_POINT('Ctrl Pts',(59.2312257364394,248.169129547296,21.0608417801966)) ;
#114895=CARTESIAN_POINT('Ctrl Pts',(59.2284391705289,248.100241527624,21.0587365672424)) ;
#114896=CARTESIAN_POINT('Ctrl Pts',(59.2256496540383,248.031280565261,21.0566291251648)) ;
#114897=CARTESIAN_POINT('Ctrl Pts',(59.2228601375477,247.962244716962,21.0581618333256)) ;
#114898=CARTESIAN_POINT('Ctrl Pts',(59.2200706210571,247.893544164318,21.0633098188821)) ;
#114899=CARTESIAN_POINT('Ctrl Pts',(59.2172794342729,247.82480247548,21.0684608869253)) ;
#114900=CARTESIAN_POINT('Ctrl Pts',(59.2144882474887,247.756396968761,21.0772314783121)) ;
#114901=CARTESIAN_POINT('Ctrl Pts',(59.2116970607045,247.688730424504,21.0895450935759)) ;
#114902=CARTESIAN_POINT('Ctrl Pts',(59.2089011086172,247.620948355341,21.1018797314773)) ;
#114903=CARTESIAN_POINT('Ctrl Pts',(59.20610515653,247.553908243824,21.1177693524051)) ;
#114904=CARTESIAN_POINT('Ctrl Pts',(59.2033092044427,247.487999587359,21.1370870658184)) ;
#114905=CARTESIAN_POINT('Ctrl Pts',(59.2020485683302,247.458282757501,21.1457970173414)) ;
#114906=CARTESIAN_POINT('Ctrl Pts',(59.2007879322176,247.428795693232,21.1552032118979)) ;
#114907=CARTESIAN_POINT('Ctrl Pts',(59.1995272961051,247.399572695686,21.1652908494305)) ;
#114908=CARTESIAN_POINT('Ctrl Pts',(59.196730959318,247.334750387128,21.1876671970903)) ;
#114909=CARTESIAN_POINT('Ctrl Pts',(59.1939346225309,247.270974611077,21.2134874063389)) ;
#114910=CARTESIAN_POINT('Ctrl Pts',(59.1911382857438,247.208636502649,21.2426337176701)) ;
#114911=CARTESIAN_POINT('Ctrl Pts',(59.1883461294462,247.146391588935,21.2717364556203)) ;
#114912=CARTESIAN_POINT('Ctrl Pts',(59.1855539731486,247.085580518145,21.3041552202885)) ;
#114913=CARTESIAN_POINT('Ctrl Pts',(59.182761816851,247.026577161891,21.3397231865845)) ;
#114914=CARTESIAN_POINT('Ctrl Pts',(59.1799729153109,246.967642584598,21.375249692056)) ;
#114915=CARTESIAN_POINT('Ctrl Pts',(59.1771840137707,246.910511955099,21.4139178560389)) ;
#114916=CARTESIAN_POINT('Ctrl Pts',(59.1743951122305,246.855535481128,21.4555144929768)) ;
#114917=CARTESIAN_POINT('Ctrl Pts',(59.1716079413808,246.800593123551,21.49708531656)) ;
#114918=CARTESIAN_POINT('Ctrl Pts',(59.1688207705312,246.747802660129,21.5415807124295)) ;
#114919=CARTESIAN_POINT('Ctrl Pts',(59.1660335996815,246.697484872359,21.5887445203145)) ;
#114920=CARTESIAN_POINT('Ctrl Pts',(59.1632472069738,246.647181132664,21.6358951606747)) ;
#114921=CARTESIAN_POINT('Ctrl Pts',(59.1604608142662,246.599349056025,21.6857123985113)) ;
#114922=CARTESIAN_POINT('Ctrl Pts',(59.1576744215586,246.554274534302,21.7379013685107)) ;
#114923=CARTESIAN_POINT('Ctrl Pts',(59.1548878555993,246.509197209947,21.7900935835016)) ;
#114924=CARTESIAN_POINT('Ctrl Pts',(59.1521012896402,246.466878099785,21.8446574502955)) ;
#114925=CARTESIAN_POINT('Ctrl Pts',(59.1493147236809,246.42756337608,21.9012643741764)) ;
#114926=CARTESIAN_POINT('Ctrl Pts',(59.1465252071417,246.388207023631,21.9579312367999)) ;
#114927=CARTESIAN_POINT('Ctrl Pts',(59.1437356906024,246.351861686745,22.0166450698203)) ;
#114928=CARTESIAN_POINT('Ctrl Pts',(59.1409461740632,246.318730095887,22.0770484267869)) ;
#114929=CARTESIAN_POINT('Ctrl Pts',(59.1381549872303,246.28557866665,22.1374879517928)) ;
#114930=CARTESIAN_POINT('Ctrl Pts',(59.1353638003974,246.255645026362,22.1996185719482)) ;
#114931=CARTESIAN_POINT('Ctrl Pts',(59.1325726135645,246.229084588378,22.2630609050312)) ;
#114932=CARTESIAN_POINT('Ctrl Pts',(59.129776661429,246.202478804622,22.3266115511476)) ;
#114933=CARTESIAN_POINT('Ctrl Pts',(59.1269807092936,246.179257882127,22.3914779178238)) ;
#114934=CARTESIAN_POINT('Ctrl Pts',(59.1241847571581,246.15952774699,22.4572642916397)) ;
#114935=CARTESIAN_POINT('Ctrl Pts',(59.1229241214786,246.150631846378,22.4869259761183)) ;
#114936=CARTESIAN_POINT('Ctrl Pts',(59.121663485799,246.142444904077,22.5167745401311)) ;
#114937=CARTESIAN_POINT('Ctrl Pts',(59.1204028501195,246.134973208986,22.5467731590085)) ;
#114938=CARTESIAN_POINT('Ctrl Pts',(59.1176065136226,246.118399527931,22.6133159629168)) ;
#114939=CARTESIAN_POINT('Ctrl Pts',(59.1148101771257,246.105283563965,22.6808585669027)) ;
#114940=CARTESIAN_POINT('Ctrl Pts',(59.1120138406289,246.095739791186,22.7490088617933)) ;
#114941=CARTESIAN_POINT('Ctrl Pts',(59.1092216846219,246.086210286234,22.8170572728011)) ;
#114942=CARTESIAN_POINT('Ctrl Pts',(59.1064295286149,246.080242440688,22.8857110893508)) ;
#114943=CARTESIAN_POINT('Ctrl Pts',(59.1036373726079,246.077900182911,22.9545659308058)) ;
#114944=CARTESIAN_POINT('Ctrl Pts',(59.1008484713576,246.075560655454,23.0233405096432)) ;
#114945=CARTESIAN_POINT('Ctrl Pts',(59.0980595701072,246.076838338569,23.0923151597208)) ;
#114946=CARTESIAN_POINT('Ctrl Pts',(59.0952706688569,246.081745394066,23.1610800694073)) ;
#114947=CARTESIAN_POINT('Ctrl Pts',(59.0924834982963,246.086649404423,23.229802306113)) ;
#114948=CARTESIAN_POINT('Ctrl Pts',(59.0896963277358,246.095178284277,23.2983145721291)) ;
#114949=CARTESIAN_POINT('Ctrl Pts',(59.0869091571752,246.107292126462,23.3662083014096)) ;
#114950=CARTESIAN_POINT('Ctrl Pts',(59.0841227647556,246.119402586622,23.4340830756645)) ;
#114951=CARTESIAN_POINT('Ctrl Pts',(59.081336372336,246.135095935891,23.5013391730481)) ;
#114952=CARTESIAN_POINT('Ctrl Pts',(59.0785499799164,246.15428079973,23.5675761808417)) ;
#114953=CARTESIAN_POINT('Ctrl Pts',(59.0757634142437,246.17346685645,23.6338173071393)) ;
#114954=CARTESIAN_POINT('Ctrl Pts',(59.0729768485709,246.196144719733,23.6990387473166)) ;
#114955=CARTESIAN_POINT('Ctrl Pts',(59.0701902828982,246.222173086422,23.7628550034729)) ;
#114956=CARTESIAN_POINT('Ctrl Pts',(59.0674007666411,246.24822901352,23.8267388321427)) ;
#114957=CARTESIAN_POINT('Ctrl Pts',(59.064611250384,246.2776423383,23.8892140521497)) ;
#114958=CARTESIAN_POINT('Ctrl Pts',(59.0618217341269,246.310223889416,23.9499158597772)) ;
#114959=CARTESIAN_POINT('Ctrl Pts',(59.0590305475741,246.342824949586,24.0106540141971)) ;
#114960=CARTESIAN_POINT('Ctrl Pts',(59.0562393610214,246.378597757097,24.0696162231625)) ;
#114961=CARTESIAN_POINT('Ctrl Pts',(59.0534481744686,246.417308958266,24.1264653959102)) ;
#114962=CARTESIAN_POINT('Ctrl Pts',(59.0506522226072,246.456086249901,24.1834116255363)) ;
#114963=CARTESIAN_POINT('Ctrl Pts',(59.0478562707458,246.497811650241,24.2382372287799)) ;
#114964=CARTESIAN_POINT('Ctrl Pts',(59.0450603188843,246.54221113912,24.2906377022076)) ;
#114965=CARTESIAN_POINT('Ctrl Pts',(59.0437996806343,246.562229972326,24.3142640178237)) ;
#114966=CARTESIAN_POINT('Ctrl Pts',(59.0425390423842,246.582791925877,24.3373978189575)) ;
#114967=CARTESIAN_POINT('Ctrl Pts',(59.0412784041341,246.603869554451,24.3600137604256)) ;
#114968=CARTESIAN_POINT('Ctrl Pts',(59.0384820671789,246.650623769395,24.4101802478371)) ;
#114969=CARTESIAN_POINT('Ctrl Pts',(59.0356857302238,246.700100944889,24.4579928233431)) ;
#114970=CARTESIAN_POINT('Ctrl Pts',(59.0328893932686,246.752034741746,24.5031417815244)) ;
#114971=CARTESIAN_POINT('Ctrl Pts',(59.0300972368053,246.80389089817,24.548223242529)) ;
#114972=CARTESIAN_POINT('Ctrl Pts',(59.0273050803419,246.858196019243,24.5906486701497)) ;
#114973=CARTESIAN_POINT('Ctrl Pts',(59.0245129238785,246.914645925946,24.630144046603)) ;
#114974=CARTESIAN_POINT('Ctrl Pts',(59.0217240221768,246.971030030109,24.6695933840767)) ;
#114975=CARTESIAN_POINT('Ctrl Pts',(59.018935120475,247.029553554085,24.7061191738536)) ;
#114976=CARTESIAN_POINT('Ctrl Pts',(59.0161462187732,247.089879548498,24.739487837926)) ;
#114977=CARTESIAN_POINT('Ctrl Pts',(59.0133590477647,247.150168106745,24.7728357945925)) ;
#114978=CARTESIAN_POINT('Ctrl Pts',(59.0105718767561,247.212256487896,24.8030302751658)) ;
#114979=CARTESIAN_POINT('Ctrl Pts',(59.0077847057475,247.275780404892,24.8298820342521)) ;
#114980=CARTESIAN_POINT('Ctrl Pts',(59.0049983128838,247.339286586767,24.8567262966472)) ;
#114981=CARTESIAN_POINT('Ctrl Pts',(59.0022119200202,247.404227056915,24.8802294993308)) ;
#114982=CARTESIAN_POINT('Ctrl Pts',(58.9994255271565,247.470216309838,24.9002499904485)) ;
#114983=CARTESIAN_POINT('Ctrl Pts',(58.9966389610445,247.536209665749,24.9202717263723)) ;
#114984=CARTESIAN_POINT('Ctrl Pts',(58.9938523949324,247.603251463472,24.936810180781)) ;
#114985=CARTESIAN_POINT('Ctrl Pts',(58.9910658288203,247.670941486527,24.949773690877)) ;
#114986=CARTESIAN_POINT('Ctrl Pts',(58.9882763121339,247.738703183619,24.9627509274732)) ;
#114987=CARTESIAN_POINT('Ctrl Pts',(58.9854867954475,247.80711399284,24.972145573031)) ;
#114988=CARTESIAN_POINT('Ctrl Pts',(58.982697278761,247.875764955148,24.9779173766203)) ;
#114989=CARTESIAN_POINT('Ctrl Pts',(58.979906091784,247.94445702388,24.9836926362167)) ;
#114990=CARTESIAN_POINT('Ctrl Pts',(58.977114904807,248.013389041257,24.9858407211746)) ;
#114991=CARTESIAN_POINT('Ctrl Pts',(58.97432371783,248.082151199172,24.9843735281036)) ;
#114992=CARTESIAN_POINT('Ctrl Pts',(58.9715277655566,248.151030752329,24.9829038301449)) ;
#114993=CARTESIAN_POINT('Ctrl Pts',(58.9687318132831,248.219739378087,24.9778065719954)) ;
#114994=CARTESIAN_POINT('Ctrl Pts',(58.9659358610097,248.287872422303,24.9691455071197)) ;
#114995=CARTESIAN_POINT('Ctrl Pts',(58.9646752267226,248.318592135381,24.9652404206671)) ;
#114996=CARTESIAN_POINT('Ctrl Pts',(58.9634145924355,248.349194980317,24.9606115349833)) ;
#114997=CARTESIAN_POINT('Ctrl Pts',(58.9621539581485,248.379644748521,24.9552680443661)) ;
#114998=CARTESIAN_POINT('Ctrl Pts',(58.9593576209136,248.447188382306,24.9434151208572)) ;
#114999=CARTESIAN_POINT('Ctrl Pts',(58.9565612836786,248.514242781497,24.9279962372586)) ;
#115000=CARTESIAN_POINT('Ctrl Pts',(58.9537649464437,248.580403117524,24.9090658720766)) ;
#115001=CARTESIAN_POINT('Ctrl Pts',(58.950972789694,248.646464544771,24.8901638075269)) ;
#115002=CARTESIAN_POINT('Ctrl Pts',(58.9481806329443,248.711634093535,24.8677608145103)) ;
#115003=CARTESIAN_POINT('Ctrl Pts',(58.9453884761946,248.77551622923,24.8419625485013)) ;
#115004=CARTESIAN_POINT('Ctrl Pts',(58.9425995741983,248.839323898978,24.8161943549422)) ;
#115005=CARTESIAN_POINT('Ctrl Pts',(58.939810672202,248.901846683219,24.7870389319116)) ;
#115006=CARTESIAN_POINT('Ctrl Pts',(58.9370217702057,248.962705088742,24.7546514520135)) ;
#115007=CARTESIAN_POINT('Ctrl Pts',(58.9342345988977,249.023525727814,24.7222840705744)) ;
#115008=CARTESIAN_POINT('Ctrl Pts',(58.9314474275897,249.082683604803,24.6866888412435)) ;
#115009=CARTESIAN_POINT('Ctrl Pts',(58.9286602562817,249.139821492819,24.6480680210235)) ;
#115010=CARTESIAN_POINT('Ctrl Pts',(58.9258738631143,249.196943428708,24.6094579832144)) ;
#115011=CARTESIAN_POINT('Ctrl Pts',(58.9230874699468,249.252046088789,24.5678243062547)) ;
#115012=CARTESIAN_POINT('Ctrl Pts',(58.9203010767794,249.304800581892,24.5234129787613)) ;
#115013=CARTESIAN_POINT('Ctrl Pts',(58.9175145103596,249.357558355164,24.4789988898608)) ;
#115014=CARTESIAN_POINT('Ctrl Pts',(58.9147279439398,249.407967297763,24.4318071256052)) ;
#115015=CARTESIAN_POINT('Ctrl Pts',(58.91194137752,249.455732409706,24.3821232562536)) ;
#115016=CARTESIAN_POINT('Ctrl Pts',(58.9091518605222,249.503548098117,24.3323867787421)) ;
#115017=CARTESIAN_POINT('Ctrl Pts',(58.9063623435245,249.54871402837,24.2801532845457)) ;
#115018=CARTESIAN_POINT('Ctrl Pts',(58.9035728265267,249.590973537813,24.2257436973031)) ;
#115019=CARTESIAN_POINT('Ctrl Pts',(58.9007816392358,249.633258351196,24.171301530958)) ;
#115020=CARTESIAN_POINT('Ctrl Pts',(58.8979904519449,249.672632999894,24.1146810812941)) ;
#115021=CARTESIAN_POINT('Ctrl Pts',(58.895199264654,249.708884077981,24.05623240857)) ;
#115022=CARTESIAN_POINT('Ctrl Pts',(58.8924033120661,249.745197046273,23.9976839484601)) ;
#115023=CARTESIAN_POINT('Ctrl Pts',(58.8896073594782,249.778375564698,23.9373014658192)) ;
#115024=CARTESIAN_POINT('Ctrl Pts',(58.8868114068903,249.808252512498,23.8754589662552)) ;
#115025=CARTESIAN_POINT('Ctrl Pts',(58.8855507753145,249.821723350289,23.8475755865395)) ;
#115026=CARTESIAN_POINT('Ctrl Pts',(58.8842901437388,249.834523668133,23.8193956569121)) ;
#115027=CARTESIAN_POINT('Ctrl Pts',(58.883029512163,249.846641437717,23.7909545454152)) ;
#115028=CARTESIAN_POINT('Ctrl Pts',(58.8799366091877,249.876371841364,23.7211755552172)) ;
#115029=CARTESIAN_POINT('Ctrl Pts',(58.8768437062124,249.902089895002,23.6495903556867)) ;
#115030=CARTESIAN_POINT('Ctrl Pts',(58.8737508032372,249.923596879455,23.5766523954176)) ;
#115031=CARTESIAN_POINT('Ctrl Pts',(58.8706676326043,249.945036188545,23.5039439467784)) ;
#115032=CARTESIAN_POINT('Ctrl Pts',(58.8675844619714,249.962290726759,23.4298915073856)) ;
#115033=CARTESIAN_POINT('Ctrl Pts',(58.8645012913385,249.975210146838,23.3549667819474)) ;
#115034=CARTESIAN_POINT('Ctrl Pts',(58.8614340620078,249.988062768026,23.2804294491742)) ;
#115035=CARTESIAN_POINT('Ctrl Pts',(58.8583668326771,249.996624855943,23.2050291159775)) ;
#115036=CARTESIAN_POINT('Ctrl Pts',(58.8552996033464,250.000796615895,23.1292483552738)) ;
#115037=CARTESIAN_POINT('Ctrl Pts',(58.8538590317929,250.002755947287,23.0936567524309)) ;
#115038=CARTESIAN_POINT('Ctrl Pts',(58.8524184602395,250.003747540578,23.0579814668026)) ;
#115039=CARTESIAN_POINT('Ctrl Pts',(58.8509778886861,250.003764876387,23.0222736029538)) ;
#115040=CARTESIAN_POINT('',(58.3509778886279,250.003764344364,23.019588882796)) ;
#115041=CARTESIAN_POINT('Ctrl Pts',(58.8509778886564,250.003764876387,23.0222736022181)) ;
#115042=CARTESIAN_POINT('Ctrl Pts',(58.8481505255564,250.003798900791,22.9521909351076)) ;
#115043=CARTESIAN_POINT('Ctrl Pts',(58.8453231624564,250.000076419562,22.8821143861072)) ;
#115044=CARTESIAN_POINT('Ctrl Pts',(58.8424957993564,249.992625746799,22.812465884105)) ;
#115045=CARTESIAN_POINT('Ctrl Pts',(58.8396672877594,249.985172047514,22.7427890903375)) ;
#115046=CARTESIAN_POINT('Ctrl Pts',(58.8368387761624,249.973987198681,22.6735411566306)) ;
#115047=CARTESIAN_POINT('Ctrl Pts',(58.8340102645655,249.9591511568,22.6051369934624)) ;
#115048=CARTESIAN_POINT('Ctrl Pts',(58.8311775185464,249.944292904629,22.5366304258706)) ;
#115049=CARTESIAN_POINT('Ctrl Pts',(58.8283447725273,249.925772649025,22.4689706108314)) ;
#115050=CARTESIAN_POINT('Ctrl Pts',(58.8255120265083,249.903720959079,22.4025598565522)) ;
#115051=CARTESIAN_POINT('Ctrl Pts',(58.8226769540086,249.881651158498,22.3360945603783)) ;
#115052=CARTESIAN_POINT('Ctrl Pts',(58.8198418815089,249.856044320734,22.2708808052718)) ;
#115053=CARTESIAN_POINT('Ctrl Pts',(58.8170068090091,249.827079144851,22.2073007817881)) ;
#115054=CARTESIAN_POINT('Ctrl Pts',(58.8141660072348,249.798055434505,22.1435922722015)) ;
#115055=CARTESIAN_POINT('Ctrl Pts',(58.8113252054604,249.765660051054,22.081524504325)) ;
#115056=CARTESIAN_POINT('Ctrl Pts',(58.8084844036861,249.730117371809,22.021454564679)) ;
#115057=CARTESIAN_POINT('Ctrl Pts',(58.8069579578499,249.711019251261,21.989177230132)) ;
#115058=CARTESIAN_POINT('Ctrl Pts',(58.8054315120137,249.69101317592,21.9574762078088)) ;
#115059=CARTESIAN_POINT('Ctrl Pts',(58.8039050661775,249.670138832976,21.9264030453423)) ;
#115060=CARTESIAN_POINT('Ctrl Pts',(58.801108726491,249.63189852846,21.8694792323062)) ;
#115061=CARTESIAN_POINT('Ctrl Pts',(58.7983123868046,249.590597531178,21.8144495208064)) ;
#115062=CARTESIAN_POINT('Ctrl Pts',(58.7955160471181,249.546449899716,21.7616618094488)) ;
#115063=CARTESIAN_POINT('Ctrl Pts',(58.7927238879383,249.502368268629,21.7089530153205)) ;
#115064=CARTESIAN_POINT('Ctrl Pts',(58.7899317287585,249.455448762239,21.6584799424396)) ;
#115065=CARTESIAN_POINT('Ctrl Pts',(58.7871395695787,249.405948442476,21.6105612289866)) ;
#115066=CARTESIAN_POINT('Ctrl Pts',(58.7843506651955,249.356505824819,21.5626983739753)) ;
#115067=CARTESIAN_POINT('Ctrl Pts',(58.7815617608122,249.30448871986,21.51738430438)) ;
#115068=CARTESIAN_POINT('Ctrl Pts',(58.7787728564289,249.25019293795,21.4749029045106)) ;
#115069=CARTESIAN_POINT('Ctrl Pts',(58.7759856827621,249.195930850491,21.4324478674157)) ;
#115070=CARTESIAN_POINT('Ctrl Pts',(58.7731985090952,249.139393277057,21.3928223145572)) ;
#115071=CARTESIAN_POINT('Ctrl Pts',(58.7704113354284,249.080910027098,21.3562706740573)) ;
#115072=CARTESIAN_POINT('Ctrl Pts',(58.7676249399336,249.02244310552,21.3197292386862)) ;
#115073=CARTESIAN_POINT('Ctrl Pts',(58.7648385444389,248.962032001927,21.2862602718357)) ;
#115074=CARTESIAN_POINT('Ctrl Pts',(58.7620521489441,248.900034997751,21.2560645586065)) ;
#115075=CARTESIAN_POINT('Ctrl Pts',(58.7592655802319,248.838034139506,21.2258669682488)) ;
#115076=CARTESIAN_POINT('Ctrl Pts',(58.7564790115198,248.774447627337,21.1989432481034)) ;
#115077=CARTESIAN_POINT('Ctrl Pts',(58.7536924428076,248.709656167469,21.17544714661)) ;
#115078=CARTESIAN_POINT('Ctrl Pts',(58.7509029235853,248.644796104282,21.1519261666751)) ;
#115079=CARTESIAN_POINT('Ctrl Pts',(58.748113404363,248.57872900956,21.1318402157891)) ;
#115080=CARTESIAN_POINT('Ctrl Pts',(58.7453238851406,248.51185234569,21.1152936577427)) ;
#115081=CARTESIAN_POINT('Ctrl Pts',(58.7425326956608,248.444935638628,21.0987371922495)) ;
#115082=CARTESIAN_POINT('Ctrl Pts',(58.7397415061809,248.37720887972,21.0857244300631)) ;
#115083=CARTESIAN_POINT('Ctrl Pts',(58.736950316701,248.30907860944,21.076308376674)) ;
#115084=CARTESIAN_POINT('Ctrl Pts',(58.7341543620011,248.240832024689,21.0668762478566)) ;
#115085=CARTESIAN_POINT('Ctrl Pts',(58.7313584073012,248.17218104245,21.0610531242674)) ;
#115086=CARTESIAN_POINT('Ctrl Pts',(58.7285624526013,248.103535307741,21.0588399916076)) ;
#115087=CARTESIAN_POINT('Ctrl Pts',(58.7273018417982,248.072585037063,21.0578421575083)) ;
#115088=CARTESIAN_POINT('Ctrl Pts',(58.726041230995,248.041635801624,21.0575774690523)) ;
#115089=CARTESIAN_POINT('Ctrl Pts',(58.7247806201919,248.010724805815,21.0580425688778)) ;
#115090=CARTESIAN_POINT('Ctrl Pts',(58.7219842798933,247.942156725141,21.0590742730181)) ;
#115091=CARTESIAN_POINT('Ctrl Pts',(58.7191879395947,247.873508291733,21.0637044531742)) ;
#115092=CARTESIAN_POINT('Ctrl Pts',(58.7163915992962,247.805187857571,21.0719432798719)) ;
#115093=CARTESIAN_POINT('Ctrl Pts',(58.7135994394385,247.736969560314,21.0801697897824)) ;
#115094=CARTESIAN_POINT('Ctrl Pts',(58.7108072795809,247.669078772524,21.0919941805918)) ;
#115095=CARTESIAN_POINT('Ctrl Pts',(58.7080151197233,247.601922755114,21.1073746202295)) ;
#115096=CARTESIAN_POINT('Ctrl Pts',(58.7052262145697,247.534845018667,21.1227371315315)) ;
#115097=CARTESIAN_POINT('Ctrl Pts',(58.7024373094162,247.468500827733,21.1416473499285)) ;
#115098=CARTESIAN_POINT('Ctrl Pts',(58.6996484042626,247.403289427283,21.1640120136241)) ;
#115099=CARTESIAN_POINT('Ctrl Pts',(58.6968612297687,247.338118493875,21.1863627988909)) ;
#115100=CARTESIAN_POINT('Ctrl Pts',(58.6940740552748,247.274079419687,21.2121636179814)) ;
#115101=CARTESIAN_POINT('Ctrl Pts',(58.691286880781,247.211556902627,21.2412711979733)) ;
#115102=CARTESIAN_POINT('Ctrl Pts',(58.6885004844042,247.149051840463,21.2703706517766)) ;
#115103=CARTESIAN_POINT('Ctrl Pts',(58.6857140880274,247.088062939629,21.3027748266298)) ;
#115104=CARTESIAN_POINT('Ctrl Pts',(58.6829276916506,247.028953828074,21.3382927901524)) ;
#115105=CARTESIAN_POINT('Ctrl Pts',(58.6801411220031,246.969841040849,21.3738129623415)) ;
#115106=CARTESIAN_POINT('Ctrl Pts',(58.6773545523557,246.912608694361,21.4124470526189)) ;
#115107=CARTESIAN_POINT('Ctrl Pts',(58.6745679827083,246.857593205218,21.4539596891866)) ;
#115108=CARTESIAN_POINT('Ctrl Pts',(58.6717784624778,246.802519462457,21.4955162817626)) ;
#115109=CARTESIAN_POINT('Ctrl Pts',(58.6689889422474,246.749667654034,21.5399572071158)) ;
#115110=CARTESIAN_POINT('Ctrl Pts',(58.666199422017,246.699341926844,21.5870061266556)) ;
#115111=CARTESIAN_POINT('Ctrl Pts',(58.663408231486,246.648986065767,21.6340832180065)) ;
#115112=CARTESIAN_POINT('Ctrl Pts',(58.660617040955,246.601159636707,21.6837710578745)) ;
#115113=CARTESIAN_POINT('Ctrl Pts',(58.6578258504241,246.556128676984,21.7357577022364)) ;
#115114=CARTESIAN_POINT('Ctrl Pts',(58.6550298946189,246.511020837926,21.7878331010608)) ;
#115115=CARTESIAN_POINT('Ctrl Pts',(58.6522339388137,246.46871829441,21.842214749955)) ;
#115116=CARTESIAN_POINT('Ctrl Pts',(58.6494379830085,246.429445163528,21.898559747003)) ;
#115117=CARTESIAN_POINT('Ctrl Pts',(58.6481773800745,246.411738222693,21.9239638211535)) ;
#115118=CARTESIAN_POINT('Ctrl Pts',(58.6469167771404,246.394646494269,21.9497666479011)) ;
#115119=CARTESIAN_POINT('Ctrl Pts',(58.6456561742064,246.378187442659,21.9759352063564)) ;
#115120=CARTESIAN_POINT('Ctrl Pts',(58.6428598595974,246.341677384473,22.0339832406195)) ;
#115121=CARTESIAN_POINT('Ctrl Pts',(58.6400635449883,246.308140358677,22.0940600892534)) ;
#115122=CARTESIAN_POINT('Ctrl Pts',(58.6372672303792,246.27780747817,22.1558289491428)) ;
#115123=CARTESIAN_POINT('Ctrl Pts',(58.6344750962971,246.247519945717,22.2175054637788)) ;
#115124=CARTESIAN_POINT('Ctrl Pts',(58.6316829622149,246.220427265785,22.2808685320038)) ;
#115125=CARTESIAN_POINT('Ctrl Pts',(58.6288908281328,246.196716358875,22.345553919129)) ;
#115126=CARTESIAN_POINT('Ctrl Pts',(58.6261019487543,246.17303309103,22.4101639045139)) ;
#115127=CARTESIAN_POINT('Ctrl Pts',(58.6233130693759,246.152723935081,22.4760926887444)) ;
#115128=CARTESIAN_POINT('Ctrl Pts',(58.6205241899974,246.135928324648,22.5429547235698)) ;
#115129=CARTESIAN_POINT('Ctrl Pts',(58.6177370412627,246.119143136759,22.6097752670487)) ;
#115130=CARTESIAN_POINT('Ctrl Pts',(58.6149498925279,246.105867288354,22.6775274372463)) ;
#115131=CARTESIAN_POINT('Ctrl Pts',(58.6121627437932,246.096190355381,22.7458106212959)) ;
#115132=CARTESIAN_POINT('Ctrl Pts',(58.6093763731201,246.086516123825,22.8140747433828)) ;
#115133=CARTESIAN_POINT('Ctrl Pts',(58.606590002447,246.080438881949,22.8828690992664)) ;
#115134=CARTESIAN_POINT('Ctrl Pts',(58.6038036317739,246.077996764028,22.9517847621219)) ;
#115135=CARTESIAN_POINT('Ctrl Pts',(58.6010170877351,246.075554494161,23.0207047128525)) ;
#115136=CARTESIAN_POINT('Ctrl Pts',(58.5982305436963,246.076747812098,23.0897454949275)) ;
#115137=CARTESIAN_POINT('Ctrl Pts',(58.5954439996576,246.081562762467,23.1584967717109)) ;
#115138=CARTESIAN_POINT('Ctrl Pts',(58.5926545047176,246.086382811783,23.2273208548889)) ;
#115139=CARTESIAN_POINT('Ctrl Pts',(58.5898650097776,246.094832112971,23.2958543303937)) ;
#115140=CARTESIAN_POINT('Ctrl Pts',(58.5870755148377,246.106844775149,23.3636915855581)) ;
#115141=CARTESIAN_POINT('Ctrl Pts',(58.5842843494512,246.118864630927,23.4315694640283)) ;
#115142=CARTESIAN_POINT('Ctrl Pts',(58.5814931840647,246.134451983669,23.4987498142027)) ;
#115143=CARTESIAN_POINT('Ctrl Pts',(58.5787020186782,246.15349031868,23.5648395660296)) ;
#115144=CARTESIAN_POINT('Ctrl Pts',(58.5759060875323,246.172561160589,23.6310421624277)) ;
#115145=CARTESIAN_POINT('Ctrl Pts',(58.5731101563863,246.195094584209,23.6961499805135)) ;
#115146=CARTESIAN_POINT('Ctrl Pts',(58.5703142252404,246.220925270349,23.7597882209357)) ;
#115147=CARTESIAN_POINT('Ctrl Pts',(58.5690533929005,246.232573684687,23.7884860490959)) ;
#115148=CARTESIAN_POINT('Ctrl Pts',(58.5677925605607,246.244891992381,23.8168853416463)) ;
#115149=CARTESIAN_POINT('Ctrl Pts',(58.5665317282209,246.257862018413,23.8449534396603)) ;
#115150=CARTESIAN_POINT('Ctrl Pts',(58.5637353561837,246.286627951021,23.907205050714)) ;
#115151=CARTESIAN_POINT('Ctrl Pts',(58.5609389841465,246.318715472937,23.9680699191845)) ;
#115152=CARTESIAN_POINT('Ctrl Pts',(58.5581426121093,246.353968178566,24.0271706885432)) ;
#115153=CARTESIAN_POINT('Ctrl Pts',(58.5553504207015,246.389168180729,24.0861831011273)) ;
#115154=CARTESIAN_POINT('Ctrl Pts',(58.5525582292937,246.427523725309,24.1434362309142)) ;
#115155=CARTESIAN_POINT('Ctrl Pts',(58.5497660378859,246.468831320435,24.1985748198616)) ;
#115156=CARTESIAN_POINT('Ctrl Pts',(58.5469771016104,246.510090759233,24.2536491283305)) ;
#115157=CARTESIAN_POINT('Ctrl Pts',(58.5441881653349,246.554295120499,24.3066134009809)) ;
#115158=CARTESIAN_POINT('Ctrl Pts',(58.5413992290594,246.601197159575,24.3571405748899)) ;
#115159=CARTESIAN_POINT('Ctrl Pts',(58.5386120237277,246.64807008906,24.4076363892807)) ;
#115160=CARTESIAN_POINT('Ctrl Pts',(58.5358248183959,246.697637041688,24.4556977466538)) ;
#115161=CARTESIAN_POINT('Ctrl Pts',(58.5330376130642,246.749610966573,24.5010311726646)) ;
#115162=CARTESIAN_POINT('Ctrl Pts',(58.5302511861787,246.80157037552,24.5463519373794)) ;
#115163=CARTESIAN_POINT('Ctrl Pts',(58.5274647592931,246.855935052385,24.5889459608517)) ;
#115164=CARTESIAN_POINT('Ctrl Pts',(58.5246783324075,246.912382936087,24.6285583647508)) ;
#115165=CARTESIAN_POINT('Ctrl Pts',(58.5218917326256,246.96883432235,24.6681732265785)) ;
#115166=CARTESIAN_POINT('Ctrl Pts',(58.5191051328438,247.027368768849,24.7048058217007)) ;
#115167=CARTESIAN_POINT('Ctrl Pts',(58.5163185330619,247.087634639173,24.7382441742145)) ;
#115168=CARTESIAN_POINT('Ctrl Pts',(58.5135289834622,247.14796430529,24.7717179236481)) ;
#115169=CARTESIAN_POINT('Ctrl Pts',(58.5107394338625,247.210028622949,24.8019904439401)) ;
#115170=CARTESIAN_POINT('Ctrl Pts',(58.5079498842627,247.273451606802,24.8288958757875)) ;
#115171=CARTESIAN_POINT('Ctrl Pts',(58.505158664758,247.336912557487,24.8558174140043)) ;
#115172=CARTESIAN_POINT('Ctrl Pts',(58.5023674452532,247.401733331759,24.8793676845295)) ;
#115173=CARTESIAN_POINT('Ctrl Pts',(58.4995762257484,247.467520864779,24.8994301066198)) ;
#115174=CARTESIAN_POINT('Ctrl Pts',(58.4967802418732,247.533420691432,24.9195267735309)) ;
#115175=CARTESIAN_POINT('Ctrl Pts',(58.4939842579979,247.600290094166,24.9361235920358)) ;
#115176=CARTESIAN_POINT('Ctrl Pts',(58.4911882741226,247.667724722639,24.9491548570577)) ;
#115177=CARTESIAN_POINT('Ctrl Pts',(58.4899279434935,247.698121867801,24.9550288903769)) ;
#115178=CARTESIAN_POINT('Ctrl Pts',(58.4886676128644,247.728633780147,24.960179144585)) ;
#115179=CARTESIAN_POINT('Ctrl Pts',(58.4874072822353,247.759223217459,24.9646030573924)) ;
#115180=CARTESIAN_POINT('Ctrl Pts',(58.4846109259678,247.827093475288,24.9744186058051)) ;
#115181=CARTESIAN_POINT('Ctrl Pts',(58.4818145697003,247.895611647255,24.9806935219246)) ;
#115182=CARTESIAN_POINT('Ctrl Pts',(58.4790182134328,247.964376111971,24.9833532460141)) ;
#115183=CARTESIAN_POINT('Ctrl Pts',(58.4762260371539,248.033037787681,24.9860089943526)) ;
#115184=CARTESIAN_POINT('Ctrl Pts',(58.473433860875,248.101944538866,24.9850602573903)) ;
#115185=CARTESIAN_POINT('Ctrl Pts',(58.4706416845961,248.170687605668,24.9804839972767)) ;
#115186=CARTESIAN_POINT('Ctrl Pts',(58.4678527624422,248.239350556276,24.975913070538)) ;
#115187=CARTESIAN_POINT('Ctrl Pts',(58.4650638402884,248.307849713925,24.9677230496966)) ;
#115188=CARTESIAN_POINT('Ctrl Pts',(58.4622749181345,248.375776108533,24.9559429471642)) ;
#115189=CARTESIAN_POINT('Ctrl Pts',(58.4594877262922,248.44366036004,24.9441701532789)) ;
#115190=CARTESIAN_POINT('Ctrl Pts',(58.4567005344499,248.510972070924,24.9288117800453)) ;
#115191=CARTESIAN_POINT('Ctrl Pts',(58.4539133426076,248.577308734089,24.9099485212185)) ;
#115192=CARTESIAN_POINT('Ctrl Pts',(58.451126928564,248.643626885226,24.8910905264064)) ;
#115193=CARTESIAN_POINT('Ctrl Pts',(58.4483405145204,248.708970056959,24.8687297219814)) ;
#115194=CARTESIAN_POINT('Ctrl Pts',(58.4455541004769,248.772949017595,24.842997191496)) ;
#115195=CARTESIAN_POINT('Ctrl Pts',(58.4427675128737,248.836931963339,24.8172630581879)) ;
#115196=CARTESIAN_POINT('Ctrl Pts',(58.4399809252705,248.899550074883,24.7881569673943)) ;
#115197=CARTESIAN_POINT('Ctrl Pts',(58.4371943376673,248.960433968837,24.7558581832023)) ;
#115198=CARTESIAN_POINT('Ctrl Pts',(58.4344047991749,249.021382336495,24.7235251958388)) ;
#115199=CARTESIAN_POINT('Ctrl Pts',(58.4316152606825,249.080592387219,24.687992998362)) ;
#115200=CARTESIAN_POINT('Ctrl Pts',(58.4288257221901,249.137720129312,24.6494864056455)) ;
#115201=CARTESIAN_POINT('Ctrl Pts',(58.4260345131964,249.194882082071,24.6109567534454)) ;
#115202=CARTESIAN_POINT('Ctrl Pts',(58.4232433042026,249.249958852386,24.5694494563931)) ;
#115203=CARTESIAN_POINT('Ctrl Pts',(58.4204520952088,249.302638453795,24.5252305088572)) ;
#115204=CARTESIAN_POINT('Ctrl Pts',(58.4176561208302,249.355407994215,24.4809360670453)) ;
#115205=CARTESIAN_POINT('Ctrl Pts',(58.4148601464515,249.405771839137,24.4339210698719)) ;
#115206=CARTESIAN_POINT('Ctrl Pts',(58.4120641720729,249.453454504378,24.3844887041671)) ;
#115207=CARTESIAN_POINT('Ctrl Pts',(58.4108037267986,249.474950191366,24.3622042396784)) ;
#115208=CARTESIAN_POINT('Ctrl Pts',(58.4095432815242,249.495901534199,24.3394289500331)) ;
#115209=CARTESIAN_POINT('Ctrl Pts',(58.4082828362499,249.516286078954,24.3161926703443)) ;
#115210=CARTESIAN_POINT('Ctrl Pts',(58.4055122728199,249.56109300186,24.2651173971337)) ;
#115211=CARTESIAN_POINT('Ctrl Pts',(58.40274170939,249.603342138574,24.2116035703064)) ;
#115212=CARTESIAN_POINT('Ctrl Pts',(58.3999711459601,249.642753907238,24.1559400585432)) ;
#115213=CARTESIAN_POINT('Ctrl Pts',(58.3972044286694,249.682110963872,24.1003538197341)) ;
#115214=CARTESIAN_POINT('Ctrl Pts',(58.3944377113788,249.718638173866,24.0426242158972)) ;
#115215=CARTESIAN_POINT('Ctrl Pts',(58.3916709940882,249.752094809022,23.9830746385671)) ;
#115216=CARTESIAN_POINT('Ctrl Pts',(58.3889071300701,249.785516940869,23.9235864737921)) ;
#115217=CARTESIAN_POINT('Ctrl Pts',(58.3861432660521,249.815874533976,23.8622824917599)) ;
#115218=CARTESIAN_POINT('Ctrl Pts',(58.3833794020341,249.842970083777,23.7995150618265)) ;
#115219=CARTESIAN_POINT('Ctrl Pts',(58.3806168005465,249.870053256357,23.7367763039944)) ;
#115220=CARTESIAN_POINT('Ctrl Pts',(58.3778541990589,249.893877133095,23.6725758783721)) ;
#115221=CARTESIAN_POINT('Ctrl Pts',(58.3750915975712,249.914290896923,23.6072892775912)) ;
#115222=CARTESIAN_POINT('Ctrl Pts',(58.3723298784158,249.93469814091,23.5420235283397)) ;
#115223=CARTESIAN_POINT('Ctrl Pts',(58.3695681592603,249.951697288545,23.4756727715741)) ;
#115224=CARTESIAN_POINT('Ctrl Pts',(58.3668064401048,249.965187020979,23.4086288486433)) ;
#115225=CARTESIAN_POINT('Ctrl Pts',(58.3640429993408,249.978685162682,23.341543131676)) ;
#115226=CARTESIAN_POINT('Ctrl Pts',(58.3612795585768,249.988669418579,23.2737638768196)) ;
#115227=CARTESIAN_POINT('Ctrl Pts',(58.3585161178127,249.995089633367,23.2056931294797)) ;
#115228=CARTESIAN_POINT('Ctrl Pts',(58.3560033747606,250.000927410066,23.1437977200838)) ;
#115229=CARTESIAN_POINT('Ctrl Pts',(58.3534906317085,250.003819081637,23.0816616940208)) ;
#115230=CARTESIAN_POINT('Ctrl Pts',(58.3509778886564,250.003764344365,23.0195888835014)) ;
#115231=CARTESIAN_POINT('',(57.9402651077866,248.892933365216,24.7900173477895)) ;
#115232=CARTESIAN_POINT('Ctrl Pts',(58.3509778886279,250.003764344364,23.019588882796)) ;
#115233=CARTESIAN_POINT('Ctrl Pts',(58.347531931365,250.003689278043,22.9344626889131)) ;
#115234=CARTESIAN_POINT('Ctrl Pts',(58.3440859741021,249.998074586572,22.8495796685279)) ;
#115235=CARTESIAN_POINT('Ctrl Pts',(58.3406400168393,249.987036956171,22.7655633879631)) ;
#115236=CARTESIAN_POINT('Ctrl Pts',(58.3371336303593,249.975805766967,22.6800737757032)) ;
#115237=CARTESIAN_POINT('Ctrl Pts',(58.3336272438794,249.95895981642,22.5954814373205)) ;
#115238=CARTESIAN_POINT('Ctrl Pts',(58.3301208573995,249.936670483819,22.5124206483804)) ;
#115239=CARTESIAN_POINT('Ctrl Pts',(58.3298000350211,249.934631086069,22.5048208700867)) ;
#115240=CARTESIAN_POINT('Ctrl Pts',(58.3294792126427,249.932546151232,22.4972338987649)) ;
#115241=CARTESIAN_POINT('Ctrl Pts',(58.3291583902643,249.930415830371,22.4896602116041)) ;
#115242=CARTESIAN_POINT('Ctrl Pts',(58.3263616510593,249.911844956662,22.423637299127)) ;
#115243=CARTESIAN_POINT('Ctrl Pts',(58.3235649118542,249.889774292161,22.3584592623116)) ;
#115244=CARTESIAN_POINT('Ctrl Pts',(58.3207681726492,249.864298716166,22.2945235043388)) ;
#115245=CARTESIAN_POINT('Ctrl Pts',(58.3179756150477,249.838861230515,22.2306833412612)) ;
#115246=CARTESIAN_POINT('Ctrl Pts',(58.3151830574462,249.810029117849,22.1680822227063)) ;
#115247=CARTESIAN_POINT('Ctrl Pts',(58.3123904998447,249.777947242342,22.1071031651792)) ;
#115248=CARTESIAN_POINT('Ctrl Pts',(58.3096012005832,249.745902799781,22.0461952576638)) ;
#115249=CARTESIAN_POINT('Ctrl Pts',(58.3068119013218,249.710616352775,21.986906084436)) ;
#115250=CARTESIAN_POINT('Ctrl Pts',(58.3040226020603,249.67228042168,21.9295977298812)) ;
#115251=CARTESIAN_POINT('Ctrl Pts',(58.3012350359522,249.633968310921,21.8723249843298)) ;
#115252=CARTESIAN_POINT('Ctrl Pts',(58.2984474698442,249.592610747277,21.8170310227065)) ;
#115253=CARTESIAN_POINT('Ctrl Pts',(58.2956599037361,249.548444863234,21.7640510505049)) ;
#115254=CARTESIAN_POINT('Ctrl Pts',(58.2928731188216,249.504291356334,21.7110859255261)) ;
#115255=CARTESIAN_POINT('Ctrl Pts',(58.2900863339071,249.457331405552,21.6604338792422)) ;
#115256=CARTESIAN_POINT('Ctrl Pts',(58.2872995489926,249.40784281188,21.6123975375607)) ;
#115257=CARTESIAN_POINT('Ctrl Pts',(58.2845125944698,249.358351206252,21.5643582723083)) ;
#115258=CARTESIAN_POINT('Ctrl Pts',(58.281725639947,249.306331006061,21.5189353676264)) ;
#115259=CARTESIAN_POINT('Ctrl Pts',(58.2789386854242,249.252095996024,21.4763937600894)) ;
#115260=CARTESIAN_POINT('Ctrl Pts',(58.2761487884291,249.197803724553,21.433807237037)) ;
#115261=CARTESIAN_POINT('Ctrl Pts',(58.2733588914341,249.141292363387,21.3941083854731)) ;
#115262=CARTESIAN_POINT('Ctrl Pts',(58.270568994439,249.082907028509,21.3575204532029)) ;
#115263=CARTESIAN_POINT('Ctrl Pts',(58.2677774312452,249.024486824397,21.320910669672)) ;
#115264=CARTESIAN_POINT('Ctrl Pts',(58.2649858680514,248.964190848044,21.2874157415453)) ;
#115265=CARTESIAN_POINT('Ctrl Pts',(58.2621943048577,248.902388871569,21.2572129585288)) ;
#115266=CARTESIAN_POINT('Ctrl Pts',(58.2593979865201,248.840481621717,21.2269587281453)) ;
#115267=CARTESIAN_POINT('Ctrl Pts',(58.2566016681825,248.777063703201,21.2000080267488)) ;
#115268=CARTESIAN_POINT('Ctrl Pts',(58.2538053498449,248.712524075554,21.1764896927257)) ;
#115269=CARTESIAN_POINT('Ctrl Pts',(58.2525482146562,248.68350912547,21.1659166027871)) ;
#115270=CARTESIAN_POINT('Ctrl Pts',(58.2512910794675,248.654267654608,21.1560365562948)) ;
#115271=CARTESIAN_POINT('Ctrl Pts',(58.2500339442788,248.62483575027,21.1468579102349)) ;
#115272=CARTESIAN_POINT('Ctrl Pts',(58.2472375760956,248.559367500237,21.1264409542565)) ;
#115273=CARTESIAN_POINT('Ctrl Pts',(58.2444412079124,248.49270009251,21.109417978687)) ;
#115274=CARTESIAN_POINT('Ctrl Pts',(58.2416448397292,248.425218349744,21.0959260329037)) ;
#115275=CARTESIAN_POINT('Ctrl Pts',(58.2388526472344,248.357837374371,21.0824542340247)) ;
#115276=CARTESIAN_POINT('Ctrl Pts',(58.2360604547397,248.289644954913,21.0725030953405)) ;
#115277=CARTESIAN_POINT('Ctrl Pts',(58.2332682622449,248.221041097842,21.0661599175538)) ;
#115278=CARTESIAN_POINT('Ctrl Pts',(58.230479317708,248.152517042732,21.0598241183322)) ;
#115279=CARTESIAN_POINT('Ctrl Pts',(58.227690373171,248.083582986998,21.0570879895587)) ;
#115280=CARTESIAN_POINT('Ctrl Pts',(58.2249014286341,248.014647364114,21.0579874677565)) ;
#115281=CARTESIAN_POINT('Ctrl Pts',(58.2221142106069,247.945754416166,21.058886389128)) ;
#115282=CARTESIAN_POINT('Ctrl Pts',(58.2193269925798,247.876860392677,21.0634164462515)) ;
#115283=CARTESIAN_POINT('Ctrl Pts',(58.2165397745527,247.808375505614,21.0715615219602)) ;
#115284=CARTESIAN_POINT('Ctrl Pts',(58.2137533306026,247.739909638441,21.0797043355868)) ;
#115285=CARTESIAN_POINT('Ctrl Pts',(58.2109668866525,247.671853169254,21.0914601166436)) ;
#115286=CARTESIAN_POINT('Ctrl Pts',(58.2081804427024,247.604611157847,21.1067608939988)) ;
#115287=CARTESIAN_POINT('Ctrl Pts',(58.2053938215471,247.537364870154,21.122062644414)) ;
#115288=CARTESIAN_POINT('Ctrl Pts',(58.2026072003918,247.470933621065,21.1409097273127)) ;
#115289=CARTESIAN_POINT('Ctrl Pts',(58.1998205792366,247.405710479151,21.1631834612825)) ;
#115290=CARTESIAN_POINT('Ctrl Pts',(58.1970310020144,247.340418148081,21.1854808233821)) ;
#115291=CARTESIAN_POINT('Ctrl Pts',(58.1942414247923,247.276336947073,21.2112119318301)) ;
#115292=CARTESIAN_POINT('Ctrl Pts',(58.1914518475702,247.21384206527,21.2402091160393)) ;
#115293=CARTESIAN_POINT('Ctrl Pts',(58.1886605968347,247.151309691755,21.2692236961382)) ;
#115294=CARTESIAN_POINT('Ctrl Pts',(58.1858693460991,247.090365965219,21.3015080218526)) ;
#115295=CARTESIAN_POINT('Ctrl Pts',(58.1830780953635,247.031360973862,21.3368487057601)) ;
#115296=CARTESIAN_POINT('Ctrl Pts',(58.1802820751297,246.972255158811,21.372249777411)) ;
#115297=CARTESIAN_POINT('Ctrl Pts',(58.1774860548958,246.915095097436,21.4107173563645)) ;
#115298=CARTESIAN_POINT('Ctrl Pts',(58.1746900346619,246.860200707424,21.4519955648736)) ;
#115299=CARTESIAN_POINT('Ctrl Pts',(58.1734298558723,246.835459561019,21.4705998375473)) ;
#115300=CARTESIAN_POINT('Ctrl Pts',(58.1721696770828,246.811178184421,21.4897745163459)) ;
#115301=CARTESIAN_POINT('Ctrl Pts',(58.1709094982933,246.787383444121,21.5094937044066)) ;
#115302=CARTESIAN_POINT('Ctrl Pts',(58.1681151052984,246.734619617146,21.5532201672229)) ;
#115303=CARTESIAN_POINT('Ctrl Pts',(58.1653207123035,246.684043271349,21.5997987073911)) ;
#115304=CARTESIAN_POINT('Ctrl Pts',(58.1625263193086,246.63597889751,21.6489820144193)) ;
#115305=CARTESIAN_POINT('Ctrl Pts',(58.1597361135886,246.587986546018,21.6980916224268)) ;
#115306=CARTESIAN_POINT('Ctrl Pts',(58.1569459078686,246.542499036916,21.7497979021576)) ;
#115307=CARTESIAN_POINT('Ctrl Pts',(58.1541557021486,246.499807471406,21.80381366164)) ;
#115308=CARTESIAN_POINT('Ctrl Pts',(58.1513687516734,246.457165712795,21.8577664026454)) ;
#115309=CARTESIAN_POINT('Ctrl Pts',(58.1485818011981,246.417313722939,21.9140228884521)) ;
#115310=CARTESIAN_POINT('Ctrl Pts',(58.1457948507228,246.380504163978,21.9722608317058)) ;
#115311=CARTESIAN_POINT('Ctrl Pts',(58.1430096300917,246.3437174525,22.0304626270022)) ;
#115312=CARTESIAN_POINT('Ctrl Pts',(58.1402244094606,246.30996968794,22.090643025414)) ;
#115313=CARTESIAN_POINT('Ctrl Pts',(58.1374391888295,246.27947088064,22.152449847082)) ;
#115314=CARTESIAN_POINT('Ctrl Pts',(58.1346547425464,246.24898055263,22.2142394851943)) ;
#115315=CARTESIAN_POINT('Ctrl Pts',(58.1318702962634,246.221737606122,22.2776542082484)) ;
#115316=CARTESIAN_POINT('Ctrl Pts',(58.1290858499804,246.197905780348,22.3423178703659)) ;
#115317=CARTESIAN_POINT('Ctrl Pts',(58.1263012237015,246.174072414006,22.4069857125577)) ;
#115318=CARTESIAN_POINT('Ctrl Pts',(58.1235165974226,246.153650773739,22.4729021919415)) ;
#115319=CARTESIAN_POINT('Ctrl Pts',(58.1207319711437,246.136755552144,22.5396735626319)) ;
#115320=CARTESIAN_POINT('Ctrl Pts',(58.1179443709375,246.119842286777,22.6065162438617)) ;
#115321=CARTESIAN_POINT('Ctrl Pts',(58.1151567707312,246.106463076697,22.67421516094)) ;
#115322=CARTESIAN_POINT('Ctrl Pts',(58.112369170525,246.096681798163,22.7423648479079)) ;
#115323=CARTESIAN_POINT('Ctrl Pts',(58.109579889445,246.08689462169,22.8105556279367)) ;
#115324=CARTESIAN_POINT('Ctrl Pts',(58.106790608365,246.080709738345,22.879197229136)) ;
#115325=CARTESIAN_POINT('Ctrl Pts',(58.104001327285,246.078139012731,22.9478803197007)) ;
#115326=CARTESIAN_POINT('Ctrl Pts',(58.1012072448587,246.075563861983,23.0166816383284)) ;
#115327=CARTESIAN_POINT('Ctrl Pts',(58.0984131624324,246.076615277465,23.0855240976552)) ;
#115328=CARTESIAN_POINT('Ctrl Pts',(58.0956190800061,246.081253054944,23.1540005109516)) ;
#115329=CARTESIAN_POINT('Ctrl Pts',(58.0943410707733,246.083374367609,23.1853215226719)) ;
#115330=CARTESIAN_POINT('Ctrl Pts',(58.0930630615406,246.086245281554,23.2165660568276)) ;
#115331=CARTESIAN_POINT('Ctrl Pts',(58.0917850523078,246.089858388485,23.2476958707352)) ;
#115332=CARTESIAN_POINT('Ctrl Pts',(58.0889844571912,246.097776053995,23.3159129090573)) ;
#115333=CARTESIAN_POINT('Ctrl Pts',(58.0861838620747,246.109292215792,23.3838458349369)) ;
#115334=CARTESIAN_POINT('Ctrl Pts',(58.0833832669581,246.124375389261,23.4510863687974)) ;
#115335=CARTESIAN_POINT('Ctrl Pts',(58.0805868570181,246.139436022612,23.5182264191906)) ;
#115336=CARTESIAN_POINT('Ctrl Pts',(58.0777904470782,246.158052980711,23.584675657751)) ;
#115337=CARTESIAN_POINT('Ctrl Pts',(58.0749940371382,246.180143156851,23.6500321834753)) ;
#115338=CARTESIAN_POINT('Ctrl Pts',(58.0722009096359,246.20220740345,23.7153119934366)) ;
#115339=CARTESIAN_POINT('Ctrl Pts',(58.0694077821336,246.227736614132,23.7795011769888)) ;
#115340=CARTESIAN_POINT('Ctrl Pts',(58.0666146546313,246.256597332155,23.8422110282283)) ;
#115341=CARTESIAN_POINT('Ctrl Pts',(58.0638232776877,246.285439962074,23.9048815768318)) ;
#115342=CARTESIAN_POINT('Ctrl Pts',(58.0610319007441,246.317609752663,23.9660741892134)) ;
#115343=CARTESIAN_POINT('Ctrl Pts',(58.0582405238005,246.352924961368,24.0254196814177)) ;
#115344=CARTESIAN_POINT('Ctrl Pts',(58.0554499512619,246.388229993113,24.0847480717338)) ;
#115345=CARTESIAN_POINT('Ctrl Pts',(58.0526593787234,246.426678393208,24.1422299785625)) ;
#115346=CARTESIAN_POINT('Ctrl Pts',(58.0498688061849,246.468043120542,24.1975219728842)) ;
#115347=CARTESIAN_POINT('Ctrl Pts',(58.0470780930781,246.509409931522,24.2528167524048)) ;
#115348=CARTESIAN_POINT('Ctrl Pts',(58.0442873799713,246.553693066345,24.3059210102196)) ;
#115349=CARTESIAN_POINT('Ctrl Pts',(58.0414966668645,246.600623992847,24.3565228413767)) ;
#115350=CARTESIAN_POINT('Ctrl Pts',(58.0387030804571,246.647603239136,24.4071767718607)) ;
#115351=CARTESIAN_POINT('Ctrl Pts',(58.0359094940496,246.697235384496,24.4553227743831)) ;
#115352=CARTESIAN_POINT('Ctrl Pts',(58.0331159076422,246.749214363596,24.500685148443)) ;
#115353=CARTESIAN_POINT('Ctrl Pts',(58.0303206895187,246.801223703288,24.5460740183772)) ;
#115354=CARTESIAN_POINT('Ctrl Pts',(58.0275254713952,246.855582220368,24.5886757213844)) ;
#115355=CARTESIAN_POINT('Ctrl Pts',(58.0247302532716,246.911952202286,24.6282560103748)) ;
#115356=CARTESIAN_POINT('Ctrl Pts',(58.0219303703382,246.968416257455,24.6679023530748)) ;
#115357=CARTESIAN_POINT('Ctrl Pts',(58.0191304874047,247.026898062941,24.7045169583855)) ;
#115358=CARTESIAN_POINT('Ctrl Pts',(58.0163306044712,247.087033262235,24.7379103641024)) ;
#115359=CARTESIAN_POINT('Ctrl Pts',(58.0151072717549,247.113307702434,24.7525007047326)) ;
#115360=CARTESIAN_POINT('Ctrl Pts',(58.0138839390385,247.139897496379,24.7664767247963)) ;
#115361=CARTESIAN_POINT('Ctrl Pts',(58.0126606063222,247.166771094637,24.7798255209739)) ;
#115362=CARTESIAN_POINT('Ctrl Pts',(58.0098986862272,247.227443657434,24.8099631179776)) ;
#115363=CARTESIAN_POINT('Ctrl Pts',(58.0071367661322,247.2898098171,24.8370223835677)) ;
#115364=CARTESIAN_POINT('Ctrl Pts',(58.0043748460373,247.353520461229,24.8608077831538)) ;
#115365=CARTESIAN_POINT('Ctrl Pts',(58.0016175292885,247.417124917582,24.8845535391494)) ;
#115366=CARTESIAN_POINT('Ctrl Pts',(57.9988602125398,247.482068941796,24.9050360866091)) ;
#115367=CARTESIAN_POINT('Ctrl Pts',(57.996102895791,247.547980335786,24.922106484412)) ;
#115368=CARTESIAN_POINT('Ctrl Pts',(57.9933481370867,247.613830581823,24.9391610455012)) ;
#115369=CARTESIAN_POINT('Ctrl Pts',(57.9905933783824,247.680645933727,24.9528096041868)) ;
#115370=CARTESIAN_POINT('Ctrl Pts',(57.9878386196781,247.748037235499,24.9629524201021)) ;
#115371=CARTESIAN_POINT('Ctrl Pts',(57.9850854200319,247.815390397105,24.9730894956817)) ;
#115372=CARTESIAN_POINT('Ctrl Pts',(57.9823322203858,247.883318364787,24.9797246873835)) ;
#115373=CARTESIAN_POINT('Ctrl Pts',(57.9795790207396,247.951421880769,24.982809352199)) ;
#115374=CARTESIAN_POINT('Ctrl Pts',(57.9768263833758,248.019511488059,24.9858933870375)) ;
#115375=CARTESIAN_POINT('Ctrl Pts',(57.9740737460121,248.087776069018,24.985428312288)) ;
#115376=CARTESIAN_POINT('Ctrl Pts',(57.9713211086483,248.155813320873,24.9814174994303)) ;
#115377=CARTESIAN_POINT('Ctrl Pts',(57.9685662598804,248.223905232256,24.9774034643798)) ;
#115378=CARTESIAN_POINT('Ctrl Pts',(57.9658114111125,248.291768945337,24.969838029674)) ;
#115379=CARTESIAN_POINT('Ctrl Pts',(57.9630565623445,248.35900545855,24.9587766240456)) ;
#115380=CARTESIAN_POINT('Ctrl Pts',(57.9603006131048,248.426268830547,24.9477107997481)) ;
#115381=CARTESIAN_POINT('Ctrl Pts',(57.9575446638651,248.492904010497,24.9331463308006)) ;
#115382=CARTESIAN_POINT('Ctrl Pts',(57.9547887146254,248.558523270173,24.9151895911899)) ;
#115383=CARTESIAN_POINT('Ctrl Pts',(57.9520281095573,248.624253385304,24.8972025159342)) ;
#115384=CARTESIAN_POINT('Ctrl Pts',(57.9492675044892,248.688963673453,24.875811884145)) ;
#115385=CARTESIAN_POINT('Ctrl Pts',(57.9465068994212,248.752283471603,24.8511733703317)) ;
#115386=CARTESIAN_POINT('Ctrl Pts',(57.9444263022096,248.800005978886,24.8326039546159)) ;
#115387=CARTESIAN_POINT('Ctrl Pts',(57.9423457049981,248.84693900529,24.8121906938376)) ;
#115388=CARTESIAN_POINT('Ctrl Pts',(57.9402651077866,248.892933365216,24.7900173477895)) ;
#115389=CARTESIAN_POINT('Ctrl Pts',(57.9402651077866,248.892933365216,24.7900173477895)) ;
#115390=CARTESIAN_POINT('Ctrl Pts',(57.9402651077866,248.907470247387,24.7827857167614)) ;
#115391=CARTESIAN_POINT('Ctrl Pts',(57.9402651077866,248.922007129558,24.7755540857334)) ;
#115392=CARTESIAN_POINT('Ctrl Pts',(57.9402651077866,248.936544011728,24.7683224547054)) ;
#115393=CARTESIAN_POINT('',(55.9402651077866,250.003765107786,23.0213203435596)) ;
#115394=CARTESIAN_POINT('Origin',(55.9402651077866,248.040265107786,23.0213203435596)) ;
#115395=CARTESIAN_POINT('Origin',(61.8645744874958,248.040265107786,23.0213203435596)) ;
#115396=CARTESIAN_POINT('',(57.9402651077867,247.09020061484,21.6384890010805)) ;
#115397=CARTESIAN_POINT('Ctrl Pts',(58.2783798877068,247.272019130299,24.5128441216388)) ;
#115398=CARTESIAN_POINT('Ctrl Pts',(58.2748979901455,247.332077509349,24.5437786657587)) ;
#115399=CARTESIAN_POINT('Ctrl Pts',(58.271320587604,247.393976935328,24.5710716276367)) ;
#115400=CARTESIAN_POINT('Ctrl Pts',(58.2627451136209,247.545035169529,24.627038133204)) ;
#115401=CARTESIAN_POINT('Ctrl Pts',(58.2577412103424,247.635251058642,24.6521323366216)) ;
#115402=CARTESIAN_POINT('Ctrl Pts',(58.2520375966099,247.746374322123,24.6732460496859)) ;
#115403=CARTESIAN_POINT('Ctrl Pts',(58.2510614554046,247.765721207416,24.6765713936764)) ;
#115404=CARTESIAN_POINT('Ctrl Pts',(58.2495470185004,247.796358451649,24.6812853540765)) ;
#115405=CARTESIAN_POINT('Ctrl Pts',(58.2489973964822,247.807611769283,24.6828999325575)) ;
#115406=CARTESIAN_POINT('Ctrl Pts',(58.2479269228372,247.82982153336,24.6858564298797)) ;
#115407=CARTESIAN_POINT('Ctrl Pts',(58.2474057836264,247.840776417959,24.6872048386251)) ;
#115408=CARTESIAN_POINT('Ctrl Pts',(58.2460500620374,247.869616457428,24.6904661162285)) ;
#115409=CARTESIAN_POINT('Ctrl Pts',(58.2452247764834,247.887520895965,24.6921996997116)) ;
#115410=CARTESIAN_POINT('Ctrl Pts',(58.2406147555242,247.989179322784,24.7003949117824)) ;
#115411=CARTESIAN_POINT('Ctrl Pts',(58.2370870272144,248.073304410782,24.7008476342292)) ;
#115412=CARTESIAN_POINT('Ctrl Pts',(58.2287463145611,248.272606508734,24.6869330955302)) ;
#115413=CARTESIAN_POINT('Ctrl Pts',(58.2239556977729,248.386951254969,24.666937377997)) ;
#115414=CARTESIAN_POINT('Ctrl Pts',(58.2174797274263,248.526774465455,24.6272557885101)) ;
#115415=CARTESIAN_POINT('Ctrl Pts',(58.2161407395415,248.555010573944,24.618429292159)) ;
#115416=CARTESIAN_POINT('Ctrl Pts',(58.2138873395185,248.601282287633,24.6026103821848)) ;
#115417=CARTESIAN_POINT('Ctrl Pts',(58.2129868720803,248.619457016907,24.5960441790141)) ;
#115418=CARTESIAN_POINT('Ctrl Pts',(58.211176412634,248.655345786747,24.5823728542874)) ;
#115419=CARTESIAN_POINT('Ctrl Pts',(58.2102668150887,248.673060055623,24.5752764884306)) ;
#115420=CARTESIAN_POINT('Ctrl Pts',(58.2079855305723,248.716687486869,24.5569295826173)) ;
#115421=CARTESIAN_POINT('Ctrl Pts',(58.2066020787698,248.742444209569,24.5453240706538)) ;
#115422=CARTESIAN_POINT('Ctrl Pts',(58.2035397571162,248.797939511295,24.5186133560451)) ;
#115423=CARTESIAN_POINT('Ctrl Pts',(58.2018532644446,248.827545110282,24.5032605867735)) ;
#115424=CARTESIAN_POINT('Ctrl Pts',(58.1964360981523,248.919771472909,24.4518902846567)) ;
#115425=CARTESIAN_POINT('Ctrl Pts',(58.1926171847178,248.980531233698,24.4127082157092)) ;
#115426=CARTESIAN_POINT('Ctrl Pts',(58.1837372591114,249.114597859774,24.3134510911288)) ;
#115427=CARTESIAN_POINT('Ctrl Pts',(58.1786702794447,249.185729624582,24.2508347284892)) ;
#115428=CARTESIAN_POINT('Ctrl Pts',(58.1729178114678,249.264707236925,24.1684763816803)) ;
#115429=CARTESIAN_POINT('Ctrl Pts',(58.1719480002254,249.277961319081,24.1541635148172)) ;
#115430=CARTESIAN_POINT('Ctrl Pts',(58.1704413246273,249.298519479715,24.1311714641225)) ;
#115431=CARTESIAN_POINT('Ctrl Pts',(58.1698932954084,249.305990030728,24.1226440957261)) ;
#115432=CARTESIAN_POINT('Ctrl Pts',(58.168827411681,249.32052174376,24.1057134721195)) ;
#115433=CARTESIAN_POINT('Ctrl Pts',(58.168309261345,249.327587902867,24.0973154820613)) ;
#115434=CARTESIAN_POINT('Ctrl Pts',(58.1669608589769,249.345957850368,24.0750431585538)) ;
#115435=CARTESIAN_POINT('Ctrl Pts',(58.1661398787163,249.357123244922,24.0610558868507)) ;
#115436=CARTESIAN_POINT('Ctrl Pts',(58.1615902604397,249.418663666299,23.9813800957598)) ;
#115437=CARTESIAN_POINT('Ctrl Pts',(58.1581133955458,249.464350905108,23.9122071198179)) ;
#115438=CARTESIAN_POINT('Ctrl Pts',(58.1497133261122,249.562639591519,23.7363718607849)) ;
#115439=CARTESIAN_POINT('Ctrl Pts',(58.1448185566736,249.609381217752,23.6269569637157)) ;
#115440=CARTESIAN_POINT('Ctrl Pts',(58.1382251156756,249.652798275206,23.4854788705331)) ;
#115441=CARTESIAN_POINT('Ctrl Pts',(58.1368966544137,249.660670299946,23.4572024944238)) ;
#115442=CARTESIAN_POINT('Ctrl Pts',(58.1346592433347,249.672461531608,23.4100991480262)) ;
#115443=CARTESIAN_POINT('Ctrl Pts',(58.133764063552,249.676806062136,23.3913849231925)) ;
#115444=CARTESIAN_POINT('Ctrl Pts',(58.1319634604706,249.684803683137,23.354034121129)) ;
#115445=CARTESIAN_POINT('Ctrl Pts',(58.1310584101892,249.688463610433,23.3354019303104)) ;
#115446=CARTESIAN_POINT('Ctrl Pts',(58.1287878578837,249.696757591018,23.2890301136861)) ;
#115447=CARTESIAN_POINT('Ctrl Pts',(58.1274106257705,249.701011779221,23.261229166923)) ;
#115448=CARTESIAN_POINT('Ctrl Pts',(58.1211474422744,249.716930184925,23.136271055147)) ;
#115449=CARTESIAN_POINT('Ctrl Pts',(58.116026325459,249.720778833748,23.0383220310557)) ;
#115450=CARTESIAN_POINT('Ctrl Pts',(58.1053096317472,249.711084330988,22.8370403410001)) ;
#115451=CARTESIAN_POINT('Ctrl Pts',(58.0997283898167,249.696506013282,22.7341548738862)) ;
#115452=CARTESIAN_POINT('Ctrl Pts',(58.0935609702691,249.668167456351,22.6149541822122)) ;
#115453=CARTESIAN_POINT('Ctrl Pts',(58.0926260918652,249.663504790088,22.5967116992631)) ;
#115454=CARTESIAN_POINT('Ctrl Pts',(58.0911615920557,249.655586213827,22.5677702245165)) ;
#115455=CARTESIAN_POINT('Ctrl Pts',(58.0906217053732,249.652528797081,22.5570189341692)) ;
#115456=CARTESIAN_POINT('Ctrl Pts',(58.0895529908071,249.646190233062,22.5355475427917)) ;
#115457=CARTESIAN_POINT('Ctrl Pts',(58.089024191361,249.64290865212,22.5248282444628)) ;
#115458=CARTESIAN_POINT('Ctrl Pts',(58.0876284254771,249.633866577783,22.496316399195)) ;
#115459=CARTESIAN_POINT('Ctrl Pts',(58.08677169367,249.627915504649,22.4785855522774)) ;
#115460=CARTESIAN_POINT('Ctrl Pts',(58.0815853579806,249.589520970401,22.3702321063645)) ;
#115461=CARTESIAN_POINT('Ctrl Pts',(58.0775885480795,249.549622248674,22.2824334260245)) ;
#115462=CARTESIAN_POINT('Ctrl Pts',(58.0693654513875,249.452957056141,22.1106526920531)) ;
#115463=CARTESIAN_POINT('Ctrl Pts',(58.0651478651584,249.395682564177,22.0274109048578)) ;
#115464=CARTESIAN_POINT('Ctrl Pts',(58.0593077990619,249.311859657264,21.9264150970558)) ;
#115465=CARTESIAN_POINT('Ctrl Pts',(58.057932431993,249.291802257686,21.9035436080008)) ;
#115466=CARTESIAN_POINT('Ctrl Pts',(58.0556320097518,249.25785639115,21.8668947867048)) ;
#115467=CARTESIAN_POINT('Ctrl Pts',(58.0547219724047,249.244328748527,21.8527923760427)) ;
#115468=CARTESIAN_POINT('Ctrl Pts',(58.0529028381644,249.217119371765,21.8254011447104)) ;
#115469=CARTESIAN_POINT('Ctrl Pts',(58.05199438389,249.203451236086,21.8121029589124)) ;
#115470=CARTESIAN_POINT('Ctrl Pts',(58.0497360855303,249.169297481163,21.7799885935626)) ;
#115471=CARTESIAN_POINT('Ctrl Pts',(58.048375181623,249.1485654137,21.7614437890237)) ;
#115472=CARTESIAN_POINT('Ctrl Pts',(58.0414723744861,249.042698798655,21.6713821694049)) ;
#115473=CARTESIAN_POINT('Ctrl Pts',(58.0356180024846,248.951073489103,21.6079453898174)) ;
#115474=CARTESIAN_POINT('Ctrl Pts',(58.0249619385237,248.775979976737,21.5108570780169)) ;
#115475=CARTESIAN_POINT('Ctrl Pts',(58.0202073655345,248.694778896838,21.4739389864986)) ;
#115476=CARTESIAN_POINT('Ctrl Pts',(58.0146997007208,248.59213829509,21.4368063633293)) ;
#115477=CARTESIAN_POINT('Ctrl Pts',(58.0137001563191,248.573126993811,21.4303122222319)) ;
#115478=CARTESIAN_POINT('Ctrl Pts',(58.0121563064781,248.543054449113,21.4206391722487)) ;
#115479=CARTESIAN_POINT('Ctrl Pts',(58.0116001012966,248.532069751408,21.4172300904024)) ;
#115480=CARTESIAN_POINT('Ctrl Pts',(58.0105177425053,248.510370249532,21.4107395497992)) ;
#115481=CARTESIAN_POINT('Ctrl Pts',(58.0099912505437,248.49965813027,21.4076514189601)) ;
#115482=CARTESIAN_POINT('Ctrl Pts',(58.0086248640635,248.471479036562,21.3998311922984)) ;
#115483=CARTESIAN_POINT('Ctrl Pts',(58.0077942134424,248.453964504307,21.3952744111645)) ;
#115484=CARTESIAN_POINT('Ctrl Pts',(58.005951466049,248.414373542241,21.3856551050401)) ;
#115485=CARTESIAN_POINT('Ctrl Pts',(58.0049464301702,248.392261256857,21.3807543828688)) ;
#115486=CARTESIAN_POINT('Ctrl Pts',(58.0016621161521,248.318671226203,21.3660011609283)) ;
#115487=CARTESIAN_POINT('Ctrl Pts',(57.9994450969059,248.266829949253,21.3581124851648)) ;
#115488=CARTESIAN_POINT('Ctrl Pts',(57.9920522315695,248.091675339794,21.3398022241462)) ;
#115489=CARTESIAN_POINT('Ctrl Pts',(57.9869451430184,247.967612030511,21.34058648171)) ;
#115490=CARTESIAN_POINT('Ctrl Pts',(57.9801496161107,247.816730852348,21.3582887454584)) ;
#115491=CARTESIAN_POINT('Ctrl Pts',(57.97886791646,247.788787547477,21.3622843005214)) ;
#115492=CARTESIAN_POINT('Ctrl Pts',(57.9767682610458,247.743958274348,21.3698529378715)) ;
#115493=CARTESIAN_POINT('Ctrl Pts',(57.9759640560679,247.727003030229,21.3729850693059)) ;
#115494=CARTESIAN_POINT('Ctrl Pts',(57.9742510932236,247.691363668561,21.3801384466992)) ;
#115495=CARTESIAN_POINT('Ctrl Pts',(57.9733405748524,247.672694031667,21.3842187278339)) ;
#115496=CARTESIAN_POINT('Ctrl Pts',(57.971072575685,247.626884688805,21.3950535390632)) ;
#115497=CARTESIAN_POINT('Ctrl Pts',(57.9697038275137,247.599837049454,21.402169300435)) ;
#115498=CARTESIAN_POINT('Ctrl Pts',(57.9666844118785,247.541471207537,21.4190949980413)) ;
#115499=CARTESIAN_POINT('Ctrl Pts',(57.9650265886409,247.510237800917,21.4291544307489)) ;
#115500=CARTESIAN_POINT('Ctrl Pts',(57.9597702061772,247.41360619379,21.4634353894848)) ;
#115501=CARTESIAN_POINT('Ctrl Pts',(57.956089153945,247.349413117597,21.4908206473135)) ;
#115502=CARTESIAN_POINT('Ctrl Pts',(57.9483128361232,247.218895015048,21.556388768177)) ;
#115503=CARTESIAN_POINT('Ctrl Pts',(57.9442208456806,247.153105283643,21.5952707933102)) ;
#115504=CARTESIAN_POINT('Ctrl Pts',(57.9402651077867,247.09020061484,21.6384890010805)) ;
#115505=CARTESIAN_POINT('',(57.9402651077866,249.01460512908,21.6554848536836)) ;
#115506=CARTESIAN_POINT('Origin',(57.9402651077866,248.040265107786,23.0213203435596)) ;
#115507=CARTESIAN_POINT('',(58.0159557280338,249.718014855353,23.0222406915478)) ;
#115508=CARTESIAN_POINT('Ctrl Pts',(58.0159557280338,249.718014855353,23.0222406915478)) ;
#115509=CARTESIAN_POINT('Ctrl Pts',(58.0130009107869,249.718048781581,22.9603948218142)) ;
#115510=CARTESIAN_POINT('Ctrl Pts',(58.0100460935399,249.71465877968,22.8984282829972)) ;
#115511=CARTESIAN_POINT('Ctrl Pts',(58.007091276293,249.707831191182,22.8367440178679)) ;
#115512=CARTESIAN_POINT('Ctrl Pts',(58.0041427654337,249.701018174625,22.7751914038217)) ;
#115513=CARTESIAN_POINT('Ctrl Pts',(58.0011942545745,249.690782209106,22.7139203500751)) ;
#115514=CARTESIAN_POINT('Ctrl Pts',(57.9982457437152,249.67716158959,22.6533326122993)) ;
#115515=CARTESIAN_POINT('Ctrl Pts',(57.9953008849976,249.663557841109,22.5928199208812)) ;
#115516=CARTESIAN_POINT('Ctrl Pts',(57.99235602628,249.64657786523,22.5329893419975)) ;
#115517=CARTESIAN_POINT('Ctrl Pts',(57.9894111675624,249.626311417612,22.4742351896888)) ;
#115518=CARTESIAN_POINT('Ctrl Pts',(57.9864689847879,249.606063385772,22.4155344262787)) ;
#115519=CARTESIAN_POINT('Ctrl Pts',(57.9835268020133,249.582534970385,22.3579086103247)) ;
#115520=CARTESIAN_POINT('Ctrl Pts',(57.9805846192387,249.555865987917,22.3017378016325)) ;
#115521=CARTESIAN_POINT('Ctrl Pts',(57.9776441397485,249.52921244462,22.2455995112676)) ;
#115522=CARTESIAN_POINT('Ctrl Pts',(57.9747036602584,249.499422156201,22.1909149978639)) ;
#115523=CARTESIAN_POINT('Ctrl Pts',(57.9717631807682,249.466682681607,22.1380435083633)) ;
#115524=CARTESIAN_POINT('Ctrl Pts',(57.9688224013677,249.433939867794,22.0851666263053)) ;
#115525=CARTESIAN_POINT('Ctrl Pts',(57.9658816219672,249.39824751513,22.0341035617204)) ;
#115526=CARTESIAN_POINT('Ctrl Pts',(57.9629408425668,249.359837984726,21.9851869134728)) ;
#115527=CARTESIAN_POINT('Ctrl Pts',(57.9599999943149,249.321427555054,21.9362691199573)) ;
#115528=CARTESIAN_POINT('Ctrl Pts',(57.957059146063,249.280300131595,21.8894982238037)) ;
#115529=CARTESIAN_POINT('Ctrl Pts',(57.9541182978111,249.236728627424,21.8451740479502)) ;
#115530=CARTESIAN_POINT('Ctrl Pts',(57.9511747935572,249.19311777202,21.8008098410945)) ;
#115531=CARTESIAN_POINT('Ctrl Pts',(57.9482312893032,249.147058780088,21.758897110781)) ;
#115532=CARTESIAN_POINT('Ctrl Pts',(57.9452877850493,249.098860870152,21.7196982500162)) ;
#115533=CARTESIAN_POINT('Ctrl Pts',(57.9436135592951,249.0714465452,21.6974024635769)) ;
#115534=CARTESIAN_POINT('Ctrl Pts',(57.9419393335408,249.043340861804,21.6759839362171)) ;
#115535=CARTESIAN_POINT('Ctrl Pts',(57.9402651077866,249.01460512908,21.6554848536836)) ;
#115536=CARTESIAN_POINT('Ctrl Pts',(58.1788076829103,247.272018954284,24.5128440309778)) ;
#115537=CARTESIAN_POINT('Ctrl Pts',(58.1784179371879,247.279284607174,24.5165863851439)) ;
#115538=CARTESIAN_POINT('Ctrl Pts',(58.1780281914655,247.286575747914,24.520274691396)) ;
#115539=CARTESIAN_POINT('Ctrl Pts',(58.1776384457431,247.293891499148,24.5239086101279)) ;
#115540=CARTESIAN_POINT('Ctrl Pts',(58.1747316426243,247.348453864506,24.551011117471)) ;
#115541=CARTESIAN_POINT('Ctrl Pts',(58.1718248395055,247.404604858308,24.5751927161058)) ;
#115542=CARTESIAN_POINT('Ctrl Pts',(58.1689180363866,247.46199958075,24.596266070479)) ;
#115543=CARTESIAN_POINT('Ctrl Pts',(58.1659845348604,247.51992146228,24.6175329794126)) ;
#115544=CARTESIAN_POINT('Ctrl Pts',(58.1630510333342,247.579109603263,24.635633945886)) ;
#115545=CARTESIAN_POINT('Ctrl Pts',(58.160117531808,247.639184487202,24.6504242071275)) ;
#115546=CARTESIAN_POINT('Ctrl Pts',(58.1572184824335,247.698553828976,24.6650407659455)) ;
#115547=CARTESIAN_POINT('Ctrl Pts',(58.1543194330591,247.758788688729,24.6764238394425)) ;
#115548=CARTESIAN_POINT('Ctrl Pts',(58.1514203836846,247.819505594553,24.6844830835875)) ;
#115549=CARTESIAN_POINT('Ctrl Pts',(58.1485230192334,247.8801872118,24.6925376437116)) ;
#115550=CARTESIAN_POINT('Ctrl Pts',(58.1456256547822,247.941349813877,24.697272137706)) ;
#115551=CARTESIAN_POINT('Ctrl Pts',(58.142728290331,248.002600915774,24.6986475242671)) ;
#115552=CARTESIAN_POINT('Ctrl Pts',(58.1398315368371,248.063839101863,24.7000226208051)) ;
#115553=CARTESIAN_POINT('Ctrl Pts',(58.1369347833431,248.125165239899,24.698040004807)) ;
#115554=CARTESIAN_POINT('Ctrl Pts',(58.1340380298492,248.186185009511,24.6927127106537)) ;
#115555=CARTESIAN_POINT('Ctrl Pts',(58.1310776940082,248.248544133741,24.687268484954)) ;
#115556=CARTESIAN_POINT('Ctrl Pts',(58.1281173581673,248.310582723376,24.6783310047208)) ;
#115557=CARTESIAN_POINT('Ctrl Pts',(58.1251570223263,248.371885976444,24.6659700515431)) ;
#115558=CARTESIAN_POINT('Ctrl Pts',(58.1222563924866,248.431952825165,24.653858402203)) ;
#115559=CARTESIAN_POINT('Ctrl Pts',(58.1193557626468,248.491313236416,24.6384603002759)) ;
#115560=CARTESIAN_POINT('Ctrl Pts',(58.1164551328071,248.549590391702,24.6198924619402)) ;
#115561=CARTESIAN_POINT('Ctrl Pts',(58.1134649439655,248.609666895456,24.6007513284376)) ;
#115562=CARTESIAN_POINT('Ctrl Pts',(58.110474755124,248.668591588852,24.5782416766697)) ;
#115563=CARTESIAN_POINT('Ctrl Pts',(58.1074845662824,248.725974522,24.5525445798354)) ;
#115564=CARTESIAN_POINT('Ctrl Pts',(58.1044943774408,248.783357455147,24.5268474830012)) ;
#115565=CARTESIAN_POINT('Ctrl Pts',(58.1015041885992,248.839198140224,24.4979632754152)) ;
#115566=CARTESIAN_POINT('Ctrl Pts',(58.0985139997577,248.893137479031,24.4661226763606)) ;
#115567=CARTESIAN_POINT('Ctrl Pts',(58.0956224023982,248.945298348437,24.4353319146303)) ;
#115568=CARTESIAN_POINT('Ctrl Pts',(58.0927308050388,248.995903687477,24.4016453930233)) ;
#115569=CARTESIAN_POINT('Ctrl Pts',(58.0898392076793,249.044610396575,24.3652457891802)) ;
#115570=CARTESIAN_POINT('Ctrl Pts',(58.0869038054332,249.094054964928,24.328294766753)) ;
#115571=CARTESIAN_POINT('Ctrl Pts',(58.083968403187,249.14154238529,24.2885479614825)) ;
#115572=CARTESIAN_POINT('Ctrl Pts',(58.0810330009409,249.186740289614,24.246244716716)) ;
#115573=CARTESIAN_POINT('Ctrl Pts',(58.0781493250111,249.231141737132,24.2046869203877)) ;
#115574=CARTESIAN_POINT('Ctrl Pts',(58.0752656490813,249.273333311625,24.1606624209357)) ;
#115575=CARTESIAN_POINT('Ctrl Pts',(58.0723819731514,249.313031776829,24.1144397646084)) ;
#115576=CARTESIAN_POINT('Ctrl Pts',(58.0695000032287,249.352706756084,24.0682444539963)) ;
#115577=CARTESIAN_POINT('Ctrl Pts',(58.066618033306,249.389891212695,24.0198539555883)) ;
#115578=CARTESIAN_POINT('Ctrl Pts',(58.0637360633833,249.424339861513,23.9695724928302)) ;
#115579=CARTESIAN_POINT('Ctrl Pts',(58.0608547006152,249.458781252914,23.9193016230424)) ;
#115580=CARTESIAN_POINT('Ctrl Pts',(58.0579733378471,249.490487688015,23.8671410062943)) ;
#115581=CARTESIAN_POINT('Ctrl Pts',(58.055091975079,249.51925646722,23.8134248955086)) ;
#115582=CARTESIAN_POINT('Ctrl Pts',(58.0521167733035,249.548962175894,23.7579593810805)) ;
#115583=CARTESIAN_POINT('Ctrl Pts',(58.0491415715279,249.57553523724,23.7008357853397)) ;
#115584=CARTESIAN_POINT('Ctrl Pts',(58.0461663697523,249.598804484298,23.6424484095493)) ;
#115585=CARTESIAN_POINT('Ctrl Pts',(58.0432809417461,249.621371604854,23.5858228150443)) ;
#115586=CARTESIAN_POINT('Ctrl Pts',(58.0403955137399,249.640831383414,23.5280091627858)) ;
#115587=CARTESIAN_POINT('Ctrl Pts',(58.0375100857337,249.657078109145,23.4693837108818)) ;
#115588=CARTESIAN_POINT('Ctrl Pts',(58.0344899970734,249.674083056779,23.4080222552788)) ;
#115589=CARTESIAN_POINT('Ctrl Pts',(58.0314699084132,249.687567524432,23.345771987281)) ;
#115590=CARTESIAN_POINT('Ctrl Pts',(58.0284498197529,249.697470551021,23.2830743911185)) ;
#115591=CARTESIAN_POINT('Ctrl Pts',(58.0254297310927,249.70737357761,23.2203767949559)) ;
#115592=CARTESIAN_POINT('Ctrl Pts',(58.0224096424324,249.713695185353,23.157232515933)) ;
#115593=CARTESIAN_POINT('Ctrl Pts',(58.0193895537721,249.716436503615,23.094083756793)) ;
#115594=CARTESIAN_POINT('Ctrl Pts',(58.0182449452072,249.717475458664,23.0701504824072)) ;
#115595=CARTESIAN_POINT('Ctrl Pts',(58.0171003366423,249.718001713324,23.0461979481158)) ;
#115596=CARTESIAN_POINT('Ctrl Pts',(58.0159557280774,249.718014855352,23.0222406924601)) ;
#115597=CARTESIAN_POINT('Origin',(67.8645744874958,248.040265107786,23.0213203435596)) ;
#115598=CARTESIAN_POINT('',(64.9402651077865,247.083045674831,21.643432097121)) ;
#115599=CARTESIAN_POINT('Ctrl Pts',(64.9402651077865,247.083045674831,21.643432097121)) ;
#115600=CARTESIAN_POINT('Ctrl Pts',(64.9429442584677,247.12507063848,21.6142373405957)) ;
#115601=CARTESIAN_POINT('Ctrl Pts',(64.9456568014745,247.168412522621,21.5869781986287)) ;
#115602=CARTESIAN_POINT('Ctrl Pts',(64.9534903335802,247.297537671544,21.5137865668355)) ;
#115603=CARTESIAN_POINT('Ctrl Pts',(64.9585541047601,247.386156155901,21.4732740839693)) ;
#115604=CARTESIAN_POINT('Ctrl Pts',(64.9651045226291,247.510493389731,21.4290290087006)) ;
#115605=CARTESIAN_POINT('Ctrl Pts',(64.9667974157123,247.54354804353,21.4184098240117)) ;
#115606=CARTESIAN_POINT('Ctrl Pts',(64.9698295496712,247.604424180614,21.4009169071032)) ;
#115607=CARTESIAN_POINT('Ctrl Pts',(64.9711783206033,247.632137220411,21.3937158607698)) ;
#115608=CARTESIAN_POINT('Ctrl Pts',(64.9741845354924,247.69525834054,21.3790279756566)) ;
#115609=CARTESIAN_POINT('Ctrl Pts',(64.9758286860229,247.730751853986,21.3719702773205)) ;
#115610=CARTESIAN_POINT('Ctrl Pts',(64.9814973341675,247.856004905134,21.3512504991235)) ;
#115611=CARTESIAN_POINT('Ctrl Pts',(64.9853512460892,247.946620612448,21.3437277039494)) ;
#115612=CARTESIAN_POINT('Ctrl Pts',(64.9919640501974,248.103010786515,21.3434608258745)) ;
#115613=CARTESIAN_POINT('Ctrl Pts',(64.9947278190027,248.168567408158,21.3471974311091)) ;
#115614=CARTESIAN_POINT('Ctrl Pts',(64.9988173788173,248.261737060338,21.3580134073213)) ;
#115615=CARTESIAN_POINT('Ctrl Pts',(65.0000640303766,248.289652569886,21.3619693947758)) ;
#115616=CARTESIAN_POINT('Ctrl Pts',(65.0023757763416,248.340108117153,21.3704215465206)) ;
#115617=CARTESIAN_POINT('Ctrl Pts',(65.0034315115626,248.362680892829,21.3746811471485)) ;
#115618=CARTESIAN_POINT('Ctrl Pts',(65.0052841444264,248.4012774587,21.3827885489868)) ;
#115619=CARTESIAN_POINT('Ctrl Pts',(65.0060701180475,248.417344242686,21.386411279269)) ;
#115620=CARTESIAN_POINT('Ctrl Pts',(65.0079962241007,248.455971264325,21.3957205707178)) ;
#115621=CARTESIAN_POINT('Ctrl Pts',(65.0091473486686,248.478469988853,21.4016405548478)) ;
#115622=CARTESIAN_POINT('Ctrl Pts',(65.0150051661908,248.590558436948,21.4336401892062)) ;
#115623=CARTESIAN_POINT('Ctrl Pts',(65.0199617587939,248.677982187339,21.4666929349023)) ;
#115624=CARTESIAN_POINT('Ctrl Pts',(65.0301831850078,248.852853334251,21.5500519205486)) ;
#115625=CARTESIAN_POINT('Ctrl Pts',(65.0354170419856,248.939451890663,21.6013212356338)) ;
#115626=CARTESIAN_POINT('Ctrl Pts',(65.0421053422461,249.048876189929,21.6801517141006)) ;
#115627=CARTESIAN_POINT('Ctrl Pts',(65.0437828749084,249.076176909543,21.7011246956489)) ;
#115628=CARTESIAN_POINT('Ctrl Pts',(65.0467952350284,249.124902498778,21.7409995180681)) ;
#115629=CARTESIAN_POINT('Ctrl Pts',(65.0481392160044,249.14652645241,21.7596366918629)) ;
#115630=CARTESIAN_POINT('Ctrl Pts',(65.051140548017,249.194471114417,21.8031398531834)) ;
#115631=CARTESIAN_POINT('Ctrl Pts',(65.0527843895861,249.220483820073,21.8283244466984)) ;
#115632=CARTESIAN_POINT('Ctrl Pts',(65.0589312649896,249.316325785309,21.927320851295)) ;
#115633=CARTESIAN_POINT('Ctrl Pts',(65.0632071273875,249.380216364349,22.00658009368)) ;
#115634=CARTESIAN_POINT('Ctrl Pts',(65.0711704638523,249.484919915245,22.1637478284439)) ;
#115635=CARTESIAN_POINT('Ctrl Pts',(65.0748495832706,249.527553272571,22.2400203241101)) ;
#115636=CARTESIAN_POINT('Ctrl Pts',(65.0798106033813,249.573462309034,22.3396632888364)) ;
#115637=CARTESIAN_POINT('Ctrl Pts',(65.0808441557246,249.58245401302,22.3602580953042)) ;
#115638=CARTESIAN_POINT('Ctrl Pts',(65.0826668577343,249.597254712333,22.3961047410567)) ;
#115639=CARTESIAN_POINT('Ctrl Pts',(65.0834457249163,249.603259483455,22.4112713940417)) ;
#115640=CARTESIAN_POINT('Ctrl Pts',(65.0853603700128,249.617255362344,22.4481855550469)) ;
#115641=CARTESIAN_POINT('Ctrl Pts',(65.0865072770545,249.62501846455,22.4700142096568)) ;
#115642=CARTESIAN_POINT('Ctrl Pts',(65.0923552155905,249.661714190565,22.5803847497001)) ;
#115643=CARTESIAN_POINT('Ctrl Pts',(65.0973069440346,249.683688334885,22.6710634921928)) ;
#115644=CARTESIAN_POINT('Ctrl Pts',(65.1074780770495,249.713338807993,22.8614116087466)) ;
#115645=CARTESIAN_POINT('Ctrl Pts',(65.1126679093436,249.719878348329,22.9609082642936)) ;
#115646=CARTESIAN_POINT('Ctrl Pts',(65.119323468634,249.716755152683,23.0949345744186)) ;
#115647=CARTESIAN_POINT('Ctrl Pts',(65.1210084104323,249.714884513712,23.129431290351)) ;
#115648=CARTESIAN_POINT('Ctrl Pts',(65.1240154692681,249.709548965202,23.192011448943)) ;
#115649=CARTESIAN_POINT('Ctrl Pts',(65.1253474629761,249.706436258269,23.2201113362441)) ;
#115650=CARTESIAN_POINT('Ctrl Pts',(65.1283238725396,249.697763541368,23.2836787901742)) ;
#115651=CARTESIAN_POINT('Ctrl Pts',(65.1299548226282,249.691772330958,23.3190737776624)) ;
#115652=CARTESIAN_POINT('Ctrl Pts',(65.1350504674581,249.669116953594,23.4309714885259)) ;
#115653=CARTESIAN_POINT('Ctrl Pts',(65.1383947776014,249.648232939902,23.5065140499877)) ;
#115654=CARTESIAN_POINT('Ctrl Pts',(65.1460082802719,249.588134284354,23.6765825893051)) ;
#115655=CARTESIAN_POINT('Ctrl Pts',(65.1502305999692,249.545406572774,23.7695274956142)) ;
#115656=CARTESIAN_POINT('Ctrl Pts',(65.1560023665131,249.480698169872,23.8819966810041)) ;
#115657=CARTESIAN_POINT('Ctrl Pts',(65.1572568431672,249.466304071478,23.9056414940144)) ;
#115658=CARTESIAN_POINT('Ctrl Pts',(65.1593194550077,249.442312338524,23.9429420954991)) ;
#115659=CARTESIAN_POINT('Ctrl Pts',(65.1601068460634,249.43308394525,23.9568302435055)) ;
#115660=CARTESIAN_POINT('Ctrl Pts',(65.1618486804703,249.412565424976,23.9867325407185)) ;
#115661=CARTESIAN_POINT('Ctrl Pts',(65.1628072591128,249.40119930379,24.0026902658671)) ;
#115662=CARTESIAN_POINT('Ctrl Pts',(65.1658433818841,249.364861971646,24.0518613283244)) ;
#115663=CARTESIAN_POINT('Ctrl Pts',(65.1679693571847,249.338935540798,24.0843472902241)) ;
#115664=CARTESIAN_POINT('Ctrl Pts',(65.1749563133598,249.251189000192,24.1862879323962)) ;
#115665=CARTESIAN_POINT('Ctrl Pts',(65.179925186363,249.184796137221,24.2515785716899)) ;
#115666=CARTESIAN_POINT('Ctrl Pts',(65.1874216699593,249.074449164494,24.3433897312442)) ;
#115667=CARTESIAN_POINT('Ctrl Pts',(65.1900282577352,249.034116798202,24.3739708699628)) ;
#115668=CARTESIAN_POINT('Ctrl Pts',(65.1946544678301,248.95853025337,24.4260739293042)) ;
#115669=CARTESIAN_POINT('Ctrl Pts',(65.1966919981801,248.923746636596,24.4482065491329)) ;
#115670=CARTESIAN_POINT('Ctrl Pts',(65.2000806067675,248.863298028551,24.4836108252965)) ;
#115671=CARTESIAN_POINT('Ctrl Pts',(65.2014536159437,248.838042315875,24.4975412914879)) ;
#115672=CARTESIAN_POINT('Ctrl Pts',(65.2042967037316,248.784180894151,24.5254637868292)) ;
#115673=CARTESIAN_POINT('Ctrl Pts',(65.2057614599285,248.755510610096,24.5393065804216)) ;
#115674=CARTESIAN_POINT('Ctrl Pts',(65.2101065780863,248.667896007713,24.578575499168)) ;
#115675=CARTESIAN_POINT('Ctrl Pts',(65.2129069953708,248.607868827205,24.6014440780068)) ;
#115676=CARTESIAN_POINT('Ctrl Pts',(65.2205135385875,248.438355378822,24.6551130669273)) ;
#115677=CARTESIAN_POINT('Ctrl Pts',(65.225169771777,248.326838347832,24.6783139549291)) ;
#115678=CARTESIAN_POINT('Ctrl Pts',(65.231290067591,248.187545396196,24.6928024449318)) ;
#115679=CARTESIAN_POINT('Ctrl Pts',(65.2324622510384,248.161191675343,24.6949154454761)) ;
#115680=CARTESIAN_POINT('Ctrl Pts',(65.2346518915165,248.11291675029,24.6976398848391)) ;
#115681=CARTESIAN_POINT('Ctrl Pts',(65.2356613661984,248.091012246291,24.6984458951228)) ;
#115682=CARTESIAN_POINT('Ctrl Pts',(65.2374610128899,248.052764168063,24.6991033291543)) ;
#115683=CARTESIAN_POINT('Ctrl Pts',(65.238241992344,248.036427754098,24.6991454827031)) ;
#115684=CARTESIAN_POINT('Ctrl Pts',(65.2401914157994,247.996274145899,24.6986626703289)) ;
#115685=CARTESIAN_POINT('Ctrl Pts',(65.2413722310537,247.972465038682,24.6978690413795)) ;
#115686=CARTESIAN_POINT('Ctrl Pts',(65.2458790470289,247.883083345827,24.6929826902272)) ;
#115687=CARTESIAN_POINT('Ctrl Pts',(65.2493207892809,247.817755356926,24.6855467624979)) ;
#115688=CARTESIAN_POINT('Ctrl Pts',(65.257209788155,247.670373880065,24.6599370900106)) ;
#115689=CARTESIAN_POINT('Ctrl Pts',(65.2616564299217,247.588901450293,24.6393921991111)) ;
#115690=CARTESIAN_POINT('Ctrl Pts',(65.2688086709557,247.456985146216,24.5953825016102)) ;
#115691=CARTESIAN_POINT('Ctrl Pts',(65.2715864294882,247.405554245718,24.5753570504909)) ;
#115692=CARTESIAN_POINT('Ctrl Pts',(65.275790800191,247.32716430926,24.5402922240756)) ;
#115693=CARTESIAN_POINT('Ctrl Pts',(65.2772701387459,247.299477434678,24.5269836826802)) ;
#115694=CARTESIAN_POINT('Ctrl Pts',(65.2787248749179,247.272170391302,24.5129220226314)) ;
#115695=CARTESIAN_POINT('',(64.9402651077866,249.014605129081,21.6554848536838)) ;
#115696=CARTESIAN_POINT('Origin',(64.9402651077866,248.040265107786,23.0213203435596)) ;
#115697=CARTESIAN_POINT('',(65.0159557280376,249.718014941427,23.0220674823532)) ;
#115698=CARTESIAN_POINT('Ctrl Pts',(65.0159557280376,249.718014941427,23.0220674823532)) ;
#115699=CARTESIAN_POINT('Ctrl Pts',(65.0129864470475,249.71804263635,22.9598766929778)) ;
#115700=CARTESIAN_POINT('Ctrl Pts',(65.0100171660575,249.714608129592,22.8975767959568)) ;
#115701=CARTESIAN_POINT('Ctrl Pts',(65.0070478850675,249.707701354092,22.8355747460244)) ;
#115702=CARTESIAN_POINT('Ctrl Pts',(65.0040845793459,249.700808477526,22.7736974666644)) ;
#115703=CARTESIAN_POINT('Ctrl Pts',(65.0011212736242,249.690457279382,22.7121173204969)) ;
#115704=CARTESIAN_POINT('Ctrl Pts',(64.9981579679026,249.676689646731,22.6512395539492)) ;
#115705=CARTESIAN_POINT('Ctrl Pts',(64.9951981429141,249.6629381857,22.5904332951301)) ;
#115706=CARTESIAN_POINT('Ctrl Pts',(64.9922383179257,249.645778363244,22.5303282478015)) ;
#115707=CARTESIAN_POINT('Ctrl Pts',(64.9892784929372,249.625303467312,22.4713217423501)) ;
#115708=CARTESIAN_POINT('Ctrl Pts',(64.9863212174516,249.604846207829,22.4123660633003)) ;
#115709=CARTESIAN_POINT('Ctrl Pts',(64.983363941966,249.581079704203,22.3545075029837)) ;
#115710=CARTESIAN_POINT('Ctrl Pts',(64.9804066664804,249.554147202028,22.2981287595155)) ;
#115711=CARTESIAN_POINT('Ctrl Pts',(64.9774510127355,249.527229469373,22.2417809335958)) ;
#115712=CARTESIAN_POINT('Ctrl Pts',(64.9744953589907,249.497149396823,22.1869117481951)) ;
#115713=CARTESIAN_POINT('Ctrl Pts',(64.9715397052459,249.464097851673,22.1338828077664)) ;
#115714=CARTESIAN_POINT('Ctrl Pts',(64.9685837648145,249.431043100656,22.0808487237425)) ;
#115715=CARTESIAN_POINT('Ctrl Pts',(64.965627824383,249.395016548061,22.0296556582547)) ;
#115716=CARTESIAN_POINT('Ctrl Pts',(64.9626718839516,249.356253739544,21.9806383635174)) ;
#115717=CARTESIAN_POINT('Ctrl Pts',(64.9597158841829,249.317490152905,21.9316200848114)) ;
#115718=CARTESIAN_POINT('Ctrl Pts',(64.9567598844142,249.275990508209,21.8847780386099)) ;
#115719=CARTESIAN_POINT('Ctrl Pts',(64.9538038846455,249.232030816093,21.8404140987611)) ;
#115720=CARTESIAN_POINT('Ctrl Pts',(64.950845407407,249.18803428067,21.7960129767989)) ;
#115721=CARTESIAN_POINT('Ctrl Pts',(64.9478869301686,249.141573928527,21.7540944464987)) ;
#115722=CARTESIAN_POINT('Ctrl Pts',(64.9449284529302,249.09296200236,21.7149228884741)) ;
#115723=CARTESIAN_POINT('Ctrl Pts',(64.943374004549,249.067420237511,21.6943412986722)) ;
#115724=CARTESIAN_POINT('Ctrl Pts',(64.9418195561678,249.041285051488,21.6745173919063)) ;
#115725=CARTESIAN_POINT('Ctrl Pts',(64.9402651077866,249.014605129081,21.6554848536842)) ;
#115726=CARTESIAN_POINT('Ctrl Pts',(65.1788202510297,247.272170391302,24.5129220226314)) ;
#115727=CARTESIAN_POINT('Ctrl Pts',(65.1766225070709,247.313246345993,24.5340739321629)) ;
#115728=CARTESIAN_POINT('Ctrl Pts',(65.174424763112,247.355149468955,24.5535035893657)) ;
#115729=CARTESIAN_POINT('Ctrl Pts',(65.1722270191532,247.397721280128,24.5711533965168)) ;
#115730=CARTESIAN_POINT('Ctrl Pts',(65.1693116248914,247.454194470969,24.594566563589)) ;
#115731=CARTESIAN_POINT('Ctrl Pts',(65.1663962306296,247.512055207638,24.6149330907892)) ;
#115732=CARTESIAN_POINT('Ctrl Pts',(65.1634808363678,247.570943480191,24.6320910511313)) ;
#115733=CARTESIAN_POINT('Ctrl Pts',(65.1605701441249,247.629736776302,24.6492213386967)) ;
#115734=CARTESIAN_POINT('Ctrl Pts',(65.1576594518821,247.689553833606,24.6631531944018)) ;
#115735=CARTESIAN_POINT('Ctrl Pts',(65.1547487596392,247.750015894706,24.6737732042507)) ;
#115736=CARTESIAN_POINT('Ctrl Pts',(65.1518406833758,247.810423615637,24.684383669385)) ;
#115737=CARTESIAN_POINT('Ctrl Pts',(65.1489326071123,247.871474693329,24.6916881022789)) ;
#115738=CARTESIAN_POINT('Ctrl Pts',(65.1460245308489,247.932778055922,24.6956236602205)) ;
#115739=CARTESIAN_POINT('Ctrl Pts',(65.1431180102194,247.994048625153,24.6995571128913)) ;
#115740=CARTESIAN_POINT('Ctrl Pts',(65.14021148959,248.055570705937,24.7001252327289)) ;
#115741=CARTESIAN_POINT('Ctrl Pts',(65.1373049689605,248.11694797027,24.697317002596)) ;
#115742=CARTESIAN_POINT('Ctrl Pts',(65.13439894578,248.178314729927,24.6945092530898)) ;
#115743=CARTESIAN_POINT('Ctrl Pts',(65.1314929225996,248.239536215573,24.6883263250917)) ;
#115744=CARTESIAN_POINT('Ctrl Pts',(65.1285868994191,248.30021800925,24.6788092730914)) ;
#115745=CARTESIAN_POINT('Ctrl Pts',(65.1256782756473,248.36095410688,24.6692837043102)) ;
#115746=CARTESIAN_POINT('Ctrl Pts',(65.1227696518755,248.421149044928,24.6564181282543)) ;
#115747=CARTESIAN_POINT('Ctrl Pts',(65.1198610281037,248.48041663666,24.6403051162274)) ;
#115748=CARTESIAN_POINT('Ctrl Pts',(65.1169511589534,248.539709604855,24.6241852051305)) ;
#115749=CARTESIAN_POINT('Ctrl Pts',(65.1140412898031,248.598073952237,24.6048152453039)) ;
#115750=CARTESIAN_POINT('Ctrl Pts',(65.1111314206528,248.655139668826,24.5823374276062)) ;
#115751=CARTESIAN_POINT('Ctrl Pts',(65.1082162276858,248.712309791282,24.5598184851111)) ;
#115752=CARTESIAN_POINT('Ctrl Pts',(65.1053010347189,248.768176072337,24.5341805344946)) ;
#115753=CARTESIAN_POINT('Ctrl Pts',(65.102385841752,248.822390237397,24.5056132203633)) ;
#115754=CARTESIAN_POINT('Ctrl Pts',(65.0998926885117,248.868755683124,24.4811816672545)) ;
#115755=CARTESIAN_POINT('Ctrl Pts',(65.0973995352714,248.913913001855,24.4546084166935)) ;
#115756=CARTESIAN_POINT('Ctrl Pts',(65.094906382031,248.957661698003,24.4260368839186)) ;
#115757=CARTESIAN_POINT('Ctrl Pts',(65.0920042795803,249.008586445128,24.3927787937431)) ;
#115758=CARTESIAN_POINT('Ctrl Pts',(65.0891021771295,249.057803619847,24.3566803705642)) ;
#115759=CARTESIAN_POINT('Ctrl Pts',(65.0862000746787,249.104977954238,24.3179435028086)) ;
#115760=CARTESIAN_POINT('Ctrl Pts',(65.0833028142183,249.152073580976,24.2792712652799)) ;
#115761=CARTESIAN_POINT('Ctrl Pts',(65.0804055537579,249.197132739833,24.2379696450035)) ;
#115762=CARTESIAN_POINT('Ctrl Pts',(65.0775082932975,249.239849324372,24.194283586725)) ;
#115763=CARTESIAN_POINT('Ctrl Pts',(65.0746137241619,249.282526228598,24.1506381093242)) ;
#115764=CARTESIAN_POINT('Ctrl Pts',(65.0717191550263,249.322864513685,24.1046129485847)) ;
#115765=CARTESIAN_POINT('Ctrl Pts',(65.0688245858907,249.360592641566,24.0564919554392)) ;
#115766=CARTESIAN_POINT('Ctrl Pts',(65.0659316230768,249.398299832476,24.0083976667157)) ;
#115767=CARTESIAN_POINT('Ctrl Pts',(65.0630386602628,249.43339942201,23.9582102548082)) ;
#115768=CARTESIAN_POINT('Ctrl Pts',(65.0601456974489,249.465659540964,23.906247330584)) ;
#115769=CARTESIAN_POINT('Ctrl Pts',(65.0572532582051,249.497913821463,23.8542938106398)) ;
#115770=CARTESIAN_POINT('Ctrl Pts',(65.0543608189613,249.52732938148,23.8005658525202)) ;
#115771=CARTESIAN_POINT('Ctrl Pts',(65.0514683797175,249.553718335989,23.7454090042501)) ;
#115772=CARTESIAN_POINT('Ctrl Pts',(65.0485732702767,249.580131651843,23.6902012371412)) ;
#115773=CARTESIAN_POINT('Ctrl Pts',(65.045678160836,249.603512557016,23.6335624081256)) ;
#115774=CARTESIAN_POINT('Ctrl Pts',(65.0427830513952,249.623720301239,23.5758604348308)) ;
#115775=CARTESIAN_POINT('Ctrl Pts',(65.0398866790995,249.643936860137,23.5181332917711)) ;
#115776=CARTESIAN_POINT('Ctrl Pts',(65.0369903068037,249.660977356128,23.4593425740367)) ;
#115777=CARTESIAN_POINT('Ctrl Pts',(65.034093934508,249.674751137605,23.3998708432641)) ;
#115778=CARTESIAN_POINT('Ctrl Pts',(65.0311920366838,249.688551195891,23.3402856558261)) ;
#115779=CARTESIAN_POINT('Ctrl Pts',(65.0282901388595,249.699071998874,23.2800173665856)) ;
#115780=CARTESIAN_POINT('Ctrl Pts',(65.0253882410353,249.706274347918,23.2194573524548)) ;
#115781=CARTESIAN_POINT('Ctrl Pts',(65.0227874089931,249.712729468432,23.1651803121289)) ;
#115782=CARTESIAN_POINT('Ctrl Pts',(65.0201865769509,249.716519689942,23.1106692791193)) ;
#115783=CARTESIAN_POINT('Ctrl Pts',(65.0175857449087,249.717652389637,23.0562054289579)) ;
#115784=CARTESIAN_POINT('Ctrl Pts',(65.0170424059649,249.717889021548,23.0448274044094)) ;
#115785=CARTESIAN_POINT('Ctrl Pts',(65.0164990670211,249.718009873619,23.0334475707981)) ;
#115786=CARTESIAN_POINT('Ctrl Pts',(65.0159557280773,249.718014941427,23.0220674831853)) ;
#115787=CARTESIAN_POINT('Origin',(64.9402651077866,248.040265107786,23.0213203435596)) ;
#115788=CARTESIAN_POINT('Ctrl Pts',(64.9402651077867,248.926035539849,24.7736739014023)) ;
#115789=CARTESIAN_POINT('Ctrl Pts',(64.9402651077866,248.976878141234,24.7437902125892)) ;
#115790=CARTESIAN_POINT('Ctrl Pts',(64.9402651077866,249.026203795482,24.711570348078)) ;
#115791=CARTESIAN_POINT('Ctrl Pts',(64.9402651077867,249.073820527419,24.6770177952892)) ;
#115792=CARTESIAN_POINT('Ctrl Pts',(64.9402651077868,249.08462711755,24.6691761131584)) ;
#115793=CARTESIAN_POINT('Ctrl Pts',(64.9402651077867,249.09534559418,24.6612141692458)) ;
#115794=CARTESIAN_POINT('Ctrl Pts',(64.9402651077867,249.10597357269,24.6531318456028)) ;
#115795=CARTESIAN_POINT('Ctrl Pts',(64.9402651077866,249.166471971025,24.6071242596107)) ;
#115796=CARTESIAN_POINT('Ctrl Pts',(64.9402651077868,249.224042137625,24.5572188157012)) ;
#115797=CARTESIAN_POINT('Ctrl Pts',(64.9402651077867,249.278496460635,24.5038024082393)) ;
#115798=CARTESIAN_POINT('Ctrl Pts',(64.9402651077867,249.292324750794,24.4902376893917)) ;
#115799=CARTESIAN_POINT('Ctrl Pts',(64.9402651077866,249.305954881182,24.4764429964786)) ;
#115800=CARTESIAN_POINT('Ctrl Pts',(64.9402651077866,249.319363494654,24.4624456517121)) ;
#115801=CARTESIAN_POINT('Ctrl Pts',(64.9402651077865,249.369335690605,24.410279329152)) ;
#115802=CARTESIAN_POINT('Ctrl Pts',(64.9402651077867,249.416286779042,24.3552521689592)) ;
#115803=CARTESIAN_POINT('Ctrl Pts',(64.9402651077868,249.460076530841,24.2977130577074)) ;
#115804=CARTESIAN_POINT('Ctrl Pts',(64.9402651077868,249.493619627768,24.2536379052686)) ;
#115805=CARTESIAN_POINT('Ctrl Pts',(64.9402651077866,249.525306996186,24.2080879408986)) ;
#115806=CARTESIAN_POINT('Ctrl Pts',(64.9402651077865,249.555057167624,24.1612106694906)) ;
#115807=CARTESIAN_POINT('Ctrl Pts',(64.9402651077865,249.566305768275,24.1434862773203)) ;
#115808=CARTESIAN_POINT('Ctrl Pts',(64.9402651077866,249.577277252061,24.1255720746347)) ;
#115809=CARTESIAN_POINT('Ctrl Pts',(64.9402651077866,249.587966566315,24.1074758724398)) ;
#115810=CARTESIAN_POINT('Ctrl Pts',(64.9402651077865,249.597031260778,24.0921300289246)) ;
#115811=CARTESIAN_POINT('Ctrl Pts',(64.9402651077867,249.605895515243,24.0766485406753)) ;
#115812=CARTESIAN_POINT('Ctrl Pts',(64.9402651077867,249.61454108935,24.0610639553866)) ;
#115813=CARTESIAN_POINT('Ctrl Pts',(64.9402651077866,249.649154760442,23.9986690579923)) ;
#115814=CARTESIAN_POINT('Ctrl Pts',(64.9402651077868,249.680311264252,23.9345528731401)) ;
#115815=CARTESIAN_POINT('Ctrl Pts',(64.9402651077867,249.707874303453,23.8690437513651)) ;
#115816=CARTESIAN_POINT('Ctrl Pts',(64.9402651077867,249.734984622184,23.8046106110963)) ;
#115817=CARTESIAN_POINT('Ctrl Pts',(64.9402651077868,249.758618760034,23.7388289129817)) ;
#115818=CARTESIAN_POINT('Ctrl Pts',(64.9402651077867,249.778599553308,23.6719980103639)) ;
#115819=CARTESIAN_POINT('Ctrl Pts',(64.9402651077866,249.793454839143,23.6223106857726)) ;
#115820=CARTESIAN_POINT('Ctrl Pts',(64.9402651077868,249.806289760678,23.5720430656005)) ;
#115821=CARTESIAN_POINT('Ctrl Pts',(64.9402651077867,249.817012969291,23.52131816757)) ;
#115822=CARTESIAN_POINT('Ctrl Pts',(64.9402651077867,249.823067203089,23.492679314856)) ;
#115823=CARTESIAN_POINT('Ctrl Pts',(64.9402651077865,249.828448004765,23.4638947217814)) ;
#115824=CARTESIAN_POINT('Ctrl Pts',(64.9402651077865,249.833136547529,23.4349869551096)) ;
#115825=CARTESIAN_POINT('Ctrl Pts',(64.9402651077865,249.83508243226,23.4229893719325)) ;
#115826=CARTESIAN_POINT('Ctrl Pts',(64.9402651077869,249.836909364897,23.4109683655323)) ;
#115827=CARTESIAN_POINT('Ctrl Pts',(64.9402651077869,249.838614913707,23.3989326615467)) ;
#115828=CARTESIAN_POINT('Ctrl Pts',(64.9402651077868,249.848169345995,23.3315090158141)) ;
#115829=CARTESIAN_POINT('Ctrl Pts',(64.9402651077869,249.853889383611,23.2638409901629)) ;
#115830=CARTESIAN_POINT('Ctrl Pts',(64.9402651077868,249.855620926811,23.1962106757776)) ;
#115831=CARTESIAN_POINT('Ctrl Pts',(64.9402651077867,249.856792844341,23.1504381238818)) ;
#115832=CARTESIAN_POINT('Ctrl Pts',(64.9402651077866,249.856136765347,23.1046826723625)) ;
#115833=CARTESIAN_POINT('Ctrl Pts',(64.9402651077866,249.853591307226,23.0590325880763)) ;
#115834=CARTESIAN_POINT('Ctrl Pts',(64.9402651077865,249.849670880286,22.9887239003222)) ;
#115835=CARTESIAN_POINT('Ctrl Pts',(64.9402651077867,249.841270878845,22.9186637285971)) ;
#115836=CARTESIAN_POINT('Ctrl Pts',(64.9402651077868,249.82857851078,22.8491862645525)) ;
#115837=CARTESIAN_POINT('Ctrl Pts',(64.9402651077869,249.823025599751,22.818789874033)) ;
#115838=CARTESIAN_POINT('Ctrl Pts',(64.9402651077869,249.816650415106,22.7885053138842)) ;
#115839=CARTESIAN_POINT('Ctrl Pts',(64.9402651077867,249.809465657346,22.7583623017282)) ;
#115840=CARTESIAN_POINT('Ctrl Pts',(64.9402651077866,249.806390130223,22.7454592012243)) ;
#115841=CARTESIAN_POINT('Ctrl Pts',(64.9402651077867,249.803166237982,22.7325820535054)) ;
#115842=CARTESIAN_POINT('Ctrl Pts',(64.9402651077868,249.799794886782,22.7197332657928)) ;
#115843=CARTESIAN_POINT('Ctrl Pts',(64.9402651077868,249.796887514073,22.7086527783227)) ;
#115844=CARTESIAN_POINT('Ctrl Pts',(64.9402651077868,249.793870437363,22.6975935970397)) ;
#115845=CARTESIAN_POINT('Ctrl Pts',(64.9402651077868,249.790748373431,22.6865709478748)) ;
#115846=CARTESIAN_POINT('Ctrl Pts',(64.9402651077867,249.772317375906,22.6214991159499)) ;
#115847=CARTESIAN_POINT('Ctrl Pts',(64.9402651077867,249.750200212747,22.5575763668043)) ;
#115848=CARTESIAN_POINT('Ctrl Pts',(64.9402651077867,249.724600278997,22.4950834172018)) ;
#115849=CARTESIAN_POINT('Ctrl Pts',(64.9402651077867,249.698928372785,22.4324147729458)) ;
#115850=CARTESIAN_POINT('Ctrl Pts',(64.9402651077868,249.66975345666,22.3711830743851)) ;
#115851=CARTESIAN_POINT('Ctrl Pts',(64.9402651077868,249.637235007895,22.3116966832185)) ;
#115852=CARTESIAN_POINT('Ctrl Pts',(64.9402651077868,249.605225152613,22.2531406682546)) ;
#115853=CARTESIAN_POINT('Ctrl Pts',(64.9402651077865,249.569974852449,22.1962750527875)) ;
#115854=CARTESIAN_POINT('Ctrl Pts',(64.9402651077866,249.531601964295,22.1414304652508)) ;
#115855=CARTESIAN_POINT('Ctrl Pts',(64.9402651077866,249.523894275526,22.1304142235314)) ;
#115856=CARTESIAN_POINT('Ctrl Pts',(64.9402651077868,249.516060509705,22.1194796620047)) ;
#115857=CARTESIAN_POINT('Ctrl Pts',(64.9402651077867,249.508101488473,22.1086296820219)) ;
#115858=CARTESIAN_POINT('Ctrl Pts',(64.9402651077866,249.501173892893,22.0991857728804)) ;
#115859=CARTESIAN_POINT('Ctrl Pts',(64.9402651077867,249.49415087098,22.0898054003738)) ;
#115860=CARTESIAN_POINT('Ctrl Pts',(64.9402651077867,249.487043011387,22.0805032570583)) ;
#115861=CARTESIAN_POINT('Ctrl Pts',(64.9402651077868,249.446920840516,22.0279948783107)) ;
#115862=CARTESIAN_POINT('Ctrl Pts',(64.9402651077866,249.404026484517,21.9778764926067)) ;
#115863=CARTESIAN_POINT('Ctrl Pts',(64.9402651077866,249.358515301884,21.9304287169379)) ;
#115864=CARTESIAN_POINT('Ctrl Pts',(64.9402651077866,249.313732515653,21.8837403324135)) ;
#115865=CARTESIAN_POINT('Ctrl Pts',(64.9402651077866,249.26641533439,21.8396371047943)) ;
#115866=CARTESIAN_POINT('Ctrl Pts',(64.9402651077867,249.216681222564,21.7984258204361)) ;
#115867=CARTESIAN_POINT('Ctrl Pts',(64.9402651077868,249.168600536501,21.758584617834)) ;
#115868=CARTESIAN_POINT('Ctrl Pts',(64.9402651077867,249.118260356068,21.7214458696138)) ;
#115869=CARTESIAN_POINT('Ctrl Pts',(64.9402651077866,249.065747227906,21.6873312956639)) ;
#115870=CARTESIAN_POINT('Ctrl Pts',(64.9402651077866,249.048922193034,21.6764010975127)) ;
#115871=CARTESIAN_POINT('Ctrl Pts',(64.9402651077868,249.03187397738,21.6657817184762)) ;
#115872=CARTESIAN_POINT('Ctrl Pts',(64.9402651077866,249.014605129081,21.6554848536838)) ;
#115873=CARTESIAN_POINT('',(64.9396944788746,247.064665290212,21.6551748675434)) ;
#115874=CARTESIAN_POINT('Ctrl Pts',(64.9402651077865,247.083045674831,21.643432097121)) ;
#115875=CARTESIAN_POINT('Ctrl Pts',(64.9400748981492,247.077082473966,21.6475747347883)) ;
#115876=CARTESIAN_POINT('Ctrl Pts',(64.9398846885119,247.071146166134,21.6517560841535)) ;
#115877=CARTESIAN_POINT('Ctrl Pts',(64.9396944788746,247.065237251657,21.655975792806)) ;
#115878=CARTESIAN_POINT('Ctrl Pts',(64.9402651077866,247.06404364217,21.6543968943227)) ;
#115879=CARTESIAN_POINT('Ctrl Pts',(64.9402651077866,247.007203713347,21.6877084303973)) ;
#115880=CARTESIAN_POINT('Ctrl Pts',(64.9402651077865,246.952576865232,21.724365095361)) ;
#115881=CARTESIAN_POINT('Ctrl Pts',(64.9402651077866,246.900517061953,21.7642811845472)) ;
#115882=CARTESIAN_POINT('Ctrl Pts',(64.9402651077866,246.894704358926,21.7687379891796)) ;
#115883=CARTESIAN_POINT('Ctrl Pts',(64.9402651077864,246.888923672635,21.7732354797134)) ;
#115884=CARTESIAN_POINT('Ctrl Pts',(64.9402651077864,246.883175508364,21.7777735755836)) ;
#115885=CARTESIAN_POINT('Ctrl Pts',(64.9402651077864,246.848492482056,21.8051553432266)) ;
#115886=CARTESIAN_POINT('Ctrl Pts',(64.9402651077864,246.814992948051,21.8340145353038)) ;
#115887=CARTESIAN_POINT('Ctrl Pts',(64.9402651077864,246.782700575228,21.8642422611924)) ;
#115888=CARTESIAN_POINT('Ctrl Pts',(64.9402651077864,246.76387471842,21.8818644669791)) ;
#115889=CARTESIAN_POINT('Ctrl Pts',(64.9402651077867,246.745459251001,21.8999519959579)) ;
#115890=CARTESIAN_POINT('Ctrl Pts',(64.9402651077865,246.727459923415,21.9184848035206)) ;
#115891=CARTESIAN_POINT('Ctrl Pts',(64.9402651077864,246.717725176082,21.9285080778969)) ;
#115892=CARTESIAN_POINT('Ctrl Pts',(64.9402651077866,246.708111935049,21.9386620458343)) ;
#115893=CARTESIAN_POINT('Ctrl Pts',(64.9402651077866,246.698631593824,21.9489318831291)) ;
#115894=CARTESIAN_POINT('Ctrl Pts',(64.9402651077866,246.654113902873,21.9971568817832)) ;
#115895=CARTESIAN_POINT('Ctrl Pts',(64.9402651077864,246.612466101452,22.0479919890593)) ;
#115896=CARTESIAN_POINT('Ctrl Pts',(64.9402651077865,246.573755852033,22.1010784736613)) ;
#115897=CARTESIAN_POINT('Ctrl Pts',(64.9402651077866,246.542635674679,22.1437560807737)) ;
#115898=CARTESIAN_POINT('Ctrl Pts',(64.9402651077864,246.513414425502,22.1878899252643)) ;
#115899=CARTESIAN_POINT('Ctrl Pts',(64.9402651077866,246.486142358642,22.2333127807452)) ;
#115900=CARTESIAN_POINT('Ctrl Pts',(64.9402651077866,246.476976048295,22.2485796834088)) ;
#115901=CARTESIAN_POINT('Ctrl Pts',(64.9402651077866,246.468030056022,22.26399232338)) ;
#115902=CARTESIAN_POINT('Ctrl Pts',(64.9402651077866,246.45930668306,22.2795446899308)) ;
#115903=CARTESIAN_POINT('Ctrl Pts',(64.9402651077867,246.451879243981,22.2927866154568)) ;
#115904=CARTESIAN_POINT('Ctrl Pts',(64.9402651077865,246.444612289006,22.3061318511815)) ;
#115905=CARTESIAN_POINT('Ctrl Pts',(64.9402651077866,246.437517831176,22.3195560702723)) ;
#115906=CARTESIAN_POINT('Ctrl Pts',(64.9402651077867,246.405909948836,22.3793648883246)) ;
#115907=CARTESIAN_POINT('Ctrl Pts',(64.9402651077867,246.377673843717,22.4408238708802)) ;
#115908=CARTESIAN_POINT('Ctrl Pts',(64.9402651077867,246.352882265298,22.5035718480605)) ;
#115909=CARTESIAN_POINT('Ctrl Pts',(64.9402651077867,246.327697168515,22.5673158280324)) ;
#115910=CARTESIAN_POINT('Ctrl Pts',(64.9402651077866,246.30606621932,22.6323909223172)) ;
#115911=CARTESIAN_POINT('Ctrl Pts',(64.9402651077865,246.288105482506,22.6984537994672)) ;
#115912=CARTESIAN_POINT('Ctrl Pts',(64.9402651077864,246.274905996492,22.7470039247776)) ;
#115913=CARTESIAN_POINT('Ctrl Pts',(64.9402651077866,246.26368954438,22.7960883480033)) ;
#115914=CARTESIAN_POINT('Ctrl Pts',(64.9402651077865,246.25451844377,22.8455783499823)) ;
#115915=CARTESIAN_POINT('Ctrl Pts',(64.9402651077865,246.249295136931,22.8737648759862)) ;
#115916=CARTESIAN_POINT('Ctrl Pts',(64.9402651077866,246.244735556015,22.9020830550201)) ;
#115917=CARTESIAN_POINT('Ctrl Pts',(64.9402651077864,246.240853456109,22.9305095743852)) ;
#115918=CARTESIAN_POINT('Ctrl Pts',(64.9402651077864,246.238895922423,22.9448435355323)) ;
#115919=CARTESIAN_POINT('Ctrl Pts',(64.9402651077865,246.23711043215,22.9592083501525)) ;
#115920=CARTESIAN_POINT('Ctrl Pts',(64.9402651077865,246.23550138577,22.9735755832766)) ;
#115921=CARTESIAN_POINT('Ctrl Pts',(64.9402651077866,246.227718516974,23.0430690992986)) ;
#115922=CARTESIAN_POINT('Ctrl Pts',(64.9402651077865,246.224042287029,23.1127331202832)) ;
#115923=CARTESIAN_POINT('Ctrl Pts',(64.9402651077865,246.224580256665,23.1822119780025)) ;
#115924=CARTESIAN_POINT('Ctrl Pts',(64.9402651077864,246.224872323712,23.2199324800773)) ;
#115925=CARTESIAN_POINT('Ctrl Pts',(64.9402651077866,246.226407295656,23.2575988579456)) ;
#115926=CARTESIAN_POINT('Ctrl Pts',(64.9402651077866,246.229208441131,23.2951564187047)) ;
#115927=CARTESIAN_POINT('Ctrl Pts',(64.9402651077865,246.234233948422,23.3625380656402)) ;
#115928=CARTESIAN_POINT('Ctrl Pts',(64.9402651077864,246.24333176806,23.4295696364802)) ;
#115929=CARTESIAN_POINT('Ctrl Pts',(64.9402651077864,246.256283967996,23.4960087497214)) ;
#115930=CARTESIAN_POINT('Ctrl Pts',(64.9402651077863,246.262795924935,23.5294122369009)) ;
#115931=CARTESIAN_POINT('Ctrl Pts',(64.9402651077864,246.270283012217,23.5626659794887)) ;
#115932=CARTESIAN_POINT('Ctrl Pts',(64.9402651077865,246.27872235646,23.5957387507467)) ;
#115933=CARTESIAN_POINT('Ctrl Pts',(64.9402651077865,246.282866147924,23.611977769237)) ;
#115934=CARTESIAN_POINT('Ctrl Pts',(64.9402651077863,246.287239565845,23.6281731490293)) ;
#115935=CARTESIAN_POINT('Ctrl Pts',(64.9402651077864,246.291840169129,23.6443211300255)) ;
#115936=CARTESIAN_POINT('Ctrl Pts',(64.9402651077864,246.29470680334,23.6543829310353)) ;
#115937=CARTESIAN_POINT('Ctrl Pts',(64.9402651077863,246.297660952432,23.6644237151454)) ;
#115938=CARTESIAN_POINT('Ctrl Pts',(64.9402651077864,246.300699298176,23.6744344455488)) ;
#115939=CARTESIAN_POINT('Ctrl Pts',(64.9402651077866,246.320915032361,23.7410411723224)) ;
#115940=CARTESIAN_POINT('Ctrl Pts',(64.9402651077867,246.344883302498,23.8064223337815)) ;
#115941=CARTESIAN_POINT('Ctrl Pts',(64.9402651077867,246.372338922461,23.8703257415957)) ;
#115942=CARTESIAN_POINT('Ctrl Pts',(64.9402651077867,246.400335511009,23.9354882627066)) ;
#115943=CARTESIAN_POINT('Ctrl Pts',(64.9402651077864,246.43195851161,23.9991150988841)) ;
#115944=CARTESIAN_POINT('Ctrl Pts',(64.9402651077865,246.466981592319,24.0609347791762)) ;
#115945=CARTESIAN_POINT('Ctrl Pts',(64.9402651077866,246.502167767235,24.1230423391028)) ;
#115946=CARTESIAN_POINT('Ctrl Pts',(64.9402651077864,246.540786197948,24.1833268110854)) ;
#115947=CARTESIAN_POINT('Ctrl Pts',(64.9402651077867,246.582656540073,24.2414951008919)) ;
#115948=CARTESIAN_POINT('Ctrl Pts',(64.9402651077868,246.592936185813,24.2557760783621)) ;
#115949=CARTESIAN_POINT('Ctrl Pts',(64.9402651077867,246.603412056763,24.2699293792961)) ;
#115950=CARTESIAN_POINT('Ctrl Pts',(64.9402651077867,246.614081887465,24.2839504011325)) ;
#115951=CARTESIAN_POINT('Ctrl Pts',(64.9402651077867,246.622719436239,24.2953008398928)) ;
#115952=CARTESIAN_POINT('Ctrl Pts',(64.9402651077867,246.631485589334,24.3065662771629)) ;
#115953=CARTESIAN_POINT('Ctrl Pts',(64.9402651077867,246.640364653424,24.3177264676288)) ;
#115954=CARTESIAN_POINT('Ctrl Pts',(64.9402651077865,246.685954500382,24.3750288330827)) ;
#115955=CARTESIAN_POINT('Ctrl Pts',(64.9402651077868,246.734594144709,24.4296616563077)) ;
#115956=CARTESIAN_POINT('Ctrl Pts',(64.9402651077866,246.786040477115,24.4813467612197)) ;
#115957=CARTESIAN_POINT('Ctrl Pts',(64.9402651077865,246.837430222288,24.5329750162671)) ;
#115958=CARTESIAN_POINT('Ctrl Pts',(64.9402651077866,246.891621013889,24.5816629683342)) ;
#115959=CARTESIAN_POINT('Ctrl Pts',(64.9402651077867,246.948416932819,24.6271104818581)) ;
#115960=CARTESIAN_POINT('Ctrl Pts',(64.9402651077868,247.003811560799,24.6714366966933)) ;
#115961=CARTESIAN_POINT('Ctrl Pts',(64.9402651077867,247.061684973714,24.7126811411786)) ;
#115962=CARTESIAN_POINT('Ctrl Pts',(64.9402651077867,247.121890830459,24.7505314348811)) ;
#115963=CARTESIAN_POINT('Ctrl Pts',(64.9402651077867,247.143744240579,24.7642702642267)) ;
#115964=CARTESIAN_POINT('Ctrl Pts',(64.9402651077866,247.165905256939,24.777561520028)) ;
#115965=CARTESIAN_POINT('Ctrl Pts',(64.9402651077866,247.188367839728,24.7903888257487)) ;
#115966=CARTESIAN_POINT('Ctrl Pts',(67.1068977162686,248.766941441459,24.5303522971223)) ;
#115967=CARTESIAN_POINT('Ctrl Pts',(67.0811241705612,249.255686601031,24.2949964189254)) ;
#115968=CARTESIAN_POINT('Ctrl Pts',(67.0295770791465,249.979311447899,23.3159220295678)) ;
#115969=CARTESIAN_POINT('Ctrl Pts',(66.9522564420243,249.378048699798,21.5837974034299)) ;
#115970=CARTESIAN_POINT('Ctrl Pts',(66.8749358049021,247.607584691196,21.1069207281648)) ;
#115971=CARTESIAN_POINT('Ctrl Pts',(66.7976151677799,246.21545175278,22.298523800085)) ;
#115972=CARTESIAN_POINT('Ctrl Pts',(66.7202945306578,246.414252996263,24.1208760392277)) ;
#115973=CARTESIAN_POINT('Ctrl Pts',(66.6429738935356,248.031328286107,24.9840872012945)) ;
#115974=CARTESIAN_POINT('Ctrl Pts',(66.5656532564134,249.656094335495,24.1356422797888)) ;
#115975=CARTESIAN_POINT('Ctrl Pts',(66.4883326192912,249.871729536703,22.315345749206)) ;
#115976=CARTESIAN_POINT('Ctrl Pts',(66.4110119821691,248.490108895369,21.1107541100679)) ;
#115977=CARTESIAN_POINT('Ctrl Pts',(66.3336913450469,246.71618583806,21.5723731211514)) ;
#115978=CARTESIAN_POINT('Ctrl Pts',(66.2563707079247,246.096997993504,23.2976342270491)) ;
#115979=CARTESIAN_POINT('Ctrl Pts',(66.1790500708025,247.172550498697,24.7819180094862)) ;
#115980=CARTESIAN_POINT('Ctrl Pts',(66.1017294336803,249.004842624028,24.7307717823553)) ;
#115981=CARTESIAN_POINT('Ctrl Pts',(66.0244087965582,249.995919764197,23.1887994578465)) ;
#115982=CARTESIAN_POINT('Ctrl Pts',(65.947088159436,249.281455006808,21.5007672727967)) ;
#115983=CARTESIAN_POINT('Ctrl Pts',(65.8697675223138,247.484539411195,21.1388215429649)) ;
#115984=CARTESIAN_POINT('Ctrl Pts',(65.7924468851916,246.172275648143,22.4186165868738)) ;
#115985=CARTESIAN_POINT('Ctrl Pts',(65.7151262480695,246.489101665562,24.2240364120271)) ;
#115986=CARTESIAN_POINT('Ctrl Pts',(65.6378056109473,248.158705508057,24.9805535194141)) ;
#115987=CARTESIAN_POINT('Ctrl Pts',(65.5604849738251,249.725024728806,24.0284187010416)) ;
#115988=CARTESIAN_POINT('Ctrl Pts',(65.483164336703,249.822034046853,22.1979632409268)) ;
#115989=CARTESIAN_POINT('Ctrl Pts',(65.4058436995807,248.365187254194,21.0856139599938)) ;
#115990=CARTESIAN_POINT('Ctrl Pts',(65.3285230624586,246.624886709414,21.6613048641929)) ;
#115991=CARTESIAN_POINT('Ctrl Pts',(65.2512024253364,246.119126056118,23.4233195575188)) ;
#115992=CARTESIAN_POINT('Ctrl Pts',(65.1738817882143,247.288380017986,24.8342756772788)) ;
#115993=CARTESIAN_POINT('Ctrl Pts',(65.0965611510921,249.114147404527,24.6653744652968)) ;
#115994=CARTESIAN_POINT('Ctrl Pts',(65.0192317351474,250.001268617604,23.0605218282742)) ;
#115995=CARTESIAN_POINT('Ctrl Pts',(64.96767586491,249.454365413351,21.9724776872887)) ;
#115996=CARTESIAN_POINT('Ctrl Pts',(64.9418935403801,249.012489323783,21.6574963150814)) ;
#115997=CARTESIAN_POINT('Ctrl Pts',(67.0508752479159,248.8090411595,24.6177774915559)) ;
#115998=CARTESIAN_POINT('Ctrl Pts',(67.0251017022085,249.326101584699,24.3687863597358)) ;
#115999=CARTESIAN_POINT('Ctrl Pts',(66.9735546107937,250.091649362878,23.3329896666175)) ;
#116000=CARTESIAN_POINT('Ctrl Pts',(66.8962339736716,249.455552685294,21.5005150565937)) ;
#116001=CARTESIAN_POINT('Ctrl Pts',(66.8189133365494,247.58251751521,20.9960107118432)) ;
#116002=CARTESIAN_POINT('Ctrl Pts',(66.7415926994272,246.109731882509,22.2566488562179)) ;
#116003=CARTESIAN_POINT('Ctrl Pts',(66.664272062305,246.320050600704,24.1845783818171)) ;
#116004=CARTESIAN_POINT('Ctrl Pts',(66.5869514251829,248.03081053473,25.097799355474)) ;
#116005=CARTESIAN_POINT('Ctrl Pts',(66.5096307880607,249.749706789539,24.2002000989301)) ;
#116006=CARTESIAN_POINT('Ctrl Pts',(66.4323101509385,249.977834734421,22.2744453785871)) ;
#116007=CARTESIAN_POINT('Ctrl Pts',(66.3549895138164,248.516170424749,21.0000661792743)) ;
#116008=CARTESIAN_POINT('Ctrl Pts',(66.2776688766941,246.639475807283,21.4884289128503)) ;
#116009=CARTESIAN_POINT('Ctrl Pts',(66.200348239572,245.984415549573,23.3136423671894)) ;
#116010=CARTESIAN_POINT('Ctrl Pts',(66.1230276024498,247.122279781611,24.8839175681433)) ;
#116011=CARTESIAN_POINT('Ctrl Pts',(66.0457069653276,249.060725056939,24.8298082037237)) ;
#116012=CARTESIAN_POINT('Ctrl Pts',(65.9683863282055,250.109219875687,23.1985022968723)) ;
#116013=CARTESIAN_POINT('Ctrl Pts',(65.8910656910833,249.353362873302,21.4126746068038)) ;
#116014=CARTESIAN_POINT('Ctrl Pts',(65.8137450539611,247.452343653537,21.029759688261)) ;
#116015=CARTESIAN_POINT('Ctrl Pts',(65.7364244168389,246.06405438661,22.3836991731043)) ;
#116016=CARTESIAN_POINT('Ctrl Pts',(65.6591037797168,246.399235599297,24.2937153117255)) ;
#116017=CARTESIAN_POINT('Ctrl Pts',(65.5817831425946,248.165567307768,25.0940609510727)) ;
#116018=CARTESIAN_POINT('Ctrl Pts',(65.5044625054724,249.822630639067,24.0867645627768)) ;
#116019=CARTESIAN_POINT('Ctrl Pts',(65.4271418683502,249.925260155198,22.1502623591688)) ;
#116020=CARTESIAN_POINT('Ctrl Pts',(65.3498212312281,248.384011495629,20.9734695441316)) ;
#116021=CARTESIAN_POINT('Ctrl Pts',(65.2725005941059,246.542887298214,21.5825128827272)) ;
#116022=CARTESIAN_POINT('Ctrl Pts',(65.1951799569837,246.00782559311,23.4466092296557)) ;
#116023=CARTESIAN_POINT('Ctrl Pts',(65.1178593198615,247.244819840209,24.9393085575803)) ;
#116024=CARTESIAN_POINT('Ctrl Pts',(65.0405386827393,249.176362368478,24.7606221178815)) ;
#116025=CARTESIAN_POINT('Ctrl Pts',(64.9632092667947,250.11487861289,23.0627929514371)) ;
#116026=CARTESIAN_POINT('Ctrl Pts',(64.9116533965574,249.536290778729,21.9117133854207)) ;
#116027=CARTESIAN_POINT('Ctrl Pts',(64.8858710720275,249.068814765345,21.578483686766)) ;
#116028=CARTESIAN_POINT('Ctrl Pts',(66.9948527795633,248.851140877543,24.7052026859895)) ;
#116029=CARTESIAN_POINT('Ctrl Pts',(66.9690792338559,249.396516568368,24.4425763005461)) ;
#116030=CARTESIAN_POINT('Ctrl Pts',(66.9175321424411,250.203987277857,23.3500573036672)) ;
#116031=CARTESIAN_POINT('Ctrl Pts',(66.840211505319,249.53305667079,21.4172327097574)) ;
#116032=CARTESIAN_POINT('Ctrl Pts',(66.7628908681968,247.557450339225,20.8851006955216)) ;
#116033=CARTESIAN_POINT('Ctrl Pts',(66.6855702310746,246.004012012238,22.2147739123507)) ;
#116034=CARTESIAN_POINT('Ctrl Pts',(66.6082495939524,246.225848205145,24.2482807244066)) ;
#116035=CARTESIAN_POINT('Ctrl Pts',(66.5309289568302,248.030292783352,25.2115115096535)) ;
#116036=CARTESIAN_POINT('Ctrl Pts',(66.4536083197081,249.843319243583,24.2647579180714)) ;
#116037=CARTESIAN_POINT('Ctrl Pts',(66.3762876825859,250.08393993214,22.2335450079682)) ;
#116038=CARTESIAN_POINT('Ctrl Pts',(66.2989670454638,248.54223195413,20.8893782484808)) ;
#116039=CARTESIAN_POINT('Ctrl Pts',(66.2216464083415,246.562765776506,21.4044847045491)) ;
#116040=CARTESIAN_POINT('Ctrl Pts',(66.1443257712194,245.871833105641,23.3296505073297)) ;
#116041=CARTESIAN_POINT('Ctrl Pts',(66.0670051340972,247.072009064524,24.9859171268005)) ;
#116042=CARTESIAN_POINT('Ctrl Pts',(65.989684496975,249.116607489848,24.9288446250921)) ;
#116043=CARTESIAN_POINT('Ctrl Pts',(65.9123638598528,250.222519987177,23.208205135898)) ;
#116044=CARTESIAN_POINT('Ctrl Pts',(65.8350432227307,249.425270739795,21.3245819408107)) ;
#116045=CARTESIAN_POINT('Ctrl Pts',(65.7577225856085,247.420147895879,20.9206978335572)) ;
#116046=CARTESIAN_POINT('Ctrl Pts',(65.6804019484863,245.955833125076,22.3487817593347)) ;
#116047=CARTESIAN_POINT('Ctrl Pts',(65.6030813113641,246.309369533032,24.3633942114241)) ;
#116048=CARTESIAN_POINT('Ctrl Pts',(65.525760674242,248.172429107479,25.2075683827315)) ;
#116049=CARTESIAN_POINT('Ctrl Pts',(65.4484400371198,249.920236549329,24.1451104245121)) ;
#116050=CARTESIAN_POINT('Ctrl Pts',(65.3711193999976,250.028486263541,22.1025614774108)) ;
#116051=CARTESIAN_POINT('Ctrl Pts',(65.2937987628754,248.402835737063,20.8613251282695)) ;
#116052=CARTESIAN_POINT('Ctrl Pts',(65.2164781257533,246.460887887013,21.5037209012614)) ;
#116053=CARTESIAN_POINT('Ctrl Pts',(65.1391574886311,245.896525130101,23.4698989017926)) ;
#116054=CARTESIAN_POINT('Ctrl Pts',(65.0618368515089,247.201259662433,25.044341437882)) ;
#116055=CARTESIAN_POINT('Ctrl Pts',(64.9845162143867,249.238577332429,24.8558697704663)) ;
#116056=CARTESIAN_POINT('Ctrl Pts',(64.907186798442,250.228488608176,23.0650640745999)) ;
#116057=CARTESIAN_POINT('Ctrl Pts',(64.8556309282047,249.618216144106,21.8509490835528)) ;
#116058=CARTESIAN_POINT('Ctrl Pts',(64.8298486036748,249.125140206909,21.4994710584505)) ;
#116059=CARTESIAN_POINT('Ctrl Pts',(66.9388303112106,248.893240595586,24.7926278804231)) ;
#116060=CARTESIAN_POINT('Ctrl Pts',(66.9130567655032,249.466931552037,24.5163662413563)) ;
#116061=CARTESIAN_POINT('Ctrl Pts',(66.8615096740885,250.316325192836,23.3671249407168)) ;
#116062=CARTESIAN_POINT('Ctrl Pts',(66.7841890369662,249.610560656286,21.3339503629212)) ;
#116063=CARTESIAN_POINT('Ctrl Pts',(66.7068683998441,247.532383163238,20.7741906792)) ;
#116064=CARTESIAN_POINT('Ctrl Pts',(66.6295477627219,245.898292141966,22.1728989684836)) ;
#116065=CARTESIAN_POINT('Ctrl Pts',(66.5522271255997,246.131645809585,24.3119830669961)) ;
#116066=CARTESIAN_POINT('Ctrl Pts',(66.4749064884777,248.029775031975,25.3252236638329)) ;
#116067=CARTESIAN_POINT('Ctrl Pts',(66.3975858513554,249.936931697627,24.3293157372126)) ;
#116068=CARTESIAN_POINT('Ctrl Pts',(66.3202652142332,250.190045129858,22.1926446373492)) ;
#116069=CARTESIAN_POINT('Ctrl Pts',(66.2429445771111,248.568293483511,20.7786903176872)) ;
#116070=CARTESIAN_POINT('Ctrl Pts',(66.1656239399888,246.486055745729,21.3205404962479)) ;
#116071=CARTESIAN_POINT('Ctrl Pts',(66.0883033028667,245.75925066171,23.3456586474699)) ;
#116072=CARTESIAN_POINT('Ctrl Pts',(66.0109826657445,247.021738347437,25.0879166854576)) ;
#116073=CARTESIAN_POINT('Ctrl Pts',(65.9336620286223,249.172489922758,25.0278810464605)) ;
#116074=CARTESIAN_POINT('Ctrl Pts',(65.8563413915001,250.335820098668,23.2179079749237)) ;
#116075=CARTESIAN_POINT('Ctrl Pts',(65.7790207543779,249.497178606289,21.2364892748176)) ;
#116076=CARTESIAN_POINT('Ctrl Pts',(65.7017001172558,247.387952138219,20.8116359788532)) ;
#116077=CARTESIAN_POINT('Ctrl Pts',(65.6243794801336,245.847611863543,22.313864345565)) ;
#116078=CARTESIAN_POINT('Ctrl Pts',(65.5470588430114,246.219503466767,24.4330731111226)) ;
#116079=CARTESIAN_POINT('Ctrl Pts',(65.4697382058892,248.17929090719,25.3210758143902)) ;
#116080=CARTESIAN_POINT('Ctrl Pts',(65.3924175687671,250.01784245959,24.2034562862473)) ;
#116081=CARTESIAN_POINT('Ctrl Pts',(65.3150969316449,250.131712371886,22.0548605956528)) ;
#116082=CARTESIAN_POINT('Ctrl Pts',(65.2377762945227,248.421659978497,20.7491807124074)) ;
#116083=CARTESIAN_POINT('Ctrl Pts',(65.1604556574006,246.378888475813,21.4249289197957)) ;
#116084=CARTESIAN_POINT('Ctrl Pts',(65.0831350202784,245.785224667093,23.4931885739294)) ;
#116085=CARTESIAN_POINT('Ctrl Pts',(65.0058143831562,247.157699484657,25.1493743181835)) ;
#116086=CARTESIAN_POINT('Ctrl Pts',(64.9284937460341,249.30079229638,24.951117423051)) ;
#116087=CARTESIAN_POINT('Ctrl Pts',(64.8511643300893,250.342098603462,23.0673351977628)) ;
#116088=CARTESIAN_POINT('Ctrl Pts',(64.7996084598521,249.700141509485,21.7901847816847)) ;
#116089=CARTESIAN_POINT('Ctrl Pts',(64.7738261353222,249.181465648471,21.4204584301351)) ;
#116090=CARTESIAN_POINT('',(66.940838214598,249.015862219827,21.6551782011097)) ;
#116091=CARTESIAN_POINT('Ctrl Pts',(66.9402651077866,249.016486567286,21.6543968495755)) ;
#116092=CARTESIAN_POINT('Ctrl Pts',(66.9402651077865,249.073326496225,21.6877083848151)) ;
#116093=CARTESIAN_POINT('Ctrl Pts',(66.9402651077866,249.127953344347,21.724365048829)) ;
#116094=CARTESIAN_POINT('Ctrl Pts',(66.9402651077866,249.180013147505,21.764281136914)) ;
#116095=CARTESIAN_POINT('Ctrl Pts',(66.9402651077866,249.185825850241,21.7687379412113)) ;
#116096=CARTESIAN_POINT('Ctrl Pts',(66.9402651077866,249.191606536244,21.7732354314043)) ;
#116097=CARTESIAN_POINT('Ctrl Pts',(66.9402651077866,249.197354700228,21.7777735269277)) ;
#116098=CARTESIAN_POINT('Ctrl Pts',(66.9402651077867,249.232037725852,21.805155293308)) ;
#116099=CARTESIAN_POINT('Ctrl Pts',(66.9402651077866,249.265537259157,21.8340144840013)) ;
#116100=CARTESIAN_POINT('Ctrl Pts',(66.9402651077867,249.297829631273,21.8642422084135)) ;
#116101=CARTESIAN_POINT('Ctrl Pts',(66.9402651077867,249.316655489125,21.8818644147024)) ;
#116102=CARTESIAN_POINT('Ctrl Pts',(66.9402651077866,249.335070957522,21.8999519442239)) ;
#116103=CARTESIAN_POINT('Ctrl Pts',(66.9402651077866,249.353070286022,21.9184847523711)) ;
#116104=CARTESIAN_POINT('Ctrl Pts',(66.9402651077866,249.362805032771,21.9285080259532)) ;
#116105=CARTESIAN_POINT('Ctrl Pts',(66.9402651077867,249.372418273226,21.9386619930784)) ;
#116106=CARTESIAN_POINT('Ctrl Pts',(66.9402651077867,249.381898613883,21.9489318295471)) ;
#116107=CARTESIAN_POINT('Ctrl Pts',(66.9402651077867,249.426416304368,21.9971568267049)) ;
#116108=CARTESIAN_POINT('Ctrl Pts',(66.9402651077866,249.468064105244,22.0479919324255)) ;
#116109=CARTESIAN_POINT('Ctrl Pts',(66.9402651077865,249.506774354067,22.1010784154893)) ;
#116110=CARTESIAN_POINT('Ctrl Pts',(66.9402651077865,249.537894530784,22.1437560211474)) ;
#116111=CARTESIAN_POINT('Ctrl Pts',(66.9402651077868,249.567115779311,22.1878898641801)) ;
#116112=CARTESIAN_POINT('Ctrl Pts',(66.9402651077867,249.594387845524,22.2333127182412)) ;
#116113=CARTESIAN_POINT('Ctrl Pts',(66.9402651077867,249.60355415791,22.2485796241852)) ;
#116114=CARTESIAN_POINT('Ctrl Pts',(66.9402651077866,249.612500152114,22.2639922675129)) ;
#116115=CARTESIAN_POINT('Ctrl Pts',(66.9402651077866,249.621223526897,22.2795446374933)) ;
#116116=CARTESIAN_POINT('Ctrl Pts',(66.9402651077866,249.628650964169,22.2927865599521)) ;
#116117=CARTESIAN_POINT('Ctrl Pts',(66.9402651077864,249.635917917401,22.306131792565)) ;
#116118=CARTESIAN_POINT('Ctrl Pts',(66.9402651077865,249.643012373558,22.3195560085153)) ;
#116119=CARTESIAN_POINT('Ctrl Pts',(66.9402651077868,249.67462025506,22.379364825088)) ;
#116120=CARTESIAN_POINT('Ctrl Pts',(66.9402651077865,249.702856359346,22.4408238062802)) ;
#116121=CARTESIAN_POINT('Ctrl Pts',(66.9402651077866,249.727647936966,22.5035717822936)) ;
#116122=CARTESIAN_POINT('Ctrl Pts',(66.9402651077866,249.752833032827,22.5673157608029)) ;
#116123=CARTESIAN_POINT('Ctrl Pts',(66.9402651077865,249.774463981167,22.6323908538163)) ;
#116124=CARTESIAN_POINT('Ctrl Pts',(66.9402651077865,249.792424717225,22.6984537299751)) ;
#116125=CARTESIAN_POINT('Ctrl Pts',(66.9402651077865,249.805624202608,22.747003854278)) ;
#116126=CARTESIAN_POINT('Ctrl Pts',(66.9402651077867,249.816840654164,22.7960882766413)) ;
#116127=CARTESIAN_POINT('Ctrl Pts',(66.9402651077866,249.82601175431,22.8455782779415)) ;
#116128=CARTESIAN_POINT('Ctrl Pts',(66.9402651077866,249.831235060844,22.8737648033397)) ;
#116129=CARTESIAN_POINT('Ctrl Pts',(66.9402651077864,249.835794641495,22.9020829818254)) ;
#116130=CARTESIAN_POINT('Ctrl Pts',(66.9402651077865,249.839676741179,22.9305095007077)) ;
#116131=CARTESIAN_POINT('Ctrl Pts',(66.9402651077865,249.841634274688,22.9448434611364)) ;
#116132=CARTESIAN_POINT('Ctrl Pts',(66.9402651077866,249.843419764806,22.9592082750519)) ;
#116133=CARTESIAN_POINT('Ctrl Pts',(66.9402651077866,249.845028811054,22.9735755074892)) ;
#116134=CARTESIAN_POINT('Ctrl Pts',(66.9402651077866,249.852811679582,23.0430690234714)) ;
#116135=CARTESIAN_POINT('Ctrl Pts',(66.9402651077867,249.856487909412,23.1127330448471)) ;
#116136=CARTESIAN_POINT('Ctrl Pts',(66.9402651077867,249.855949939848,23.1822119034766)) ;
#116137=CARTESIAN_POINT('Ctrl Pts',(66.9402651077867,249.85565787284,23.2199324061758)) ;
#116138=CARTESIAN_POINT('Ctrl Pts',(66.9402651077866,249.854122900981,23.2575987848212)) ;
#116139=CARTESIAN_POINT('Ctrl Pts',(66.9402651077866,249.851321755643,23.295156346524)) ;
#116140=CARTESIAN_POINT('Ctrl Pts',(66.9402651077866,249.846296248548,23.3625379958313)) ;
#116141=CARTESIAN_POINT('Ctrl Pts',(66.9402651077866,249.837198429191,23.429569569572)) ;
#116142=CARTESIAN_POINT('Ctrl Pts',(66.9402651077864,249.824246229587,23.496008686096)) ;
#116143=CARTESIAN_POINT('Ctrl Pts',(66.9402651077863,249.817734272897,23.5294121745024)) ;
#116144=CARTESIAN_POINT('Ctrl Pts',(66.9402651077864,249.810247185901,23.5626659184175)) ;
#116145=CARTESIAN_POINT('Ctrl Pts',(66.9402651077865,249.801807841976,23.5957386910865)) ;
#116146=CARTESIAN_POINT('Ctrl Pts',(66.9402651077865,249.797664050485,23.6119777109885)) ;
#116147=CARTESIAN_POINT('Ctrl Pts',(66.9402651077864,249.793290632525,23.6281730922088)) ;
#116148=CARTESIAN_POINT('Ctrl Pts',(66.9402651077864,249.788690029188,23.6443210746468)) ;
#116149=CARTESIAN_POINT('Ctrl Pts',(66.9402651077864,249.785823394845,23.6543828769038)) ;
#116150=CARTESIAN_POINT('Ctrl Pts',(66.9402651077864,249.782869245611,23.6644236622611)) ;
#116151=CARTESIAN_POINT('Ctrl Pts',(66.9402651077864,249.779830899714,23.6744343939138)) ;
#116152=CARTESIAN_POINT('Ctrl Pts',(66.9402651077865,249.759680252296,23.7408266779849)) ;
#116153=CARTESIAN_POINT('Ctrl Pts',(66.9402651077866,249.735801164671,23.8060012765027)) ;
#116154=CARTESIAN_POINT('Ctrl Pts',(66.9402651077866,249.708456355635,23.8697084272248)) ;
#116155=CARTESIAN_POINT('Ctrl Pts',(66.9402651077865,249.680373402716,23.9351352843627)) ;
#116156=CARTESIAN_POINT('Ctrl Pts',(66.9402651077866,249.648634875389,23.9990152885733)) ;
#116157=CARTESIAN_POINT('Ctrl Pts',(66.9402651077865,249.613469833398,24.0610737847212)) ;
#116158=CARTESIAN_POINT('Ctrl Pts',(66.9402651077864,249.578304791407,24.123132280869)) ;
#116159=CARTESIAN_POINT('Ctrl Pts',(66.9402651077865,249.539712760019,24.1833701962856)) ;
#116160=CARTESIAN_POINT('Ctrl Pts',(66.9402651077866,249.497873662861,24.2414950835056)) ;
#116161=CARTESIAN_POINT('Ctrl Pts',(66.9402651077866,249.487594016516,24.255776062901)) ;
#116162=CARTESIAN_POINT('Ctrl Pts',(66.9402651077866,249.477118144931,24.2699293657298)) ;
#116163=CARTESIAN_POINT('Ctrl Pts',(66.9402651077867,249.466448313562,24.2839503894272)) ;
#116164=CARTESIAN_POINT('Ctrl Pts',(66.9402651077867,249.457810767089,24.2953008259602)) ;
#116165=CARTESIAN_POINT('Ctrl Pts',(66.9402651077867,249.449044616362,24.3065662610333)) ;
#116166=CARTESIAN_POINT('Ctrl Pts',(66.9402651077867,249.440165554696,24.3177264493437)) ;
#116167=CARTESIAN_POINT('Ctrl Pts',(66.9402651077865,249.394575708576,24.3750288183199)) ;
#116168=CARTESIAN_POINT('Ctrl Pts',(66.9402651077866,249.345936065014,24.429661644788)) ;
#116169=CARTESIAN_POINT('Ctrl Pts',(66.9402651077866,249.294489733256,24.4813467525077)) ;
#116170=CARTESIAN_POINT('Ctrl Pts',(66.9402651077867,249.243099989585,24.5329750095)) ;
#116171=CARTESIAN_POINT('Ctrl Pts',(66.9402651077866,249.188909199461,24.5816629631761)) ;
#116172=CARTESIAN_POINT('Ctrl Pts',(66.9402651077867,249.132113281926,24.6271104778317)) ;
#116173=CARTESIAN_POINT('Ctrl Pts',(66.9402651077867,249.076718656809,24.6714366925687)) ;
#116174=CARTESIAN_POINT('Ctrl Pts',(66.9402651077867,249.018845246814,24.7126811366689)) ;
#116175=CARTESIAN_POINT('Ctrl Pts',(66.9402651077867,248.958639392982,24.7505314295909)) ;
#116176=CARTESIAN_POINT('Ctrl Pts',(66.9402651077867,248.936785980341,24.764270260903)) ;
#116177=CARTESIAN_POINT('Ctrl Pts',(66.9402651077868,248.914624961358,24.7775615184723)) ;
#116178=CARTESIAN_POINT('Ctrl Pts',(66.9402651077866,248.892162375845,24.7903888257488)) ;
#116179=CARTESIAN_POINT('Ctrl Pts',(66.940838214598,249.015292748841,21.6559756392158)) ;
#116180=CARTESIAN_POINT('Ctrl Pts',(66.9406471789942,249.009383798495,21.6517559063544)) ;
#116181=CARTESIAN_POINT('Ctrl Pts',(66.9404561433903,249.003447454475,21.6475745332417)) ;
#116182=CARTESIAN_POINT('Ctrl Pts',(66.9402651077865,248.99748421711,21.6434318722943)) ;
#116183=CARTESIAN_POINT('Origin',(66.9402651077866,248.040265107786,23.0213203435596)) ;
#116184=CARTESIAN_POINT('Ctrl Pts',(66.9402651077866,247.154495177753,24.7736741551652)) ;
#116185=CARTESIAN_POINT('Ctrl Pts',(66.9402651077866,247.103652956155,24.7437896484996)) ;
#116186=CARTESIAN_POINT('Ctrl Pts',(66.9402651077865,247.054326565403,24.7115704134065)) ;
#116187=CARTESIAN_POINT('Ctrl Pts',(66.9402651077866,247.006709671402,24.6770177424811)) ;
#116188=CARTESIAN_POINT('Ctrl Pts',(66.9402651077866,246.995903081062,24.6691760600765)) ;
#116189=CARTESIAN_POINT('Ctrl Pts',(66.9402651077867,246.98518460422,24.6612141158822)) ;
#116190=CARTESIAN_POINT('Ctrl Pts',(66.9402651077867,246.974556625495,24.6531317919492)) ;
#116191=CARTESIAN_POINT('Ctrl Pts',(66.9402651077867,246.914058226574,24.6071242047902)) ;
#116192=CARTESIAN_POINT('Ctrl Pts',(66.9402651077865,246.856488059237,24.5572187595307)) ;
#116193=CARTESIAN_POINT('Ctrl Pts',(66.9402651077866,246.802033735395,24.5038023506277)) ;
#116194=CARTESIAN_POINT('Ctrl Pts',(66.9402651077866,246.788205445077,24.4902376314661)) ;
#116195=CARTESIAN_POINT('Ctrl Pts',(66.9402651077866,246.774575314523,24.4764429382347)) ;
#116196=CARTESIAN_POINT('Ctrl Pts',(66.9402651077866,246.761166700878,24.4624455931476)) ;
#116197=CARTESIAN_POINT('Ctrl Pts',(66.9402651077867,246.71119450402,24.4102792691181)) ;
#116198=CARTESIAN_POINT('Ctrl Pts',(66.9402651077868,246.664243414614,24.355252107392)) ;
#116199=CARTESIAN_POINT('Ctrl Pts',(66.9402651077866,246.620453661835,24.2977129946242)) ;
#116200=CARTESIAN_POINT('Ctrl Pts',(66.9402651077865,246.586910564207,24.25363784109)) ;
#116201=CARTESIAN_POINT('Ctrl Pts',(66.9402651077868,246.555223195075,24.208087875639)) ;
#116202=CARTESIAN_POINT('Ctrl Pts',(66.9402651077866,246.525473022933,24.1612106032007)) ;
#116203=CARTESIAN_POINT('Ctrl Pts',(66.9402651077865,246.514224422105,24.1434862107816)) ;
#116204=CARTESIAN_POINT('Ctrl Pts',(66.9402651077867,246.503252938138,24.1255720078574)) ;
#116205=CARTESIAN_POINT('Ctrl Pts',(66.9402651077867,246.492563623701,24.1074758054361)) ;
#116206=CARTESIAN_POINT('Ctrl Pts',(66.9402651077868,246.483498928947,24.0921299614971)) ;
#116207=CARTESIAN_POINT('Ctrl Pts',(66.9402651077866,246.474634674195,24.0766484728284)) ;
#116208=CARTESIAN_POINT('Ctrl Pts',(66.9402651077865,246.465989099807,24.061063887127)) ;
#116209=CARTESIAN_POINT('Ctrl Pts',(66.9402651077865,246.43137542783,23.9986689885137)) ;
#116210=CARTESIAN_POINT('Ctrl Pts',(66.9402651077865,246.40021892318,23.9345528025734)) ;
#116211=CARTESIAN_POINT('Ctrl Pts',(66.9402651077865,246.372655883232,23.8690436799177)) ;
#116212=CARTESIAN_POINT('Ctrl Pts',(66.9402651077865,246.345545564146,23.8046105396851)) ;
#116213=CARTESIAN_POINT('Ctrl Pts',(66.9402651077867,246.321911425932,23.7388288418451)) ;
#116214=CARTESIAN_POINT('Ctrl Pts',(66.9402651077866,246.301930632325,23.6719979398038)) ;
#116215=CARTESIAN_POINT('Ctrl Pts',(66.9402651077865,246.287075345967,23.6223106147206)) ;
#116216=CARTESIAN_POINT('Ctrl Pts',(66.9402651077867,246.274240423999,23.572042994202)) ;
#116217=CARTESIAN_POINT('Ctrl Pts',(66.9402651077865,246.263517215067,23.5213180960051)) ;
#116218=CARTESIAN_POINT('Ctrl Pts',(66.9402651077864,246.257462981285,23.4926792441283)) ;
#116219=CARTESIAN_POINT('Ctrl Pts',(66.9402651077865,246.252082179617,23.4638946519576)) ;
#116220=CARTESIAN_POINT('Ctrl Pts',(66.9402651077865,246.247393636855,23.4349868862611)) ;
#116221=CARTESIAN_POINT('Ctrl Pts',(66.9402651077865,246.245447752022,23.4229893028557)) ;
#116222=CARTESIAN_POINT('Ctrl Pts',(66.9402651077865,246.243620819294,23.4109682962387)) ;
#116223=CARTESIAN_POINT('Ctrl Pts',(66.9402651077865,246.241915270405,23.398932592043)) ;
#116224=CARTESIAN_POINT('Ctrl Pts',(66.9402651077866,246.232360838049,23.3315089477653)) ;
#116225=CARTESIAN_POINT('Ctrl Pts',(66.9402651077867,246.226640800444,23.2638409239364)) ;
#116226=CARTESIAN_POINT('Ctrl Pts',(66.9402651077867,246.22490925737,23.1962106118006)) ;
#116227=CARTESIAN_POINT('Ctrl Pts',(66.9402651077867,246.223737339853,23.1504380585975)) ;
#116228=CARTESIAN_POINT('Ctrl Pts',(66.9402651077867,246.224393419138,23.1046826059687)) ;
#116229=CARTESIAN_POINT('Ctrl Pts',(66.9402651077866,246.226938877851,23.059032520807)) ;
#116230=CARTESIAN_POINT('Ctrl Pts',(66.9402651077863,246.230859305516,22.98872383506)) ;
#116231=CARTESIAN_POINT('Ctrl Pts',(66.9402651077865,246.239259307967,22.9186636658731)) ;
#116232=CARTESIAN_POINT('Ctrl Pts',(66.9402651077866,246.251951677252,22.8491862047465)) ;
#116233=CARTESIAN_POINT('Ctrl Pts',(66.9402651077867,246.257504588814,22.8187898155036)) ;
#116234=CARTESIAN_POINT('Ctrl Pts',(66.9402651077866,246.263879774033,22.7885052567041)) ;
#116235=CARTESIAN_POINT('Ctrl Pts',(66.9402651077865,246.271064532401,22.7583622459574)) ;
#116236=CARTESIAN_POINT('Ctrl Pts',(66.9402651077865,246.274140059972,22.7454591452704)) ;
#116237=CARTESIAN_POINT('Ctrl Pts',(66.9402651077867,246.277363952684,22.7325819973825)) ;
#116238=CARTESIAN_POINT('Ctrl Pts',(66.9402651077866,246.28073530438,22.7197332095146)) ;
#116239=CARTESIAN_POINT('Ctrl Pts',(66.9402651077864,246.283642677311,22.7086527226913)) ;
#116240=CARTESIAN_POINT('Ctrl Pts',(66.9402651077864,246.286659754245,22.6975935420638)) ;
#116241=CARTESIAN_POINT('Ctrl Pts',(66.9402651077865,246.289781818403,22.6865708935598)) ;
#116242=CARTESIAN_POINT('Ctrl Pts',(66.9402651077866,246.308212817329,22.6214990652872)) ;
#116243=CARTESIAN_POINT('Ctrl Pts',(66.9402651077864,246.330329981973,22.5575763200012)) ;
#116244=CARTESIAN_POINT('Ctrl Pts',(66.9402651077865,246.355929917223,22.4950833743233)) ;
#116245=CARTESIAN_POINT('Ctrl Pts',(66.9402651077867,246.381601825482,22.4324147326794)) ;
#116246=CARTESIAN_POINT('Ctrl Pts',(66.9402651077865,246.410776743819,22.3711830368571)) ;
#116247=CARTESIAN_POINT('Ctrl Pts',(66.9402651077865,246.443295194883,22.3116966484315)) ;
#116248=CARTESIAN_POINT('Ctrl Pts',(66.9402651077865,246.475305053119,22.2531406349017)) ;
#116249=CARTESIAN_POINT('Ctrl Pts',(66.9402651077865,246.510555356463,22.196275020944)) ;
#116250=CARTESIAN_POINT('Ctrl Pts',(66.9402651077864,246.54892824794,22.141430434894)) ;
#116251=CARTESIAN_POINT('Ctrl Pts',(66.9402651077864,246.556635945235,22.1304141822409)) ;
#116252=CARTESIAN_POINT('Ctrl Pts',(66.9402651077867,246.564469719844,22.1194796099464)) ;
#116253=CARTESIAN_POINT('Ctrl Pts',(66.9402651077867,246.572428750125,22.1086296193694)) ;
#116254=CARTESIAN_POINT('Ctrl Pts',(66.9402651077867,246.579356337263,22.0991857232521)) ;
#116255=CARTESIAN_POINT('Ctrl Pts',(66.9402651077867,246.586379350469,22.0898053636188)) ;
#116256=CARTESIAN_POINT('Ctrl Pts',(66.9402651077866,246.593487201128,22.0805032329674)) ;
#116257=CARTESIAN_POINT('Ctrl Pts',(66.9402651077865,246.633609374762,22.0279948560982)) ;
#116258=CARTESIAN_POINT('Ctrl Pts',(66.9402651077865,246.676503733551,21.977876472155)) ;
#116259=CARTESIAN_POINT('Ctrl Pts',(66.9402651077865,246.722014918924,21.930428698024)) ;
#116260=CARTESIAN_POINT('Ctrl Pts',(66.9402651077866,246.766261027012,21.884299832657)) ;
#116261=CARTESIAN_POINT('Ctrl Pts',(66.9402651077865,246.812981198213,21.8406946224787)) ;
#116262=CARTESIAN_POINT('Ctrl Pts',(66.9402651077866,246.862061994689,21.7999086912144)) ;
#116263=CARTESIAN_POINT('Ctrl Pts',(66.9402651077866,246.910681941446,21.7595057240879)) ;
#116264=CARTESIAN_POINT('Ctrl Pts',(66.9402651077866,246.961618918586,21.7218687438548)) ;
#116265=CARTESIAN_POINT('Ctrl Pts',(66.9402651077866,247.014783014899,21.6873312777196)) ;
#116266=CARTESIAN_POINT('Ctrl Pts',(66.9402651077866,247.031608040966,21.6764010859492)) ;
#116267=CARTESIAN_POINT('Ctrl Pts',(66.9402651077867,247.048656247541,21.665781712902)) ;
#116268=CARTESIAN_POINT('Ctrl Pts',(66.9402651077866,247.065925086493,21.6554848536835)) ;
#116269=CARTESIAN_POINT('Ctrl Pts',(67.1066093021096,246.899167654978,21.4205873299757)) ;
#116270=CARTESIAN_POINT('Ctrl Pts',(67.0808268545257,246.380530910519,21.7902818863321)) ;
#116271=CARTESIAN_POINT('Ctrl Pts',(67.0292708612343,245.73862285314,23.0673282297465)) ;
#116272=CARTESIAN_POINT('Ctrl Pts',(66.9519413222356,246.779843576752,24.950955615441)) ;
#116273=CARTESIAN_POINT('Ctrl Pts',(66.8746206851134,248.922756726385,25.1491958853405)) ;
#116274=CARTESIAN_POINT('Ctrl Pts',(66.7973000479912,250.295116492069,23.4931490133159)) ;
#116275=CARTESIAN_POINT('Ctrl Pts',(66.7199794108692,249.701502455305,21.4250627499166)) ;
#116276=CARTESIAN_POINT('Ctrl Pts',(66.642658773747,247.658902211124,20.7493711995695)) ;
#116277=CARTESIAN_POINT('Ctrl Pts',(66.5653381366247,245.948993181706,22.0549416187025)) ;
#116278=CARTESIAN_POINT('Ctrl Pts',(66.4880174995025,246.062853547653,24.2033571811817)) ;
#116279=CARTESIAN_POINT('Ctrl Pts',(66.4106968623804,247.901250963731,25.3208830123917)) ;
#116280=CARTESIAN_POINT('Ctrl Pts',(66.3333762252582,249.860874103791,24.4329547557814)) ;
#116281=CARTESIAN_POINT('Ctrl Pts',(66.256055588136,250.23273452922,22.3139236556595)) ;
#116282=CARTESIAN_POINT('Ctrl Pts',(66.1787349510139,248.692523390174,20.8118212295067)) ;
#116283=CARTESIAN_POINT('Ctrl Pts',(66.1014143138918,246.583473750784,21.2366389075348)) ;
#116284=CARTESIAN_POINT('Ctrl Pts',(66.0240936767696,245.74490256657,23.2178914938439)) ;
#116285=CARTESIAN_POINT('Ctrl Pts',(65.9467730396473,246.908135213782,25.0277128248629)) ;
#116286=CARTESIAN_POINT('Ctrl Pts',(65.8694524025251,249.058706479129,25.0877434307034)) ;
#116287=CARTESIAN_POINT('Ctrl Pts',(65.792131765403,250.321088323227,23.3456314563494)) ;
#116288=CARTESIAN_POINT('Ctrl Pts',(65.7148111282808,249.59434417144,21.3206830824085)) ;
#116289=CARTESIAN_POINT('Ctrl Pts',(65.6374904911586,247.51228099978,20.7788783305243)) ;
#116290=CARTESIAN_POINT('Ctrl Pts',(65.5601698540364,245.890665314093,22.1927141098144)) ;
#116291=CARTESIAN_POINT('Ctrl Pts',(65.4828492169142,246.143757526522,24.3292060812583)) ;
#116292=CARTESIAN_POINT('Ctrl Pts',(65.4055285797921,248.050754303577,25.3250305138284)) ;
#116293=CARTESIAN_POINT('Ctrl Pts',(65.3282079426699,249.948724394557,24.3118748680936)) ;
#116294=CARTESIAN_POINT('Ctrl Pts',(65.2508873055477,250.182058496545,22.1729700982747)) ;
#116295=CARTESIAN_POINT('Ctrl Pts',(65.1735666684256,248.548104464289,20.7743790968438)) ;
#116296=CARTESIAN_POINT('Ctrl Pts',(65.0962460313034,246.470101190474,21.3340918495046)) ;
#116297=CARTESIAN_POINT('Ctrl Pts',(65.0189253941812,245.764395780262,23.3670960744596)) ;
#116298=CARTESIAN_POINT('Ctrl Pts',(64.9673783027664,246.613718254765,24.5162409181759)) ;
#116299=CARTESIAN_POINT('Ctrl Pts',(64.941604757059,247.187361121204,24.7924793994338)) ;
#116300=CARTESIAN_POINT('Ctrl Pts',(67.0506108178113,246.955468616385,21.4995663929808)) ;
#116301=CARTESIAN_POINT('Ctrl Pts',(67.0248283702273,246.46242105124,21.8510204748725)) ;
#116302=CARTESIAN_POINT('Ctrl Pts',(66.973272376936,245.852184294744,23.0650582323697)) ;
#116303=CARTESIAN_POINT('Ctrl Pts',(66.8959428379373,246.842031905892,24.8557487418266)) ;
#116304=CARTESIAN_POINT('Ctrl Pts',(66.8186222008151,248.879215198501,25.0442079735181)) ;
#116305=CARTESIAN_POINT('Ctrl Pts',(66.7413015636929,250.183863679742,23.469869312129)) ;
#116306=CARTESIAN_POINT('Ctrl Pts',(66.6639809265707,249.619538150188,21.503820998788)) ;
#116307=CARTESIAN_POINT('Ctrl Pts',(66.5866602894486,247.677718393453,20.86146760357)) ;
#116308=CARTESIAN_POINT('Ctrl Pts',(66.5093396523264,246.052175096372,22.1026220785603)) ;
#116309=CARTESIAN_POINT('Ctrl Pts',(66.4320190152043,246.160417670383,24.1450362987605)) ;
#116310=CARTESIAN_POINT('Ctrl Pts',(66.354698378082,247.908109825732,25.2074241761182)) ;
#116311=CARTESIAN_POINT('Ctrl Pts',(66.2773777409599,249.771046511443,24.3633056873628)) ;
#116312=CARTESIAN_POINT('Ctrl Pts',(66.2000571038377,250.12455959992,22.348826120411)) ;
#116313=CARTESIAN_POINT('Ctrl Pts',(66.1227364667155,248.660341416326,20.9208363920962)) ;
#116314=CARTESIAN_POINT('Ctrl Pts',(66.0454158295933,246.655350831718,21.3246938588499)) ;
#116315=CARTESIAN_POINT('Ctrl Pts',(65.9680951924712,245.858154171443,23.2081928088468)) ;
#116316=CARTESIAN_POINT('Ctrl Pts',(65.890774555349,246.963993722022,24.9287188034683)) ;
#116317=CARTESIAN_POINT('Ctrl Pts',(65.8134539182268,249.008457284197,24.9857875406145)) ;
#116318=CARTESIAN_POINT('Ctrl Pts',(65.7361332811046,250.208554078661,23.3296301696934)) ;
#116319=CARTESIAN_POINT('Ctrl Pts',(65.6588126439825,249.517666982151,21.4045913520933)) ;
#116320=CARTESIAN_POINT('Ctrl Pts',(65.5814920068603,247.538331371565,20.8895188730319)) ;
#116321=CARTESIAN_POINT('Ctrl Pts',(65.5041713697381,245.996725085524,22.2335969699703)) ;
#116322=CARTESIAN_POINT('Ctrl Pts',(65.4268507326159,246.237329902726,24.2646759008943)) ;
#116323=CARTESIAN_POINT('Ctrl Pts',(65.3495300954938,248.05023677389,25.2113670426942)) ;
#116324=CARTESIAN_POINT('Ctrl Pts',(65.2722094583716,249.854562329444,24.2481997978353)) ;
#116325=CARTESIAN_POINT('Ctrl Pts',(65.1948888212494,250.07638388775,22.2148271143443)) ;
#116326=CARTESIAN_POINT('Ctrl Pts',(65.1175681841272,248.523048020651,20.8852416284384)) ;
#116327=CARTESIAN_POINT('Ctrl Pts',(65.040247547005,246.547571995349,21.4173385398677)) ;
#116328=CARTESIAN_POINT('Ctrl Pts',(64.9629269098829,245.876685603414,23.3500357383482)) ;
#116329=CARTESIAN_POINT('Ctrl Pts',(64.9113798184681,246.684103092728,24.44248256794)) ;
#116330=CARTESIAN_POINT('Ctrl Pts',(64.8856062727607,247.22944281573,24.7050916330301)) ;
#116331=CARTESIAN_POINT('Ctrl Pts',(66.994612333513,247.011769577792,21.5785454559859)) ;
#116332=CARTESIAN_POINT('Ctrl Pts',(66.9688298859291,246.544311191959,21.9117590634128)) ;
#116333=CARTESIAN_POINT('Ctrl Pts',(66.9172738926377,245.965745736347,23.0627882349928)) ;
#116334=CARTESIAN_POINT('Ctrl Pts',(66.839944353639,246.904220235031,24.7605418682122)) ;
#116335=CARTESIAN_POINT('Ctrl Pts',(66.7626237165168,248.835673670616,24.9392200616958)) ;
#116336=CARTESIAN_POINT('Ctrl Pts',(66.6853030793946,250.072610867414,23.4465896109422)) ;
#116337=CARTESIAN_POINT('Ctrl Pts',(66.6079824422724,249.537573845071,21.5825792476595)) ;
#116338=CARTESIAN_POINT('Ctrl Pts',(66.5306618051503,247.696534575781,20.9735640075703)) ;
#116339=CARTESIAN_POINT('Ctrl Pts',(66.4533411680281,246.155357011037,22.1503025384181)) ;
#116340=CARTESIAN_POINT('Ctrl Pts',(66.3760205309059,246.257981793112,24.0867154163394)) ;
#116341=CARTESIAN_POINT('Ctrl Pts',(66.2986998937837,247.914968687735,25.0939653398447)) ;
#116342=CARTESIAN_POINT('Ctrl Pts',(66.2213792566616,249.681218919094,24.2936566189442)) ;
#116343=CARTESIAN_POINT('Ctrl Pts',(66.1440586195394,250.01638467062,22.3837285851626)) ;
#116344=CARTESIAN_POINT('Ctrl Pts',(66.0667379824172,248.628159442479,21.0298515546859)) ;
#116345=CARTESIAN_POINT('Ctrl Pts',(65.989417345295,246.72722791265,21.4127488101651)) ;
#116346=CARTESIAN_POINT('Ctrl Pts',(65.9120967081729,245.971405776317,23.1984941238496)) ;
#116347=CARTESIAN_POINT('Ctrl Pts',(65.8347760710507,247.019852230261,24.8297247820737)) ;
#116348=CARTESIAN_POINT('Ctrl Pts',(65.7574554339285,248.958208089265,24.8838316505256)) ;
#116349=CARTESIAN_POINT('Ctrl Pts',(65.6801347968063,250.096019834095,23.3136288830372)) ;
#116350=CARTESIAN_POINT('Ctrl Pts',(65.6028141596841,249.440989792863,21.4884996217781)) ;
#116351=CARTESIAN_POINT('Ctrl Pts',(65.525493522562,247.564381743349,21.0001594155395)) ;
#116352=CARTESIAN_POINT('Ctrl Pts',(65.4481728854398,246.102784856954,22.2744798301262)) ;
#116353=CARTESIAN_POINT('Ctrl Pts',(65.3708522483176,246.330902278931,24.2001457205304)) ;
#116354=CARTESIAN_POINT('Ctrl Pts',(65.2935316111954,248.049719244203,25.09770357156)) ;
#116355=CARTESIAN_POINT('Ctrl Pts',(65.2162109740733,249.760400264332,24.1845247275771)) ;
#116356=CARTESIAN_POINT('Ctrl Pts',(65.1388903369511,249.970709278956,22.2566841304139)) ;
#116357=CARTESIAN_POINT('Ctrl Pts',(65.0615696998289,248.497991577014,20.9961041600331)) ;
#116358=CARTESIAN_POINT('Ctrl Pts',(64.9842490627067,246.625042800225,21.500585230231)) ;
#116359=CARTESIAN_POINT('Ctrl Pts',(64.9069284255846,245.988975426567,23.3329754022367)) ;
#116360=CARTESIAN_POINT('Ctrl Pts',(64.8553813341698,246.754487930692,24.3687242177039)) ;
#116361=CARTESIAN_POINT('Ctrl Pts',(64.8296077884624,247.271524510254,24.6177038666263)) ;
#116362=CARTESIAN_POINT('Ctrl Pts',(66.9386138492147,247.068070539199,21.6575245189909)) ;
#116363=CARTESIAN_POINT('Ctrl Pts',(66.9128314016307,246.62620133268,21.9724976519531)) ;
#116364=CARTESIAN_POINT('Ctrl Pts',(66.8612754083394,246.079307177951,23.0605182376159)) ;
#116365=CARTESIAN_POINT('Ctrl Pts',(66.7839458693407,246.966408564169,24.6653349945978)) ;
#116366=CARTESIAN_POINT('Ctrl Pts',(66.7066252322185,248.792132142731,24.8342321498734)) ;
#116367=CARTESIAN_POINT('Ctrl Pts',(66.6293045950963,249.961358055087,23.4233099097552)) ;
#116368=CARTESIAN_POINT('Ctrl Pts',(66.5519839579741,249.455609539954,21.661337496531)) ;
#116369=CARTESIAN_POINT('Ctrl Pts',(66.4746633208519,247.71535075811,21.0856604115707)) ;
#116370=CARTESIAN_POINT('Ctrl Pts',(66.3973426837298,246.258538925704,22.1979829982759)) ;
#116371=CARTESIAN_POINT('Ctrl Pts',(66.3200220466076,246.355545915842,24.0283945339182)) ;
#116372=CARTESIAN_POINT('Ctrl Pts',(66.2427014094854,247.921827549737,24.9805065035713)) ;
#116373=CARTESIAN_POINT('Ctrl Pts',(66.1653807723632,249.591391326746,24.2240075505256)) ;
#116374=CARTESIAN_POINT('Ctrl Pts',(66.0880601352411,249.908209741321,22.418631049914)) ;
#116375=CARTESIAN_POINT('Ctrl Pts',(66.0107394981189,248.595977468631,21.1388667172755)) ;
#116376=CARTESIAN_POINT('Ctrl Pts',(65.9334188609967,246.799104993584,21.5008037614803)) ;
#116377=CARTESIAN_POINT('Ctrl Pts',(65.8560982238745,246.08465738119,23.1887954388525)) ;
#116378=CARTESIAN_POINT('Ctrl Pts',(65.7787775867523,247.075710738501,24.7307307606792)) ;
#116379=CARTESIAN_POINT('Ctrl Pts',(65.7014569496302,248.907958894332,24.7818757604367)) ;
#116380=CARTESIAN_POINT('Ctrl Pts',(65.624136312508,249.983485589529,23.2976275963811)) ;
#116381=CARTESIAN_POINT('Ctrl Pts',(65.5468156753858,249.364312603574,21.5724078914629)) ;
#116382=CARTESIAN_POINT('Ctrl Pts',(65.4694950382637,247.590432115134,21.110799958047)) ;
#116383=CARTESIAN_POINT('Ctrl Pts',(65.3921744011415,246.208844628384,22.3153626902822)) ;
#116384=CARTESIAN_POINT('Ctrl Pts',(65.3148537640193,246.424474655136,24.1356155401664)) ;
#116385=CARTESIAN_POINT('Ctrl Pts',(65.2375331268972,248.049201714516,24.9840401004258)) ;
#116386=CARTESIAN_POINT('Ctrl Pts',(65.1602124897749,249.66623819922,24.1208496573188)) ;
#116387=CARTESIAN_POINT('Ctrl Pts',(65.0828918526528,249.865034670162,22.2985411464835)) ;
#116388=CARTESIAN_POINT('Ctrl Pts',(65.0055712155306,248.472935133376,21.1069666916277)) ;
#116389=CARTESIAN_POINT('Ctrl Pts',(64.9282505784084,246.702513605101,21.5838319205941)) ;
#116390=CARTESIAN_POINT('Ctrl Pts',(64.8509299412862,246.10126524972,23.3159150661253)) ;
#116391=CARTESIAN_POINT('Ctrl Pts',(64.7993828498715,246.824872768656,24.294965867468)) ;
#116392=CARTESIAN_POINT('Ctrl Pts',(64.7736093041641,247.313606204779,24.5303161002225)) ;
#116393=CARTESIAN_POINT('Origin',(57.9402651077866,248.040265107786,23.0213203435596)) ;
#116394=CARTESIAN_POINT('Ctrl Pts',(57.9402651077866,248.936544011729,24.7683224547055)) ;
#116395=CARTESIAN_POINT('Ctrl Pts',(57.9402651077867,248.969834251372,24.748365352915)) ;
#116396=CARTESIAN_POINT('Ctrl Pts',(57.9402651077867,249.002451928547,24.7273685302422)) ;
#116397=CARTESIAN_POINT('Ctrl Pts',(57.9402651077867,249.034342381865,24.7053298307907)) ;
#116398=CARTESIAN_POINT('Ctrl Pts',(57.9402651077867,249.093869423035,24.664192172554)) ;
#116399=CARTESIAN_POINT('Ctrl Pts',(57.9402651077867,249.150864283323,24.6194251339319)) ;
#116400=CARTESIAN_POINT('Ctrl Pts',(57.9402651077866,249.205168560284,24.571368724925)) ;
#116401=CARTESIAN_POINT('Ctrl Pts',(57.9402651077866,249.222893676953,24.5556829354442)) ;
#116402=CARTESIAN_POINT('Ctrl Pts',(57.9402651077868,249.240331820689,24.5396464364662)) ;
#116403=CARTESIAN_POINT('Ctrl Pts',(57.9402651077867,249.257476513462,24.5232703805546)) ;
#116404=CARTESIAN_POINT('Ctrl Pts',(57.9402651077866,249.270127083224,24.51118696556)) ;
#116405=CARTESIAN_POINT('Ctrl Pts',(57.9402651077866,249.282617872539,24.4989186712449)) ;
#116406=CARTESIAN_POINT('Ctrl Pts',(57.9402651077866,249.294946099205,24.4864698925067)) ;
#116407=CARTESIAN_POINT('Ctrl Pts',(57.9402651077866,249.305879409717,24.4754296701666)) ;
#116408=CARTESIAN_POINT('Ctrl Pts',(57.9402651077865,249.31667896791,24.4642533778532)) ;
#116409=CARTESIAN_POINT('Ctrl Pts',(57.9402651077865,249.327339178069,24.4529489071045)) ;
#116410=CARTESIAN_POINT('Ctrl Pts',(57.9402651077867,249.377034801787,24.400249878074)) ;
#116411=CARTESIAN_POINT('Ctrl Pts',(57.9402651077866,249.423735093708,24.3447378984001)) ;
#116412=CARTESIAN_POINT('Ctrl Pts',(57.9402651077866,249.467281735283,24.2867546595153)) ;
#116413=CARTESIAN_POINT('Ctrl Pts',(57.9402651077866,249.499219736011,24.2442285620089)) ;
#116414=CARTESIAN_POINT('Ctrl Pts',(57.9402651077867,249.529460550065,24.2003723299463)) ;
#116415=CARTESIAN_POINT('Ctrl Pts',(57.9402651077867,249.557925674325,24.155313058082)) ;
#116416=CARTESIAN_POINT('Ctrl Pts',(57.9402651077868,249.569913244849,24.1363371634292)) ;
#116417=CARTESIAN_POINT('Ctrl Pts',(57.9402651077868,249.581585718254,24.1171478514142)) ;
#116418=CARTESIAN_POINT('Ctrl Pts',(57.9402651077866,249.592936441842,24.0977544311853)) ;
#116419=CARTESIAN_POINT('Ctrl Pts',(57.9402651077866,249.599573895685,24.0864139267119)) ;
#116420=CARTESIAN_POINT('Ctrl Pts',(57.9402651077867,249.606102094572,24.0750020847712)) ;
#116421=CARTESIAN_POINT('Ctrl Pts',(57.9402651077867,249.612511676398,24.0635354567494)) ;
#116422=CARTESIAN_POINT('Ctrl Pts',(57.9402651077865,249.647369793866,24.0011749038419)) ;
#116423=CARTESIAN_POINT('Ctrl Pts',(57.9402651077865,249.678777831925,23.9371051763225)) ;
#116424=CARTESIAN_POINT('Ctrl Pts',(57.9402651077865,249.706585851766,23.8716486500327)) ;
#116425=CARTESIAN_POINT('Ctrl Pts',(57.9402651077865,249.733893355817,23.8073702739726)) ;
#116426=CARTESIAN_POINT('Ctrl Pts',(57.9402651077864,249.757729494085,23.7417535820802)) ;
#116427=CARTESIAN_POINT('Ctrl Pts',(57.9402651077865,249.777904928993,23.6750907110336)) ;
#116428=CARTESIAN_POINT('Ctrl Pts',(57.9402651077865,249.792011167119,23.6284814390459)) ;
#116429=CARTESIAN_POINT('Ctrl Pts',(57.9402651077868,249.804326895486,23.5813604604367)) ;
#116430=CARTESIAN_POINT('Ctrl Pts',(57.9402651077866,249.81477232718,23.5338274809802)) ;
#116431=CARTESIAN_POINT('Ctrl Pts',(57.9402651077865,249.823437278949,23.4943967531299)) ;
#116432=CARTESIAN_POINT('Ctrl Pts',(57.9402651077867,249.830814990046,23.4546824717317)) ;
#116433=CARTESIAN_POINT('Ctrl Pts',(57.9402651077865,249.836852913976,23.414742758069)) ;
#116434=CARTESIAN_POINT('Ctrl Pts',(57.9402651077864,249.838603276049,23.4031644472442)) ;
#116435=CARTESIAN_POINT('Ctrl Pts',(57.9402651077868,249.840240928434,23.3915670359813)) ;
#116436=CARTESIAN_POINT('Ctrl Pts',(57.9402651077868,249.841762838499,23.379966701035)) ;
#116437=CARTESIAN_POINT('Ctrl Pts',(57.9402651077867,249.850592372617,23.3126660401371)) ;
#116438=CARTESIAN_POINT('Ctrl Pts',(57.9402651077866,249.855549682227,23.2451444439586)) ;
#116439=CARTESIAN_POINT('Ctrl Pts',(57.9402651077867,249.85646379212,23.1776764759888)) ;
#116440=CARTESIAN_POINT('Ctrl Pts',(57.9402651077867,249.856814189209,23.1518146187315)) ;
#116441=CARTESIAN_POINT('Ctrl Pts',(57.9402651077864,249.856569965134,23.1259606312009)) ;
#116442=CARTESIAN_POINT('Ctrl Pts',(57.9402651077865,249.855719437616,23.10013009651)) ;
#116443=CARTESIAN_POINT('Ctrl Pts',(57.9402651077868,249.853467922705,23.0317515516244)) ;
#116444=CARTESIAN_POINT('Ctrl Pts',(57.9402651077864,249.846971114348,22.9635360782984)) ;
#116445=CARTESIAN_POINT('Ctrl Pts',(57.9402651077865,249.836406722431,22.8957887401495)) ;
#116446=CARTESIAN_POINT('Ctrl Pts',(57.9402651077865,249.831283115032,22.8629320678713)) ;
#116447=CARTESIAN_POINT('Ctrl Pts',(57.9402651077866,249.825202010033,22.8301857600486)) ;
#116448=CARTESIAN_POINT('Ctrl Pts',(57.9402651077866,249.81817979325,22.797586544371)) ;
#116449=CARTESIAN_POINT('Ctrl Pts',(57.9402651077866,249.814099592292,22.7786450398378)) ;
#116450=CARTESIAN_POINT('Ctrl Pts',(57.9402651077866,249.809701618464,22.7597532225742)) ;
#116451=CARTESIAN_POINT('Ctrl Pts',(57.9402651077866,249.804988737036,22.7409185608578)) ;
#116452=CARTESIAN_POINT('Ctrl Pts',(57.9402651077867,249.802096108424,22.7293583970392)) ;
#116453=CARTESIAN_POINT('Ctrl Pts',(57.9402651077864,249.799084386936,22.7178180905904)) ;
#116454=CARTESIAN_POINT('Ctrl Pts',(57.9402651077865,249.795955629747,22.7063046865931)) ;
#116455=CARTESIAN_POINT('Ctrl Pts',(57.9402651077866,249.778217509192,22.6410307980329)) ;
#116456=CARTESIAN_POINT('Ctrl Pts',(57.9402651077866,249.75679097115,22.5768702168924)) ;
#116457=CARTESIAN_POINT('Ctrl Pts',(57.9402651077866,249.731879665945,22.5141040056564)) ;
#116458=CARTESIAN_POINT('Ctrl Pts',(57.9402651077866,249.706868342887,22.4510857906947)) ;
#116459=CARTESIAN_POINT('Ctrl Pts',(57.9402651077866,249.678343600578,22.3894722456789)) ;
#116460=CARTESIAN_POINT('Ctrl Pts',(57.9402651077867,249.646464982076,22.3295717693722)) ;
#116461=CARTESIAN_POINT('Ctrl Pts',(57.9402651077868,249.615056130998,22.2705539941925)) ;
#116462=CARTESIAN_POINT('Ctrl Pts',(57.9402651077867,249.580390846709,22.2131984103696)) ;
#116463=CARTESIAN_POINT('Ctrl Pts',(57.9402651077866,249.54258637471,22.1578355096128)) ;
#116464=CARTESIAN_POINT('Ctrl Pts',(57.9402651077866,249.533519373627,22.1445573058834)) ;
#116465=CARTESIAN_POINT('Ctrl Pts',(57.9402651077865,249.524271660954,22.1313939187497)) ;
#116466=CARTESIAN_POINT('Ctrl Pts',(57.9402651077865,249.514844610744,22.1183502921032)) ;
#116467=CARTESIAN_POINT('Ctrl Pts',(57.9402651077866,249.505448906097,22.1053500363732)) ;
#116468=CARTESIAN_POINT('Ctrl Pts',(57.9402651077865,249.495871453199,22.0924642624107)) ;
#116469=CARTESIAN_POINT('Ctrl Pts',(57.9402651077865,249.486133728681,22.0797237707493)) ;
#116470=CARTESIAN_POINT('Ctrl Pts',(57.9402651077865,249.446013857083,22.027232360806)) ;
#116471=CARTESIAN_POINT('Ctrl Pts',(57.9402651077865,249.403126873497,21.9771313880535)) ;
#116472=CARTESIAN_POINT('Ctrl Pts',(57.9402651077866,249.357623594114,21.929703658124)) ;
#116473=CARTESIAN_POINT('Ctrl Pts',(57.9402651077867,249.312871487116,21.8830588695883)) ;
#116474=CARTESIAN_POINT('Ctrl Pts',(57.9402651077866,249.265588098698,21.8389991407756)) ;
#116475=CARTESIAN_POINT('Ctrl Pts',(57.9402651077866,249.215886432752,21.7978329278902)) ;
#116476=CARTESIAN_POINT('Ctrl Pts',(57.9402651077865,249.167850788198,21.7580466243097)) ;
#116477=CARTESIAN_POINT('Ctrl Pts',(57.9402651077866,249.117555685649,21.7209627068944)) ;
#116478=CARTESIAN_POINT('Ctrl Pts',(57.9402651077865,249.065083510332,21.6869041375018)) ;
#116479=CARTESIAN_POINT('Ctrl Pts',(57.9402651077864,249.048474840792,21.6761238044844)) ;
#116480=CARTESIAN_POINT('Ctrl Pts',(57.9402651077865,249.031647939631,21.6656469393582)) ;
#116481=CARTESIAN_POINT('Ctrl Pts',(57.9402651077866,249.01460512908,21.6554848536836)) ;
#116482=CARTESIAN_POINT('',(57.9394803992446,247.064599950825,21.6547731742408)) ;
#116483=CARTESIAN_POINT('Ctrl Pts',(57.9402651077867,247.09020061484,21.6384890010805)) ;
#116484=CARTESIAN_POINT('Ctrl Pts',(57.9400035382726,247.081876264352,21.6442081872039)) ;
#116485=CARTESIAN_POINT('Ctrl Pts',(57.9397419687586,247.073603557709,21.6500025415884)) ;
#116486=CARTESIAN_POINT('Ctrl Pts',(57.9394803992446,247.065383843876,21.6558711193933)) ;
#116487=CARTESIAN_POINT('Ctrl Pts',(57.9402651077866,247.063751382118,21.653699040999)) ;
#116488=CARTESIAN_POINT('Ctrl Pts',(57.9402651077865,247.022795562072,21.6777771701807)) ;
#116489=CARTESIAN_POINT('Ctrl Pts',(57.9402651077866,246.983015097768,21.7036389402643)) ;
#116490=CARTESIAN_POINT('Ctrl Pts',(57.9402651077865,246.944545251137,21.731258981544)) ;
#116491=CARTESIAN_POINT('Ctrl Pts',(57.9402651077865,246.893065219322,21.7682198932282)) ;
#116492=CARTESIAN_POINT('Ctrl Pts',(57.9402651077865,246.843930666271,21.8083275360126)) ;
#116493=CARTESIAN_POINT('Ctrl Pts',(57.9402651077865,246.79721860728,21.8512529472481)) ;
#116494=CARTESIAN_POINT('Ctrl Pts',(57.9402651077865,246.778270710595,21.8686648591795)) ;
#116495=CARTESIAN_POINT('Ctrl Pts',(57.9402651077864,246.759721683068,21.8865409338896)) ;
#116496=CARTESIAN_POINT('Ctrl Pts',(57.9402651077865,246.741577912132,21.9048612357463)) ;
#116497=CARTESIAN_POINT('Ctrl Pts',(57.9402651077866,246.732151157705,21.9143797083529)) ;
#116498=CARTESIAN_POINT('Ctrl Pts',(57.9402651077865,246.722832136955,21.9240198964915)) ;
#116499=CARTESIAN_POINT('Ctrl Pts',(57.9402651077865,246.713627348976,21.933773241702)) ;
#116500=CARTESIAN_POINT('Ctrl Pts',(57.9402651077864,246.668538281455,21.9815493818791)) ;
#116501=CARTESIAN_POINT('Ctrl Pts',(57.9402651077864,246.626266996622,22.0319509032703)) ;
#116502=CARTESIAN_POINT('Ctrl Pts',(57.9402651077864,246.586892797857,22.084618239577)) ;
#116503=CARTESIAN_POINT('Ctrl Pts',(57.9402651077864,246.55575619811,22.1262668780695)) ;
#116504=CARTESIAN_POINT('Ctrl Pts',(57.9402651077867,246.52643165571,22.1693336238241)) ;
#116505=CARTESIAN_POINT('Ctrl Pts',(57.9402651077865,246.498971999877,22.2136592363338)) ;
#116506=CARTESIAN_POINT('Ctrl Pts',(57.9402651077864,246.484061222999,22.2377283405538)) ;
#116507=CARTESIAN_POINT('Ctrl Pts',(57.9402651077866,246.469700544209,22.2621688855007)) ;
#116508=CARTESIAN_POINT('Ctrl Pts',(57.9402651077866,246.455900172974,22.2869569486825)) ;
#116509=CARTESIAN_POINT('Ctrl Pts',(57.9402651077867,246.449901218829,22.2977321989879)) ;
#116510=CARTESIAN_POINT('Ctrl Pts',(57.9402651077867,246.444008646131,22.3085724311742)) ;
#116511=CARTESIAN_POINT('Ctrl Pts',(57.9402651077866,246.438229248595,22.3194639887581)) ;
#116512=CARTESIAN_POINT('Ctrl Pts',(57.9402651077865,246.406422480815,22.3794053997209)) ;
#116513=CARTESIAN_POINT('Ctrl Pts',(57.9402651077865,246.377989861048,22.4409885827609)) ;
#116514=CARTESIAN_POINT('Ctrl Pts',(57.9402651077866,246.353019437315,22.5038540656447)) ;
#116515=CARTESIAN_POINT('Ctrl Pts',(57.9402651077866,246.327688728189,22.5676266022309)) ;
#116516=CARTESIAN_POINT('Ctrl Pts',(57.9402651077867,246.305920219198,22.6327195891187)) ;
#116517=CARTESIAN_POINT('Ctrl Pts',(57.9402651077866,246.287845359425,22.6987929595691)) ;
#116518=CARTESIAN_POINT('Ctrl Pts',(57.9402651077865,246.275494931828,22.7439404399967)) ;
#116519=CARTESIAN_POINT('Ctrl Pts',(57.9402651077865,246.264869853737,22.7895463862758)) ;
#116520=CARTESIAN_POINT('Ctrl Pts',(57.9402651077865,246.256024758883,22.8355082400426)) ;
#116521=CARTESIAN_POINT('Ctrl Pts',(57.9402651077865,246.251600756467,22.8584967275025)) ;
#116522=CARTESIAN_POINT('Ctrl Pts',(57.9402651077866,246.247622214495,22.881574306955)) ;
#116523=CARTESIAN_POINT('Ctrl Pts',(57.9402651077866,246.2440970561,22.9047283899068)) ;
#116524=CARTESIAN_POINT('Ctrl Pts',(57.9402651077865,246.241835333762,22.9195839228383)) ;
#116525=CARTESIAN_POINT('Ctrl Pts',(57.9402651077866,246.239760258836,22.9344709506001)) ;
#116526=CARTESIAN_POINT('Ctrl Pts',(57.9402651077865,246.237874091866,22.9493861652913)) ;
#116527=CARTESIAN_POINT('Ctrl Pts',(57.9402651077864,246.236484466093,22.9603748884925)) ;
#116528=CARTESIAN_POINT('Ctrl Pts',(57.9402651077865,246.235198549517,22.9713697420018)) ;
#116529=CARTESIAN_POINT('Ctrl Pts',(57.9402651077865,246.23401688886,22.9823680560691)) ;
#116530=CARTESIAN_POINT('Ctrl Pts',(57.9402651077867,246.226554706152,23.0518223690129)) ;
#116531=CARTESIAN_POINT('Ctrl Pts',(57.9402651077868,246.223244400811,23.1214287161277)) ;
#116532=CARTESIAN_POINT('Ctrl Pts',(57.9402651077866,246.224210769353,23.1908364633901)) ;
#116533=CARTESIAN_POINT('Ctrl Pts',(57.9402651077865,246.224503387308,23.2118532413484)) ;
#116534=CARTESIAN_POINT('Ctrl Pts',(57.9402651077866,246.225188455189,23.2328519633107)) ;
#116535=CARTESIAN_POINT('Ctrl Pts',(57.9402651077867,246.226270324961,23.2538232262009)) ;
#116536=CARTESIAN_POINT('Ctrl Pts',(57.9402651077868,246.229736559053,23.3210136665446)) ;
#116537=CARTESIAN_POINT('Ctrl Pts',(57.9402651077866,246.237271980017,23.3879220396537)) ;
#116538=CARTESIAN_POINT('Ctrl Pts',(57.9402651077866,246.248654075727,23.4543056841415)) ;
#116539=CARTESIAN_POINT('Ctrl Pts',(57.9402651077867,246.254586354754,23.4889044357236)) ;
#116540=CARTESIAN_POINT('Ctrl Pts',(57.9402651077866,246.261564434129,23.523360710123)) ;
#116541=CARTESIAN_POINT('Ctrl Pts',(57.9402651077867,246.26956226066,23.55763995277)) ;
#116542=CARTESIAN_POINT('Ctrl Pts',(57.9402651077867,246.273897374718,23.5762205541502)) ;
#116543=CARTESIAN_POINT('Ctrl Pts',(57.9402651077867,246.278532156485,23.5947491358563)) ;
#116544=CARTESIAN_POINT('Ctrl Pts',(57.9402651077867,246.283462886363,23.6132201155199)) ;
#116545=CARTESIAN_POINT('Ctrl Pts',(57.9402651077867,246.28644344509,23.624385569922)) ;
#116546=CARTESIAN_POINT('Ctrl Pts',(57.9402651077865,246.289532150096,23.635529975047)) ;
#116547=CARTESIAN_POINT('Ctrl Pts',(57.9402651077865,246.292728231333,23.646652083647)) ;
#116548=CARTESIAN_POINT('Ctrl Pts',(57.9402651077865,246.296265107811,23.6589601325905)) ;
#116549=CARTESIAN_POINT('Ctrl Pts',(57.9402651077868,246.299931179453,23.6712327041133)) ;
#116550=CARTESIAN_POINT('Ctrl Pts',(57.9402651077867,246.303722785304,23.6834617388722)) ;
#116551=CARTESIAN_POINT('Ctrl Pts',(57.9402651077865,246.324579729698,23.7507314678489)) ;
#116552=CARTESIAN_POINT('Ctrl Pts',(57.9402651077866,246.349248273941,23.8167452634601)) ;
#116553=CARTESIAN_POINT('Ctrl Pts',(57.9402651077866,246.377460807139,23.8812387823142)) ;
#116554=CARTESIAN_POINT('Ctrl Pts',(57.9402651077866,246.405673340336,23.9457323011682)) ;
#116555=CARTESIAN_POINT('Ctrl Pts',(57.9402651077867,246.437430309462,24.0087064048567)) ;
#116556=CARTESIAN_POINT('Ctrl Pts',(57.9402651077866,246.47251718865,24.0698922633336)) ;
#116557=CARTESIAN_POINT('Ctrl Pts',(57.9402651077865,246.508042580594,24.1318428173341)) ;
#116558=CARTESIAN_POINT('Ctrl Pts',(57.9402651077865,246.546981996077,24.1919611082941)) ;
#116559=CARTESIAN_POINT('Ctrl Pts',(57.9402651077866,246.589161244989,24.2499497148609)) ;
#116560=CARTESIAN_POINT('Ctrl Pts',(57.9402651077866,246.598810156939,24.2632151705834)) ;
#116561=CARTESIAN_POINT('Ctrl Pts',(57.9402651077865,246.608628797714,24.2763690679559)) ;
#116562=CARTESIAN_POINT('Ctrl Pts',(57.9402651077864,246.618615401402,24.289407630059)) ;
#116563=CARTESIAN_POINT('Ctrl Pts',(57.9402651077864,246.625695864494,24.2986519197716)) ;
#116564=CARTESIAN_POINT('Ctrl Pts',(57.9402651077866,246.632860426978,24.3078376671516)) ;
#116565=CARTESIAN_POINT('Ctrl Pts',(57.9402651077866,246.64009999969,24.3169532337087)) ;
#116566=CARTESIAN_POINT('Ctrl Pts',(57.9402651077866,246.685677256768,24.3743409466196)) ;
#116567=CARTESIAN_POINT('Ctrl Pts',(57.9402651077865,246.73430598704,24.4290572965446)) ;
#116568=CARTESIAN_POINT('Ctrl Pts',(57.9402651077865,246.78574661108,24.4808204424783)) ;
#116569=CARTESIAN_POINT('Ctrl Pts',(57.9402651077865,246.837101404366,24.5324972195167)) ;
#116570=CARTESIAN_POINT('Ctrl Pts',(57.9402651077867,246.891259241171,24.5812315797706)) ;
#116571=CARTESIAN_POINT('Ctrl Pts',(57.9402651077866,246.948028081008,24.6267202960962)) ;
#116572=CARTESIAN_POINT('Ctrl Pts',(57.9402651077866,247.003352437633,24.6710515519693)) ;
#116573=CARTESIAN_POINT('Ctrl Pts',(57.9402651077867,247.061157230315,24.7123009754626)) ;
#116574=CARTESIAN_POINT('Ctrl Pts',(57.9402651077866,247.121300105744,24.7501540607501)) ;
#116575=CARTESIAN_POINT('Ctrl Pts',(57.9402651077866,247.143343628465,24.7640279458888)) ;
#116576=CARTESIAN_POINT('Ctrl Pts',(57.9402651077865,247.16570154556,24.7774451902113)) ;
#116577=CARTESIAN_POINT('Ctrl Pts',(57.9402651077866,247.188367839728,24.7903888257488)) ;
#116578=CARTESIAN_POINT('Ctrl Pts',(61.1070133762705,248.766854525377,24.5301718052866)) ;
#116579=CARTESIAN_POINT('Ctrl Pts',(61.080638560942,249.266941772283,24.2893541299283)) ;
#116580=CARTESIAN_POINT('Ctrl Pts',(61.027888930285,249.999896115323,23.2741377447068)) ;
#116581=CARTESIAN_POINT('Ctrl Pts',(60.9487644842995,249.321107628342,21.5135065273509)) ;
#116582=CARTESIAN_POINT('Ctrl Pts',(60.869640038314,247.474294984015,21.1268386661821)) ;
#116583=CARTESIAN_POINT('Ctrl Pts',(60.7905155923284,246.143541845113,22.4625909175899)) ;
#116584=CARTESIAN_POINT('Ctrl Pts',(60.7113911463429,246.537942674782,24.3072111397376)) ;
#116585=CARTESIAN_POINT('Ctrl Pts',(60.6322667003574,248.299453084171,24.9816336600195)) ;
#116586=CARTESIAN_POINT('Ctrl Pts',(60.5531422543719,249.825029443136,23.8726149962676)) ;
#116587=CARTESIAN_POINT('Ctrl Pts',(60.4740178083863,249.726823714205,21.9890071491867)) ;
#116588=CARTESIAN_POINT('Ctrl Pts',(60.3948933624008,248.094107651175,21.0446559799089)) ;
#116589=CARTESIAN_POINT('Ctrl Pts',(60.3157689164153,246.412415556467,21.8987259886766)) ;
#116590=CARTESIAN_POINT('Ctrl Pts',(60.2366444704298,246.211787909224,23.7741738257661)) ;
#116591=CARTESIAN_POINT('Ctrl Pts',(60.1575200244442,247.674770120869,24.9646488533224)) ;
#116592=CARTESIAN_POINT('Ctrl Pts',(60.0783955784587,249.470290254645,24.3870222847478)) ;
#116593=CARTESIAN_POINT('Ctrl Pts',(59.9992711324732,249.964728074474,22.5668356392193)) ;
#116594=CARTESIAN_POINT('Ctrl Pts',(59.9201466864877,248.708227359668,21.1601540415291)) ;
#116595=CARTESIAN_POINT('Ctrl Pts',(59.8410222405021,246.843993229004,21.4468212689482)) ;
#116596=CARTESIAN_POINT('Ctrl Pts',(59.7618977945166,246.068165661642,23.1660184318367)) ;
#116597=CARTESIAN_POINT('Ctrl Pts',(59.6827733485311,247.086617602811,24.7535645967704)) ;
#116598=CARTESIAN_POINT('Ctrl Pts',(59.6036489025456,248.972728693476,24.765059256107)) ;
#116599=CARTESIAN_POINT('Ctrl Pts',(59.5245244565601,250.01045443974,23.1900441840451)) ;
#116600=CARTESIAN_POINT('Ctrl Pts',(59.4454000105745,249.255638581674,21.4615187367073)) ;
#116601=CARTESIAN_POINT('Ctrl Pts',(59.366275564589,247.395036866021,21.1521509471284)) ;
#116602=CARTESIAN_POINT('Ctrl Pts',(59.2871511186035,246.121484539962,22.5434135589518)) ;
#116603=CARTESIAN_POINT('Ctrl Pts',(59.2080266726179,246.593700488024,24.3694911579488)) ;
#116604=CARTESIAN_POINT('Ctrl Pts',(59.1289022266325,248.382047392536,24.9689595410457)) ;
#116605=CARTESIAN_POINT('Ctrl Pts',(59.0497777806469,249.859429881076,23.7964032967042)) ;
#116606=CARTESIAN_POINT('Ctrl Pts',(58.9706533346614,249.681677563272,21.9186513706623)) ;
#116607=CARTESIAN_POINT('Ctrl Pts',(58.8915288886758,248.010515861749,21.0441437544105)) ;
#116608=CARTESIAN_POINT('Ctrl Pts',(58.8124044426904,246.366420027326,21.9685336234909)) ;
#116609=CARTESIAN_POINT('Ctrl Pts',(58.7332799967048,246.245244316357,23.8507855964087)) ;
#116610=CARTESIAN_POINT('Ctrl Pts',(58.6541555507193,247.757231817376,24.9783571808533)) ;
#116611=CARTESIAN_POINT('Ctrl Pts',(58.5750311047338,249.52674160729,24.3253671527601)) ;
#116612=CARTESIAN_POINT('Ctrl Pts',(58.4959066587482,249.943786803312,22.4858845648418)) ;
#116613=CARTESIAN_POINT('Ctrl Pts',(58.4167822127627,248.628990691216,21.1336209784045)) ;
#116614=CARTESIAN_POINT('Ctrl Pts',(58.3376577667772,246.778457851123,21.4987139336705)) ;
#116615=CARTESIAN_POINT('Ctrl Pts',(58.2585333207917,246.076159531858,23.2494146074457)) ;
#116616=CARTESIAN_POINT('Ctrl Pts',(58.1794088748061,247.160417795382,24.7919845448622)) ;
#116617=CARTESIAN_POINT('Ctrl Pts',(58.1002844288207,249.04608391346,24.7249601520188)) ;
#116618=CARTESIAN_POINT('Ctrl Pts',(58.0211505904172,250.014463203649,23.1051876352719)) ;
#116619=CARTESIAN_POINT('Ctrl Pts',(57.9683915673424,249.46448777725,21.9799214227029)) ;
#116620=CARTESIAN_POINT('Ctrl Pts',(57.9420073595959,249.012341492745,21.6576369534145)) ;
#116621=CARTESIAN_POINT('Ctrl Pts',(61.0509160513592,248.809010496563,24.6177138162294)) ;
#116622=CARTESIAN_POINT('Ctrl Pts',(61.0245412360307,249.338112291522,24.3629241468703)) ;
#116623=CARTESIAN_POINT('Ctrl Pts',(60.9717916053737,250.113591892182,23.2888059504641)) ;
#116624=CARTESIAN_POINT('Ctrl Pts',(60.8926671593882,249.395420794876,21.4260247195345)) ;
#116625=CARTESIAN_POINT('Ctrl Pts',(60.8135427134026,247.441457979165,21.0169227864956)) ;
#116626=CARTESIAN_POINT('Ctrl Pts',(60.7344182674171,246.033495910951,22.4301740105829)) ;
#116627=CARTESIAN_POINT('Ctrl Pts',(60.6552938214316,246.450779471375,24.3818172020345)) ;
#116628=CARTESIAN_POINT('Ctrl Pts',(60.5761693754461,248.314490904155,25.0953690237408)) ;
#116629=CARTESIAN_POINT('Ctrl Pts',(60.4970449294606,249.928579635412,23.9220062370182)) ;
#116630=CARTESIAN_POINT('Ctrl Pts',(60.417920483475,249.824676111027,21.9291133987079)) ;
#116631=CARTESIAN_POINT('Ctrl Pts',(60.3387960374895,248.097231540201,20.929971945236)) ;
#116632=CARTESIAN_POINT('Ctrl Pts',(60.259671591504,246.317969398677,21.8335942180601)) ;
#116633=CARTESIAN_POINT('Ctrl Pts',(60.1805471455185,246.105701541555,23.8178536109865)) ;
#116634=CARTESIAN_POINT('Ctrl Pts',(60.1014226995329,247.6535644774,25.0773987760169)) ;
#116635=CARTESIAN_POINT('Ctrl Pts',(60.0222982535474,249.55325884382,24.4662589076446)) ;
#116636=CARTESIAN_POINT('Ctrl Pts',(59.9431738075619,250.076383437751,22.5404669038136)) ;
#116637=CARTESIAN_POINT('Ctrl Pts',(59.8640493615764,248.74698184296,21.0521710856772)) ;
#116638=CARTESIAN_POINT('Ctrl Pts',(59.7849249155908,246.77458676418,21.3554704509814)) ;
#116639=CARTESIAN_POINT('Ctrl Pts',(59.7058004696053,245.95374647879,23.1744136661912)) ;
#116640=CARTESIAN_POINT('Ctrl Pts',(59.6266760236198,247.031287954775,24.8540676278617)) ;
#116641=CARTESIAN_POINT('Ctrl Pts',(59.5475515776343,249.026829272288,24.8662291955183)) ;
#116642=CARTESIAN_POINT('Ctrl Pts',(59.4684271316487,250.124762799729,23.1998333678479)) ;
#116643=CARTESIAN_POINT('Ctrl Pts',(59.3893026856632,249.326153301412,21.3710206507133)) ;
#116644=CARTESIAN_POINT('Ctrl Pts',(59.3101782396777,247.357601386628,21.0437036599653)) ;
#116645=CARTESIAN_POINT('Ctrl Pts',(59.2310537936922,246.010158863627,22.5156858985233)) ;
#116646=CARTESIAN_POINT('Ctrl Pts',(59.1519293477067,246.509772295631,24.447710642888)) ;
#116647=CARTESIAN_POINT('Ctrl Pts',(59.0728049017211,248.401877249398,25.0819595654112)) ;
#116648=CARTESIAN_POINT('Ctrl Pts',(58.9936804557356,249.964975951402,23.8413728129799)) ;
#116649=CARTESIAN_POINT('Ctrl Pts',(58.9145560097501,249.77691062682,21.8546756502285)) ;
#116650=CARTESIAN_POINT('Ctrl Pts',(58.8354315637646,248.008789841071,20.9294300009407)) ;
#116651=CARTESIAN_POINT('Ctrl Pts',(58.756307117779,246.269305256213,21.9074520200949)) ;
#116652=CARTESIAN_POINT('Ctrl Pts',(58.6771826717935,246.141099055042,23.8989103178167)) ;
#116653=CARTESIAN_POINT('Ctrl Pts',(58.598058225808,247.74081051678,25.0919024466211)) ;
#116654=CARTESIAN_POINT('Ctrl Pts',(58.5189337798225,249.612985445922,24.401026608271)) ;
#116655=CARTESIAN_POINT('Ctrl Pts',(58.4398093338369,250.054227175559,22.4548191313059)) ;
#116656=CARTESIAN_POINT('Ctrl Pts',(58.3606848878514,248.663147944448,21.0240986015019)) ;
#116657=CARTESIAN_POINT('Ctrl Pts',(58.2815604418659,246.705249091034,21.4103738747732)) ;
#116658=CARTESIAN_POINT('Ctrl Pts',(58.2024359958804,245.96220414514,23.2626484021906)) ;
#116659=CARTESIAN_POINT('Ctrl Pts',(58.1233115498949,247.109369958663,24.8947166618521)) ;
#116660=CARTESIAN_POINT('Ctrl Pts',(58.0441871039093,249.104440486738,24.8238035826266)) ;
#116661=CARTESIAN_POINT('Ctrl Pts',(57.9650532655059,250.129004148,23.1100535293344)) ;
#116662=CARTESIAN_POINT('Ctrl Pts',(57.912294242431,249.54711971265,21.9195005277123)) ;
#116663=CARTESIAN_POINT('Ctrl Pts',(57.8859100346846,249.068740365456,21.5785174447743)) ;
#116664=CARTESIAN_POINT('Ctrl Pts',(60.9948187264479,248.85116646775,24.7052558271723)) ;
#116665=CARTESIAN_POINT('Ctrl Pts',(60.9684439111194,249.409282810763,24.4364941638122)) ;
#116666=CARTESIAN_POINT('Ctrl Pts',(60.9156942804624,250.227287669041,23.3034741562214)) ;
#116667=CARTESIAN_POINT('Ctrl Pts',(60.8365698344769,249.46973396141,21.338542911718)) ;
#116668=CARTESIAN_POINT('Ctrl Pts',(60.7574453884913,247.408620974313,20.9070069068091)) ;
#116669=CARTESIAN_POINT('Ctrl Pts',(60.6783209425058,245.92344997679,22.3977571035757)) ;
#116670=CARTESIAN_POINT('Ctrl Pts',(60.5991964965203,246.363616267967,24.4564232643313)) ;
#116671=CARTESIAN_POINT('Ctrl Pts',(60.5200720505348,248.32952872414,25.209104387462)) ;
#116672=CARTESIAN_POINT('Ctrl Pts',(60.4409476045492,250.032129827686,23.9713974777687)) ;
#116673=CARTESIAN_POINT('Ctrl Pts',(60.3618231585637,249.92252850785,21.869219648229)) ;
#116674=CARTESIAN_POINT('Ctrl Pts',(60.2826987125782,248.100355429226,20.815287910563)) ;
#116675=CARTESIAN_POINT('Ctrl Pts',(60.2035742665927,246.223523240888,21.7684624474437)) ;
#116676=CARTESIAN_POINT('Ctrl Pts',(60.1244498206071,245.999615173888,23.8615333962069)) ;
#116677=CARTESIAN_POINT('Ctrl Pts',(60.0453253746216,247.632358833932,25.1901486987114)) ;
#116678=CARTESIAN_POINT('Ctrl Pts',(59.966200928636,249.636227432995,24.5454955305414)) ;
#116679=CARTESIAN_POINT('Ctrl Pts',(59.8870764826506,250.188038801027,22.514098168408)) ;
#116680=CARTESIAN_POINT('Ctrl Pts',(59.807952036665,248.785736326251,20.9441881298252)) ;
#116681=CARTESIAN_POINT('Ctrl Pts',(59.7288275906795,246.705180299356,21.2641196330146)) ;
#116682=CARTESIAN_POINT('Ctrl Pts',(59.649703144694,245.839327295939,23.1828089005457)) ;
#116683=CARTESIAN_POINT('Ctrl Pts',(59.5705786987085,246.975958306739,24.9545706589532)) ;
#116684=CARTESIAN_POINT('Ctrl Pts',(59.4914542527229,249.0809298511,24.9673991349296)) ;
#116685=CARTESIAN_POINT('Ctrl Pts',(59.4123298067374,250.239071159718,23.2096225516508)) ;
#116686=CARTESIAN_POINT('Ctrl Pts',(59.3332053607519,249.39666802115,21.2805225647191)) ;
#116687=CARTESIAN_POINT('Ctrl Pts',(59.2540809147664,247.320165907236,20.9352563728022)) ;
#116688=CARTESIAN_POINT('Ctrl Pts',(59.1749564687808,245.898833187292,22.4879582380948)) ;
#116689=CARTESIAN_POINT('Ctrl Pts',(59.0958320227954,246.425844103238,24.5259301278273)) ;
#116690=CARTESIAN_POINT('Ctrl Pts',(59.0167075768098,248.421707106259,25.1949595897767)) ;
#116691=CARTESIAN_POINT('Ctrl Pts',(58.9375831308243,250.070522021727,23.8863423292556)) ;
#116692=CARTESIAN_POINT('Ctrl Pts',(58.8584586848388,249.872143690368,21.7906999297945)) ;
#116693=CARTESIAN_POINT('Ctrl Pts',(58.7793342388532,248.007063820394,20.8147162474708)) ;
#116694=CARTESIAN_POINT('Ctrl Pts',(58.7002097928677,246.172190485098,21.8463704166988)) ;
#116695=CARTESIAN_POINT('Ctrl Pts',(58.6210853468822,246.036953793729,23.9470350392246)) ;
#116696=CARTESIAN_POINT('Ctrl Pts',(58.5419609008967,247.724389216186,25.2054477123889)) ;
#116697=CARTESIAN_POINT('Ctrl Pts',(58.4628364549111,249.699229284554,24.4766860637818)) ;
#116698=CARTESIAN_POINT('Ctrl Pts',(58.3837120089257,250.164667547808,22.4237536977701)) ;
#116699=CARTESIAN_POINT('Ctrl Pts',(58.3045875629401,248.697305197679,20.9145762245993)) ;
#116700=CARTESIAN_POINT('Ctrl Pts',(58.2254631169546,246.632040330946,21.322033815876)) ;
#116701=CARTESIAN_POINT('Ctrl Pts',(58.1463386709691,245.848248758422,23.2758821969355)) ;
#116702=CARTESIAN_POINT('Ctrl Pts',(58.0672142249835,247.058322121945,24.997448778842)) ;
#116703=CARTESIAN_POINT('Ctrl Pts',(57.988089778998,249.162797060017,24.9226470132344)) ;
#116704=CARTESIAN_POINT('Ctrl Pts',(57.9089559405946,250.243545092351,23.1149194233968)) ;
#116705=CARTESIAN_POINT('Ctrl Pts',(57.8561969175197,249.629751648052,21.8590796327216)) ;
#116706=CARTESIAN_POINT('Ctrl Pts',(57.8298127097733,249.125139238166,21.4993979361343)) ;
#116707=CARTESIAN_POINT('Ctrl Pts',(60.9387214015366,248.893322438937,24.7927978381151)) ;
#116708=CARTESIAN_POINT('Ctrl Pts',(60.9123465862081,249.480453330002,24.5100641807542)) ;
#116709=CARTESIAN_POINT('Ctrl Pts',(60.8595969555511,250.340983445901,23.3181423619787)) ;
#116710=CARTESIAN_POINT('Ctrl Pts',(60.7804725095656,249.544047127944,21.2510611039017)) ;
#116711=CARTESIAN_POINT('Ctrl Pts',(60.70134806358,247.375783969461,20.7970910271226)) ;
#116712=CARTESIAN_POINT('Ctrl Pts',(60.6222236175945,245.813404042628,22.3653401965687)) ;
#116713=CARTESIAN_POINT('Ctrl Pts',(60.543099171609,246.27645306456,24.5310293266281)) ;
#116714=CARTESIAN_POINT('Ctrl Pts',(60.4639747256235,248.344566544123,25.3228397511833)) ;
#116715=CARTESIAN_POINT('Ctrl Pts',(60.3848502796379,250.13568001996,24.0207887185192)) ;
#116716=CARTESIAN_POINT('Ctrl Pts',(60.3057258336524,250.020380904671,21.8093258977503)) ;
#116717=CARTESIAN_POINT('Ctrl Pts',(60.2266013876669,248.103479318252,20.7006038758901)) ;
#116718=CARTESIAN_POINT('Ctrl Pts',(60.1474769416814,246.129077083099,21.7033306768272)) ;
#116719=CARTESIAN_POINT('Ctrl Pts',(60.0683524956958,245.893528806219,23.9052131814272)) ;
#116720=CARTESIAN_POINT('Ctrl Pts',(59.9892280497103,247.611153190463,25.3028986214059)) ;
#116721=CARTESIAN_POINT('Ctrl Pts',(59.9101036037248,249.71919602217,24.6247321534382)) ;
#116722=CARTESIAN_POINT('Ctrl Pts',(59.8309791577393,250.299694164303,22.4877294330023)) ;
#116723=CARTESIAN_POINT('Ctrl Pts',(59.7518547117538,248.824490809544,20.8362051739732)) ;
#116724=CARTESIAN_POINT('Ctrl Pts',(59.6727302657682,246.635773834532,21.1727688150478)) ;
#116725=CARTESIAN_POINT('Ctrl Pts',(59.5936058197827,245.724908113088,23.1912041349002)) ;
#116726=CARTESIAN_POINT('Ctrl Pts',(59.5144813737972,246.920628658703,25.0550736900445)) ;
#116727=CARTESIAN_POINT('Ctrl Pts',(59.4353569278117,249.135030429914,25.068569074341)) ;
#116728=CARTESIAN_POINT('Ctrl Pts',(59.3562324818261,250.353379519707,23.2194117354537)) ;
#116729=CARTESIAN_POINT('Ctrl Pts',(59.2771080358406,249.467182740888,21.190024478725)) ;
#116730=CARTESIAN_POINT('Ctrl Pts',(59.1979835898551,247.282730427844,20.8268090856391)) ;
#116731=CARTESIAN_POINT('Ctrl Pts',(59.1188591438696,245.787507510957,22.4602305776664)) ;
#116732=CARTESIAN_POINT('Ctrl Pts',(59.0397346978841,246.341915910844,24.6041496127664)) ;
#116733=CARTESIAN_POINT('Ctrl Pts',(58.9606102518985,248.441536963121,25.3079596141421)) ;
#116734=CARTESIAN_POINT('Ctrl Pts',(58.881485805913,250.176068092052,23.9313118455313)) ;
#116735=CARTESIAN_POINT('Ctrl Pts',(58.8023613599274,249.967376753917,21.7267242093606)) ;
#116736=CARTESIAN_POINT('Ctrl Pts',(58.7232369139419,248.005337799717,20.7000024940009)) ;
#116737=CARTESIAN_POINT('Ctrl Pts',(58.6441124679564,246.075075713985,21.7852888133028)) ;
#116738=CARTESIAN_POINT('Ctrl Pts',(58.5649880219709,245.932808532414,23.9951597606326)) ;
#116739=CARTESIAN_POINT('Ctrl Pts',(58.4858635759853,247.70796791559,25.3189929781567)) ;
#116740=CARTESIAN_POINT('Ctrl Pts',(58.4067391299999,249.785473123187,24.5523455192925)) ;
#116741=CARTESIAN_POINT('Ctrl Pts',(58.3276146840143,250.275107920055,22.3926882642343)) ;
#116742=CARTESIAN_POINT('Ctrl Pts',(58.2484902380288,248.731462450911,20.8050538476968)) ;
#116743=CARTESIAN_POINT('Ctrl Pts',(58.1693657920433,246.558831570858,21.2336937569787)) ;
#116744=CARTESIAN_POINT('Ctrl Pts',(58.0902413460577,245.734293371704,23.2891159916804)) ;
#116745=CARTESIAN_POINT('Ctrl Pts',(58.0111169000722,247.007274285226,25.1001808958319)) ;
#116746=CARTESIAN_POINT('Ctrl Pts',(57.9319924540867,249.221153633296,25.0214904438423)) ;
#116747=CARTESIAN_POINT('Ctrl Pts',(57.8528586156833,250.358086036701,23.1197853174594)) ;
#116748=CARTESIAN_POINT('Ctrl Pts',(57.8000995926084,249.712383583452,21.7986587377309)) ;
#116749=CARTESIAN_POINT('Ctrl Pts',(57.773715384862,249.181538110878,21.4202784274943)) ;
#116750=CARTESIAN_POINT('Ctrl Pts',(60.9402651077866,249.016778829374,21.653698982557)) ;
#116751=CARTESIAN_POINT('Ctrl Pts',(60.9402651077866,249.057734649078,21.6777771102707)) ;
#116752=CARTESIAN_POINT('Ctrl Pts',(60.9402651077866,249.097515112934,21.7036388786869)) ;
#116753=CARTESIAN_POINT('Ctrl Pts',(60.9402651077866,249.135984959003,21.7312589180718)) ;
#116754=CARTESIAN_POINT('Ctrl Pts',(60.9402651077866,249.187464991094,21.7682198279585)) ;
#116755=CARTESIAN_POINT('Ctrl Pts',(60.9402651077866,249.236599544122,21.8083274686639)) ;
#116756=CARTESIAN_POINT('Ctrl Pts',(60.9402651077866,249.283311602843,21.8512528776645)) ;
#116757=CARTESIAN_POINT('Ctrl Pts',(60.9402651077866,249.302259501122,21.8686647902544)) ;
#116758=CARTESIAN_POINT('Ctrl Pts',(60.9402651077865,249.320808530131,21.8865408656809)) ;
#116759=CARTESIAN_POINT('Ctrl Pts',(60.9402651077866,249.338952302437,21.9048611683146)) ;
#116760=CARTESIAN_POINT('Ctrl Pts',(60.9402651077866,249.348379057922,21.9143796416741)) ;
#116761=CARTESIAN_POINT('Ctrl Pts',(60.9402651077866,249.357698079696,21.9240198305948)) ;
#116762=CARTESIAN_POINT('Ctrl Pts',(60.9402651077866,249.36690286865,21.9337731766018)) ;
#116763=CARTESIAN_POINT('Ctrl Pts',(60.9402651077866,249.411991934883,21.9815493142511)) ;
#116764=CARTESIAN_POINT('Ctrl Pts',(60.9402651077867,249.454263218238,22.0319508329691)) ;
#116765=CARTESIAN_POINT('Ctrl Pts',(60.9402651077866,249.493637415392,22.0846181666045)) ;
#116766=CARTESIAN_POINT('Ctrl Pts',(60.9402651077865,249.524774012978,22.1262668017985)) ;
#116767=CARTESIAN_POINT('Ctrl Pts',(60.9402651077866,249.554098553236,22.1693335441747)) ;
#116768=CARTESIAN_POINT('Ctrl Pts',(60.9402651077865,249.581558206979,22.2136591533113)) ;
#116769=CARTESIAN_POINT('Ctrl Pts',(60.9402651077865,249.59646898522,22.2377282597327)) ;
#116770=CARTESIAN_POINT('Ctrl Pts',(60.9402651077866,249.610829665203,22.2621688070069)) ;
#116771=CARTESIAN_POINT('Ctrl Pts',(60.9402651077866,249.624630037462,22.2869568726434)) ;
#116772=CARTESIAN_POINT('Ctrl Pts',(60.9402651077866,249.630628989966,22.2977321202693)) ;
#116773=CARTESIAN_POINT('Ctrl Pts',(60.9402651077866,249.636521561056,22.3085723497387)) ;
#116774=CARTESIAN_POINT('Ctrl Pts',(60.9402651077866,249.642300957031,22.3194639045933)) ;
#116775=CARTESIAN_POINT('Ctrl Pts',(60.9402651077865,249.674107722661,22.3794053126736)) ;
#116776=CARTESIAN_POINT('Ctrl Pts',(60.9402651077867,249.702540340268,22.44098849303)) ;
#116777=CARTESIAN_POINT('Ctrl Pts',(60.9402651077866,249.727510761889,22.503853973586)) ;
#116778=CARTESIAN_POINT('Ctrl Pts',(60.9402651077866,249.752826501334,22.5675888255631)) ;
#116779=CARTESIAN_POINT('Ctrl Pts',(60.9402651077866,249.774584244754,22.6326425708184)) ;
#116780=CARTESIAN_POINT('Ctrl Pts',(60.9402651077865,249.792652789188,22.6986757373846)) ;
#116781=CARTESIAN_POINT('Ctrl Pts',(60.9402651077865,249.805016882959,22.7438614614688)) ;
#116782=CARTESIAN_POINT('Ctrl Pts',(60.9402651077865,249.815652686325,22.7895065347492)) ;
#116783=CARTESIAN_POINT('Ctrl Pts',(60.9402651077866,249.824505428491,22.8355081310719)) ;
#116784=CARTESIAN_POINT('Ctrl Pts',(60.9402651077867,249.828929431581,22.8584966244073)) ;
#116785=CARTESIAN_POINT('Ctrl Pts',(60.9402651077868,249.832907974007,22.8815742098594)) ;
#116786=CARTESIAN_POINT('Ctrl Pts',(60.9402651077866,249.836433132633,22.9047282989318)) ;
#116787=CARTESIAN_POINT('Ctrl Pts',(60.9402651077865,249.838694859355,22.9195838636081)) ;
#116788=CARTESIAN_POINT('Ctrl Pts',(60.9402651077866,249.840769937873,22.9344709232824)) ;
#116789=CARTESIAN_POINT('Ctrl Pts',(60.9402651077865,249.842656107631,22.9493861700344)) ;
#116790=CARTESIAN_POINT('Ctrl Pts',(60.9402651077865,249.844045727851,22.9603748567076)) ;
#116791=CARTESIAN_POINT('Ctrl Pts',(60.9402651077865,249.84533163955,22.9713696735096)) ;
#116792=CARTESIAN_POINT('Ctrl Pts',(60.9402651077865,249.84651329604,22.9823679509404)) ;
#116793=CARTESIAN_POINT('Ctrl Pts',(60.9402651077866,249.853975477243,23.0518222634181)) ;
#116794=CARTESIAN_POINT('Ctrl Pts',(60.9402651077866,249.857285781381,23.1214286108591)) ;
#116795=CARTESIAN_POINT('Ctrl Pts',(60.9402651077865,249.856319412001,23.1908363594129)) ;
#116796=CARTESIAN_POINT('Ctrl Pts',(60.9402651077864,249.856026793893,23.2118531305353)) ;
#116797=CARTESIAN_POINT('Ctrl Pts',(60.9402651077868,249.855341726161,23.2328518457626)) ;
#116798=CARTESIAN_POINT('Ctrl Pts',(60.9402651077867,249.854259856848,23.2538231020334)) ;
#116799=CARTESIAN_POINT('Ctrl Pts',(60.9402651077866,249.850793622953,23.3210135458965)) ;
#116800=CARTESIAN_POINT('Ctrl Pts',(60.9402651077866,249.843258202366,23.3879219235019)) ;
#116801=CARTESIAN_POINT('Ctrl Pts',(60.9402651077865,249.831876107148,23.4543055732081)) ;
#116802=CARTESIAN_POINT('Ctrl Pts',(60.9402651077864,249.825943828568,23.4889043263943)) ;
#116803=CARTESIAN_POINT('Ctrl Pts',(60.9402651077865,249.818965749739,23.5233606026032)) ;
#116804=CARTESIAN_POINT('Ctrl Pts',(60.9402651077864,249.810967923841,23.5576398472338)) ;
#116805=CARTESIAN_POINT('Ctrl Pts',(60.9402651077864,249.806632810109,23.5762204497635)) ;
#116806=CARTESIAN_POINT('Ctrl Pts',(60.9402651077864,249.801998028691,23.5947490326698)) ;
#116807=CARTESIAN_POINT('Ctrl Pts',(60.9402651077866,249.797067299182,23.6132200135793)) ;
#116808=CARTESIAN_POINT('Ctrl Pts',(60.9402651077867,249.794086739133,23.6243854745273)) ;
#116809=CARTESIAN_POINT('Ctrl Pts',(60.9402651077865,249.790998032701,23.6355298861929)) ;
#116810=CARTESIAN_POINT('Ctrl Pts',(60.9402651077866,249.787801949933,23.6466520013255)) ;
#116811=CARTESIAN_POINT('Ctrl Pts',(60.9402651077867,249.784265075083,23.6589600459386)) ;
#116812=CARTESIAN_POINT('Ctrl Pts',(60.9402651077866,249.780599005193,23.671232613158)) ;
#116813=CARTESIAN_POINT('Ctrl Pts',(60.9402651077866,249.776807401206,23.6834616436752)) ;
#116814=CARTESIAN_POINT('Ctrl Pts',(60.9402651077866,249.755950457756,23.7507313793397)) ;
#116815=CARTESIAN_POINT('Ctrl Pts',(60.9402651077866,249.731281914511,23.816745182075)) ;
#116816=CARTESIAN_POINT('Ctrl Pts',(60.9402651077866,249.703069382292,23.8812387082105)) ;
#116817=CARTESIAN_POINT('Ctrl Pts',(60.9402651077866,249.674856850073,23.9457322343459)) ;
#116818=CARTESIAN_POINT('Ctrl Pts',(60.9402651077867,249.643099881907,24.0087063454738)) ;
#116819=CARTESIAN_POINT('Ctrl Pts',(60.9402651077868,249.608013003586,24.0698922112783)) ;
#116820=CARTESIAN_POINT('Ctrl Pts',(60.9402651077869,249.572487613619,24.1318427707814)) ;
#116821=CARTESIAN_POINT('Ctrl Pts',(60.9402651077866,249.53354820023,24.1919610672433)) ;
#116822=CARTESIAN_POINT('Ctrl Pts',(60.9402651077867,249.491368953434,24.2499496790592)) ;
#116823=CARTESIAN_POINT('Ctrl Pts',(60.9402651077867,249.481720037426,24.2632151422266)) ;
#116824=CARTESIAN_POINT('Ctrl Pts',(60.9402651077867,249.471901392435,24.2763690469256)) ;
#116825=CARTESIAN_POINT('Ctrl Pts',(60.9402651077868,249.461914784373,24.2894076162287)) ;
#116826=CARTESIAN_POINT('Ctrl Pts',(60.9402651077868,249.454834323785,24.2986519037288)) ;
#116827=CARTESIAN_POINT('Ctrl Pts',(60.9402651077866,249.44766976387,24.3078376489109)) ;
#116828=CARTESIAN_POINT('Ctrl Pts',(60.9402651077866,249.440430193774,24.3169532133058)) ;
#116829=CARTESIAN_POINT('Ctrl Pts',(60.9402651077866,249.394852937774,24.3743409319824)) ;
#116830=CARTESIAN_POINT('Ctrl Pts',(60.9402651077865,249.346224208465,24.4290572871775)) ;
#116831=CARTESIAN_POINT('Ctrl Pts',(60.9402651077866,249.294783585182,24.4808204376118)) ;
#116832=CARTESIAN_POINT('Ctrl Pts',(60.9402651077867,249.243428794205,24.5324972175814)) ;
#116833=CARTESIAN_POINT('Ctrl Pts',(60.9402651077866,249.189270959674,24.5812315801778)) ;
#116834=CARTESIAN_POINT('Ctrl Pts',(60.9402651077867,249.132502121971,24.6267202980104)) ;
#116835=CARTESIAN_POINT('Ctrl Pts',(60.9402651077868,249.077177770065,24.6710515532367)) ;
#116836=CARTESIAN_POINT('Ctrl Pts',(60.9402651077868,249.019372982206,24.7123009755837)) ;
#116837=CARTESIAN_POINT('Ctrl Pts',(60.9402651077867,248.959230111589,24.7501540590356)) ;
#116838=CARTESIAN_POINT('Ctrl Pts',(60.9402651077867,248.937186588349,24.7640279449378)) ;
#116839=CARTESIAN_POINT('Ctrl Pts',(60.9402651077866,248.914828670669,24.7774451898368)) ;
#116840=CARTESIAN_POINT('Ctrl Pts',(60.9402651077866,248.892162375845,24.7903888257488)) ;
#116841=CARTESIAN_POINT('Origin',(60.9402651077866,248.040265107786,23.0213203435596)) ;
#116842=CARTESIAN_POINT('Ctrl Pts',(60.9402651077865,247.14398687089,24.7683227969254)) ;
#116843=CARTESIAN_POINT('Ctrl Pts',(60.9402651077865,247.110696623296,24.7483652569324)) ;
#116844=CARTESIAN_POINT('Ctrl Pts',(60.9402651077865,247.078078487436,24.7273686112138)) ;
#116845=CARTESIAN_POINT('Ctrl Pts',(60.9402651077865,247.046187815054,24.7053297595934)) ;
#116846=CARTESIAN_POINT('Ctrl Pts',(60.9402651077865,246.986660772535,24.6641920989713)) ;
#116847=CARTESIAN_POINT('Ctrl Pts',(60.9402651077865,246.929665910612,24.6194250575563)) ;
#116848=CARTESIAN_POINT('Ctrl Pts',(60.9402651077866,246.875361631822,24.5713686455035)) ;
#116849=CARTESIAN_POINT('Ctrl Pts',(60.9402651077866,246.857636515018,24.5556828554362)) ;
#116850=CARTESIAN_POINT('Ctrl Pts',(60.9402651077866,246.84019837111,24.5396463558629)) ;
#116851=CARTESIAN_POINT('Ctrl Pts',(60.9402651077867,246.823053678133,24.5232702993519)) ;
#116852=CARTESIAN_POINT('Ctrl Pts',(60.9402651077867,246.810403115074,24.5111868904612)) ;
#116853=CARTESIAN_POINT('Ctrl Pts',(60.9402651077867,246.797912332271,24.4989186024479)) ;
#116854=CARTESIAN_POINT('Ctrl Pts',(60.9402651077866,246.785584111923,24.4864698302042)) ;
#116855=CARTESIAN_POINT('Ctrl Pts',(60.9402651077866,246.774650795282,24.4754296017774)) ;
#116856=CARTESIAN_POINT('Ctrl Pts',(60.9402651077867,246.763851231069,24.4642533032112)) ;
#116857=CARTESIAN_POINT('Ctrl Pts',(60.9402651077867,246.753191015033,24.4529488260821)) ;
#116858=CARTESIAN_POINT('Ctrl Pts',(60.9402651077866,246.703495389042,24.4002497939465)) ;
#116859=CARTESIAN_POINT('Ctrl Pts',(60.9402651077865,246.656795094732,24.3447378110376)) ;
#116860=CARTESIAN_POINT('Ctrl Pts',(60.9402651077865,246.613248450744,24.2867545689444)) ;
#116861=CARTESIAN_POINT('Ctrl Pts',(60.9402651077865,246.581310448125,24.2442284689238)) ;
#116862=CARTESIAN_POINT('Ctrl Pts',(60.9402651077867,246.55106963218,24.2003722343513)) ;
#116863=CARTESIAN_POINT('Ctrl Pts',(60.9402651077866,246.522604506068,24.1553129600453)) ;
#116864=CARTESIAN_POINT('Ctrl Pts',(60.9402651077866,246.510616937053,24.136337067987)) ;
#116865=CARTESIAN_POINT('Ctrl Pts',(60.9402651077867,246.498944465043,24.11714775866)) ;
#116866=CARTESIAN_POINT('Ctrl Pts',(60.9402651077866,246.487593742736,24.0977543412124)) ;
#116867=CARTESIAN_POINT('Ctrl Pts',(60.9402651077865,246.480956285133,24.08641383066)) ;
#116868=CARTESIAN_POINT('Ctrl Pts',(60.9402651077866,246.474428082592,24.0750019825718)) ;
#116869=CARTESIAN_POINT('Ctrl Pts',(60.9402651077866,246.468018497233,24.0635353483554)) ;
#116870=CARTESIAN_POINT('Ctrl Pts',(60.9402651077868,246.433160377772,24.0011747925748)) ;
#116871=CARTESIAN_POINT('Ctrl Pts',(60.9402651077867,246.401752337816,23.937105062428)) ;
#116872=CARTESIAN_POINT('Ctrl Pts',(60.9402651077866,246.373944316263,23.8716485339039)) ;
#116873=CARTESIAN_POINT('Ctrl Pts',(60.9402651077865,246.346636811236,23.8073701573079)) ;
#116874=CARTESIAN_POINT('Ctrl Pts',(60.9402651077868,246.32280067199,23.7417534653275)) ;
#116875=CARTESIAN_POINT('Ctrl Pts',(60.9402651077867,246.302625236177,23.6750905947637)) ;
#116876=CARTESIAN_POINT('Ctrl Pts',(60.9402651077866,246.288518996942,23.6284813215364)) ;
#116877=CARTESIAN_POINT('Ctrl Pts',(60.9402651077865,246.276203267621,23.5813603419321)) ;
#116878=CARTESIAN_POINT('Ctrl Pts',(60.9402651077867,246.265757835163,23.53382736178)) ;
#116879=CARTESIAN_POINT('Ctrl Pts',(60.9402651077868,246.257092882906,23.4943966340122)) ;
#116880=CARTESIAN_POINT('Ctrl Pts',(60.9402651077865,246.249715171408,23.454682352912)) ;
#116881=CARTESIAN_POINT('Ctrl Pts',(60.9402651077866,246.243677247182,23.414742639793)) ;
#116882=CARTESIAN_POINT('Ctrl Pts',(60.9402651077867,246.241926884875,23.4031643281448)) ;
#116883=CARTESIAN_POINT('Ctrl Pts',(60.9402651077865,246.240289232283,23.3915669160736)) ;
#116884=CARTESIAN_POINT('Ctrl Pts',(60.9402651077865,246.23876732204,23.3799665803396)) ;
#116885=CARTESIAN_POINT('Ctrl Pts',(60.9402651077868,246.229937787811,23.312665921877)) ;
#116886=CARTESIAN_POINT('Ctrl Pts',(60.9402651077865,246.224980478258,23.2451443288552)) ;
#116887=CARTESIAN_POINT('Ctrl Pts',(60.9402651077866,246.224066368655,23.177676364878)) ;
#116888=CARTESIAN_POINT('Ctrl Pts',(60.9402651077867,246.223715971633,23.1518145059036)) ;
#116889=CARTESIAN_POINT('Ctrl Pts',(60.9402651077866,246.22396019596,23.1259605167808)) ;
#116890=CARTESIAN_POINT('Ctrl Pts',(60.9402651077866,246.22481072392,23.1001299806353)) ;
#116891=CARTESIAN_POINT('Ctrl Pts',(60.9402651077866,246.227062239739,23.0317514399507)) ;
#116892=CARTESIAN_POINT('Ctrl Pts',(60.9402651077865,246.23355904935,22.9635359717512)) ;
#116893=CARTESIAN_POINT('Ctrl Pts',(60.9402651077865,246.244123442748,22.895788639393)) ;
#116894=CARTESIAN_POINT('Ctrl Pts',(60.9402651077865,246.249247050823,22.8629319701989)) ;
#116895=CARTESIAN_POINT('Ctrl Pts',(60.9402651077865,246.255328156535,22.8301856656148)) ;
#116896=CARTESIAN_POINT('Ctrl Pts',(60.9402651077864,246.262350374056,22.7975864532994)) ;
#116897=CARTESIAN_POINT('Ctrl Pts',(60.9402651077864,246.266430574556,22.7786449548353)) ;
#116898=CARTESIAN_POINT('Ctrl Pts',(60.9402651077865,246.270828547796,22.759753143661)) ;
#116899=CARTESIAN_POINT('Ctrl Pts',(60.9402651077865,246.275541428506,22.7409184880431)) ;
#116900=CARTESIAN_POINT('Ctrl Pts',(60.9402651077866,246.278434058103,22.7293583222674)) ;
#116901=CARTESIAN_POINT('Ctrl Pts',(60.9402651077867,246.281445780643,22.7178180138917)) ;
#116902=CARTESIAN_POINT('Ctrl Pts',(60.9402651077867,246.284574538954,22.7063046079789)) ;
#116903=CARTESIAN_POINT('Ctrl Pts',(60.9402651077867,246.302289420104,22.6411162498198)) ;
#116904=CARTESIAN_POINT('Ctrl Pts',(60.9402651077866,246.323683070667,22.5770382879317)) ;
#116905=CARTESIAN_POINT('Ctrl Pts',(60.9402651077866,246.348552607161,22.5143506693262)) ;
#116906=CARTESIAN_POINT('Ctrl Pts',(60.9402651077866,246.373476863233,22.4515251213285)) ;
#116907=CARTESIAN_POINT('Ctrl Pts',(60.9402651077865,246.401892937332,22.3900951413175)) ;
#116908=CARTESIAN_POINT('Ctrl Pts',(60.9402651077866,246.433642655425,22.3303661652523)) ;
#116909=CARTESIAN_POINT('Ctrl Pts',(60.9402651077867,246.465163048057,22.2710686064036)) ;
#116910=CARTESIAN_POINT('Ctrl Pts',(60.9402651077867,246.499969738244,22.2134467522368)) ;
#116911=CARTESIAN_POINT('Ctrl Pts',(60.9402651077868,246.537943823293,22.1578354708785)) ;
#116912=CARTESIAN_POINT('Ctrl Pts',(60.9402651077868,246.547010825524,22.1445572678233)) ;
#116913=CARTESIAN_POINT('Ctrl Pts',(60.9402651077867,246.556258539357,22.1313938813587)) ;
#116914=CARTESIAN_POINT('Ctrl Pts',(60.9402651077867,246.565685590736,22.1183502553737)) ;
#116915=CARTESIAN_POINT('Ctrl Pts',(60.9402651077867,246.575081295221,22.10535000214)) ;
#116916=CARTESIAN_POINT('Ctrl Pts',(60.9402651077867,246.584658747915,22.0924642306346)) ;
#116917=CARTESIAN_POINT('Ctrl Pts',(60.9402651077866,246.594396472188,22.0797237413789)) ;
#116918=CARTESIAN_POINT('Ctrl Pts',(60.9402651077865,246.634516348228,22.0272323342157)) ;
#116919=CARTESIAN_POINT('Ctrl Pts',(60.9402651077865,246.677403336317,21.9771313640338)) ;
#116920=CARTESIAN_POINT('Ctrl Pts',(60.9402651077865,246.722906620125,21.9297036362799)) ;
#116921=CARTESIAN_POINT('Ctrl Pts',(60.9402651077866,246.767658732713,21.8830588485941)) ;
#116922=CARTESIAN_POINT('Ctrl Pts',(60.9402651077868,246.814942126786,21.8389991203923)) ;
#116923=CARTESIAN_POINT('Ctrl Pts',(60.9402651077867,246.864643798312,21.7978329077263)) ;
#116924=CARTESIAN_POINT('Ctrl Pts',(60.9402651077866,246.912679449409,21.7580466034055)) ;
#116925=CARTESIAN_POINT('Ctrl Pts',(60.9402651077866,246.962974558538,21.7209626850137)) ;
#116926=CARTESIAN_POINT('Ctrl Pts',(60.9402651077867,247.015446740337,21.686904114294)) ;
#116927=CARTESIAN_POINT('Ctrl Pts',(60.9402651077867,247.03205539854,21.6761237895472)) ;
#116928=CARTESIAN_POINT('Ctrl Pts',(60.9402651077866,247.048882288002,21.6656469321673)) ;
#116929=CARTESIAN_POINT('Ctrl Pts',(60.9402651077866,247.065925086493,21.6554848536835)) ;
#116930=CARTESIAN_POINT('Ctrl Pts',(61.1067325548923,246.899092893641,21.4203834081426)) ;
#116931=CARTESIAN_POINT('Ctrl Pts',(61.080348061988,246.368276064864,21.7987339961471)) ;
#116932=CARTESIAN_POINT('Ctrl Pts',(61.0275887537553,245.722609719904,23.1197710503415)) ;
#116933=CARTESIAN_POINT('Ctrl Pts',(60.948454630194,246.859463067054,25.0213439274063)) ;
#116934=CARTESIAN_POINT('Ctrl Pts',(60.8693301842085,249.073180249221,25.1000285863252)) ;
#116935=CARTESIAN_POINT('Ctrl Pts',(60.7902057382229,250.346067934117,23.2890963835466)) ;
#116936=CARTESIAN_POINT('Ctrl Pts',(60.7110812922374,249.521590130723,21.2338246910011)) ;
#116937=CARTESIAN_POINT('Ctrl Pts',(60.6319568462519,247.349118393682,20.8052161888267)) ;
#116938=CARTESIAN_POINT('Ctrl Pts',(60.5528324002664,245.805585994569,22.3927343089783)) ;
#116939=CARTESIAN_POINT('Ctrl Pts',(60.4737079542808,246.295184926232,24.5522333747062)) ;
#116940=CARTESIAN_POINT('Ctrl Pts',(60.3945835082953,248.372537959759,25.3188246765677)) ;
#116941=CARTESIAN_POINT('Ctrl Pts',(60.3154590623098,250.147567314984,23.9950884285102)) ;
#116942=CARTESIAN_POINT('Ctrl Pts',(60.2363346163243,250.005310554343,21.7853793507168)) ;
#116943=CARTESIAN_POINT('Ctrl Pts',(60.1572101703387,248.075189857469,20.7001725272112)) ;
#116944=CARTESIAN_POINT('Ctrl Pts',(60.0780857243532,246.113294619792,21.7268190366224)) ;
#116945=CARTESIAN_POINT('Ctrl Pts',(59.9989612783677,245.904618567983,23.9312451899875)) ;
#116946=CARTESIAN_POINT('Ctrl Pts',(59.9198368323822,247.639022645035,25.307792121131)) ;
#116947=CARTESIAN_POINT('Ctrl Pts',(59.8407123863967,249.738489903116,24.6040336728245)) ;
#116948=CARTESIAN_POINT('Ctrl Pts',(59.7615879404111,250.292857693394,22.4602716766755)) ;
#116949=CARTESIAN_POINT('Ctrl Pts',(59.6824634944256,248.797744299413,20.8269698304018)) ;
#116950=CARTESIAN_POINT('Ctrl Pts',(59.6033390484401,246.613451994329,21.1901586184867)) ;
#116951=CARTESIAN_POINT('Ctrl Pts',(59.5242146024546,245.727320128136,23.2193972255469)) ;
#116952=CARTESIAN_POINT('Ctrl Pts',(59.4450901564691,246.945579975629,25.0684191163454)) ;
#116953=CARTESIAN_POINT('Ctrl Pts',(59.3659657104835,249.159819545126,25.0549247205655)) ;
#116954=CARTESIAN_POINT('Ctrl Pts',(59.286841264498,250.355452505948,23.1911916911607)) ;
#116955=CARTESIAN_POINT('Ctrl Pts',(59.2077168185125,249.444653504094,21.1729042187596)) ;
#116956=CARTESIAN_POINT('Ctrl Pts',(59.1285923725269,247.256096849426,20.8363652304909)) ;
#116957=CARTESIAN_POINT('Ctrl Pts',(59.0494679265414,245.78100155116,22.4877685177501)) ;
#116958=CARTESIAN_POINT('Ctrl Pts',(58.9703434805559,246.361457172664,24.624614705875)) ;
#116959=CARTESIAN_POINT('Ctrl Pts',(58.8912190345704,248.469345593264,25.3027314990645)) ;
#116960=CARTESIAN_POINT('Ctrl Pts',(58.8120945885848,250.186844164077,23.9051484376557)) ;
#116961=CARTESIAN_POINT('Ctrl Pts',(58.7329701425994,249.951313140653,21.7034272174656)) ;
#116962=CARTESIAN_POINT('Ctrl Pts',(58.6538456966138,247.977055527801,20.7007738653896)) ;
#116963=CARTESIAN_POINT('Ctrl Pts',(58.5747212506283,246.060294351269,21.8094146738284)) ;
#116964=CARTESIAN_POINT('Ctrl Pts',(58.4955968046428,245.945003682052,24.0207155105206)) ;
#116965=CARTESIAN_POINT('Ctrl Pts',(58.4164723586572,247.735985960427,25.3226711654736)) ;
#116966=CARTESIAN_POINT('Ctrl Pts',(58.3373479126717,249.803947954416,24.5309187497578)) ;
#116967=CARTESIAN_POINT('Ctrl Pts',(58.2582234666862,250.266963056667,22.365388238877)) ;
#116968=CARTESIAN_POINT('Ctrl Pts',(58.1790990207007,248.704697564139,20.7972539868847)) ;
#116969=CARTESIAN_POINT('Ctrl Pts',(58.0999745747151,246.536593225254,21.2511907819118)) ;
#116970=CARTESIAN_POINT('Ctrl Pts',(58.0208501287296,245.739715191048,23.3181208433496)) ;
#116971=CARTESIAN_POINT('Ctrl Pts',(57.9681004980726,246.600182354009,24.5099551564717)) ;
#116972=CARTESIAN_POINT('Ctrl Pts',(57.9417256827441,247.187270248071,24.7926681085687)) ;
#116973=CARTESIAN_POINT('Ctrl Pts',(61.0506450234148,246.955481069846,21.4994897103189)) ;
#116974=CARTESIAN_POINT('Ctrl Pts',(61.0242605305105,246.450893229562,21.8591450485099)) ;
#116975=CARTESIAN_POINT('Ctrl Pts',(60.9715012222777,245.837130875234,23.1149063544326)) ;
#116976=CARTESIAN_POINT('Ctrl Pts',(60.8923670987165,246.91780945221,24.9225177547551)) ;
#116977=CARTESIAN_POINT('Ctrl Pts',(60.813242652731,249.022141326017,24.9973144076774)) ;
#116978=CARTESIAN_POINT('Ctrl Pts',(60.7341182067454,250.232132443528,23.2758648989914)) ;
#116979=CARTESIAN_POINT('Ctrl Pts',(60.6549937607599,249.448394152609,21.3221493264703)) ;
#116980=CARTESIAN_POINT('Ctrl Pts',(60.5758693147743,247.38326968322,20.9147194434772)) ;
#116981=CARTESIAN_POINT('Ctrl Pts',(60.4967448687889,245.916007084424,22.4237943187109)) ;
#116982=CARTESIAN_POINT('Ctrl Pts',(60.4176204228033,246.381413707085,24.4765871289558)) ;
#116983=CARTESIAN_POINT('Ctrl Pts',(60.3384959768178,248.356119526246,25.2052992353106)) ;
#116984=CARTESIAN_POINT('Ctrl Pts',(60.2593715308323,250.043440236965,23.9469721094513)) ;
#116985=CARTESIAN_POINT('Ctrl Pts',(60.1802470848468,249.908212739029,21.8464502895457)) ;
#116986=CARTESIAN_POINT('Ctrl Pts',(60.1011226388612,248.073464138147,20.8148662521754)) ;
#116987=CARTESIAN_POINT('Ctrl Pts',(60.0219981928757,246.208511056077,21.7907835871857)) ;
#116988=CARTESIAN_POINT('Ctrl Pts',(59.9428737468902,246.010146210441,23.8862835251857)) ;
#116989=CARTESIAN_POINT('Ctrl Pts',(59.8637493009047,247.658849039693,25.1948118260597)) ;
#116990=CARTESIAN_POINT('Ctrl Pts',(59.7846248549191,249.654576364206,24.5258278446539)) ;
#116991=CARTESIAN_POINT('Ctrl Pts',(59.7055004089336,250.18155145402,22.4879944959797)) ;
#116992=CARTESIAN_POINT('Ctrl Pts',(59.6263759629481,248.760315356087,20.9353981831583)) ;
#116993=CARTESIAN_POINT('Ctrl Pts',(59.5472515169626,246.683954402516,21.2806409039238)) ;
#116994=CARTESIAN_POINT('Ctrl Pts',(59.468127070977,245.841608530402,23.2096097508913)) ;
#116995=CARTESIAN_POINT('Ctrl Pts',(59.3890026249916,246.999671108725,24.9672668407485)) ;
#116996=CARTESIAN_POINT('Ctrl Pts',(59.309878179006,249.104499557396,24.9544392368494)) ;
#116997=CARTESIAN_POINT('Ctrl Pts',(59.2307537330205,250.24105330017,23.1827979225761)) ;
#116998=CARTESIAN_POINT('Ctrl Pts',(59.151629287035,249.375259157325,21.2642390872863)) ;
#116999=CARTESIAN_POINT('Ctrl Pts',(59.0725048410494,247.29484456636,20.9443293330062)) ;
#117000=CARTESIAN_POINT('Ctrl Pts',(58.9933803950639,245.892637419915,22.5141326492943)) ;
#117001=CARTESIAN_POINT('Ctrl Pts',(58.9142559490784,246.444411275898,24.5453919173336)) ;
#117002=CARTESIAN_POINT('Ctrl Pts',(58.8351315030929,248.448143652206,25.1900012619997)) ;
#117003=CARTESIAN_POINT('Ctrl Pts',(58.7560070571073,250.080776318608,23.8614762787238)) ;
#117004=CARTESIAN_POINT('Ctrl Pts',(58.6768826111218,249.85688347274,21.7685476163785)) ;
#117005=CARTESIAN_POINT('Ctrl Pts',(58.5977581651363,247.980178871404,20.8154378767288)) ;
#117006=CARTESIAN_POINT('Ctrl Pts',(58.5186337191508,246.158129663517,21.8692979671662)) ;
#117007=CARTESIAN_POINT('Ctrl Pts',(58.4395092731652,246.048535794914,23.9713328931781)) ;
#117008=CARTESIAN_POINT('Ctrl Pts',(58.3603848271797,247.751021154908,25.2089556595693)) ;
#117009=CARTESIAN_POINT('Ctrl Pts',(58.2812603811942,249.716799969307,24.4563257129906)) ;
#117010=CARTESIAN_POINT('Ctrl Pts',(58.2021359352087,250.156936336125,22.3977994863984)) ;
#117011=CARTESIAN_POINT('Ctrl Pts',(58.1230114892231,248.671866292958,20.9071506738677)) ;
#117012=CARTESIAN_POINT('Ctrl Pts',(58.0438870432376,246.610893417648,21.3386573153505)) ;
#117013=CARTESIAN_POINT('Ctrl Pts',(57.9647625972521,245.853391122223,23.3034551875683)) ;
#117014=CARTESIAN_POINT('Ctrl Pts',(57.9120129665951,246.671340448346,24.4363979833345)) ;
#117015=CARTESIAN_POINT('Ctrl Pts',(57.8856381512666,247.229418859696,24.7051413806521)) ;
#117016=CARTESIAN_POINT('Ctrl Pts',(60.9945574919372,247.011869246051,21.5785960124951)) ;
#117017=CARTESIAN_POINT('Ctrl Pts',(60.9681729990329,246.533510394261,21.9195561008726)) ;
#117018=CARTESIAN_POINT('Ctrl Pts',(60.9154136908002,245.951652030563,23.1100416585237)) ;
#117019=CARTESIAN_POINT('Ctrl Pts',(60.836279567239,246.976155837366,24.8236915821038)) ;
#117020=CARTESIAN_POINT('Ctrl Pts',(60.7571551212534,248.971102402814,24.8946002290295)) ;
#117021=CARTESIAN_POINT('Ctrl Pts',(60.6780306752679,250.118196952939,23.2626334144363)) ;
#117022=CARTESIAN_POINT('Ctrl Pts',(60.5989062292824,249.375198174497,21.4104739619396)) ;
#117023=CARTESIAN_POINT('Ctrl Pts',(60.5197817832969,247.417420972759,21.0242226981276)) ;
#117024=CARTESIAN_POINT('Ctrl Pts',(60.4406573373113,246.026428174279,22.4548543284435)) ;
#117025=CARTESIAN_POINT('Ctrl Pts',(60.3615328913258,246.467642487938,24.4009408832055)) ;
#117026=CARTESIAN_POINT('Ctrl Pts',(60.2824084453403,248.339701092733,25.0917737940535)) ;
#117027=CARTESIAN_POINT('Ctrl Pts',(60.2032839993548,249.939313158944,23.8988557903925)) ;
#117028=CARTESIAN_POINT('Ctrl Pts',(60.1241595533693,249.811114923714,21.9075212283746)) ;
#117029=CARTESIAN_POINT('Ctrl Pts',(60.0450351073837,248.071738418825,20.9295599771395)) ;
#117030=CARTESIAN_POINT('Ctrl Pts',(59.9659106613982,246.303727492363,21.854748137749)) ;
#117031=CARTESIAN_POINT('Ctrl Pts',(59.8867862154127,246.1156738529,23.8413218603838)) ;
#117032=CARTESIAN_POINT('Ctrl Pts',(59.8076617694271,247.67867543435,25.0818315309884)) ;
#117033=CARTESIAN_POINT('Ctrl Pts',(59.7285373234416,249.570662825296,24.4476220164834)) ;
#117034=CARTESIAN_POINT('Ctrl Pts',(59.6494128774561,250.070245214644,22.515717315284)) ;
#117035=CARTESIAN_POINT('Ctrl Pts',(59.5702884314706,248.722886412761,21.0438265359149)) ;
#117036=CARTESIAN_POINT('Ctrl Pts',(59.4911639854851,246.754456810702,21.3711231893609)) ;
#117037=CARTESIAN_POINT('Ctrl Pts',(59.4120395394995,245.955896932668,23.1998222762357)) ;
#117038=CARTESIAN_POINT('Ctrl Pts',(59.332915093514,247.053762241821,24.8661145651516)) ;
#117039=CARTESIAN_POINT('Ctrl Pts',(59.2537906475285,249.049179569667,24.8539537531333)) ;
#117040=CARTESIAN_POINT('Ctrl Pts',(59.174666201543,250.126654094392,23.1744041539915)) ;
#117041=CARTESIAN_POINT('Ctrl Pts',(59.0955417555573,249.305864810557,21.355573955813)) ;
#117042=CARTESIAN_POINT('Ctrl Pts',(59.0164173095719,247.333592283294,21.0522934355215)) ;
#117043=CARTESIAN_POINT('Ctrl Pts',(58.9372928635864,246.004273288669,22.5404967808384)) ;
#117044=CARTESIAN_POINT('Ctrl Pts',(58.8581684176009,246.527365379132,24.4661691287921)) ;
#117045=CARTESIAN_POINT('Ctrl Pts',(58.7790439716154,248.426941711148,25.0772710249347)) ;
#117046=CARTESIAN_POINT('Ctrl Pts',(58.6999195256298,249.974708473138,23.817804119792)) ;
#117047=CARTESIAN_POINT('Ctrl Pts',(58.6207950796443,249.762453804827,21.8336680152914)) ;
#117048=CARTESIAN_POINT('Ctrl Pts',(58.5416706336588,247.983302215006,20.9301018880681)) ;
#117049=CARTESIAN_POINT('Ctrl Pts',(58.4625461876733,246.255964975764,21.9291812605039)) ;
#117050=CARTESIAN_POINT('Ctrl Pts',(58.3834217416877,246.152067907775,23.9219502758357)) ;
#117051=CARTESIAN_POINT('Ctrl Pts',(58.3042972957023,247.76605634939,25.095240153665)) ;
#117052=CARTESIAN_POINT('Ctrl Pts',(58.2251728497167,249.629651984198,24.3817326762235)) ;
#117053=CARTESIAN_POINT('Ctrl Pts',(58.1460484037312,250.046909615583,22.4302107339199)) ;
#117054=CARTESIAN_POINT('Ctrl Pts',(58.0669239577456,248.639035021779,21.0170473608507)) ;
#117055=CARTESIAN_POINT('Ctrl Pts',(57.9877995117601,246.685193610043,21.426123848789)) ;
#117056=CARTESIAN_POINT('Ctrl Pts',(57.9086750657746,245.967067053397,23.288789531787)) ;
#117057=CARTESIAN_POINT('Ctrl Pts',(57.8559254351176,246.742498542684,24.3628408101973)) ;
#117058=CARTESIAN_POINT('Ctrl Pts',(57.8295506197891,247.271567471321,24.6176146527354)) ;
#117059=CARTESIAN_POINT('Ctrl Pts',(60.9384699604597,247.068257422256,21.6577023146713)) ;
#117060=CARTESIAN_POINT('Ctrl Pts',(60.9120854675554,246.616127558959,21.9799671532354)) ;
#117061=CARTESIAN_POINT('Ctrl Pts',(60.8593261593227,246.066173185893,23.1051769626147)) ;
#117062=CARTESIAN_POINT('Ctrl Pts',(60.7801920357613,247.034502222522,24.7248654094525)) ;
#117063=CARTESIAN_POINT('Ctrl Pts',(60.7010675897758,248.92006347961,24.7918860503816)) ;
#117064=CARTESIAN_POINT('Ctrl Pts',(60.6219431437903,250.004261462351,23.2494019298812)) ;
#117065=CARTESIAN_POINT('Ctrl Pts',(60.5428186978048,249.302002196383,21.4987985974089)) ;
#117066=CARTESIAN_POINT('Ctrl Pts',(60.4636942518192,247.451572262297,21.133725952778)) ;
#117067=CARTESIAN_POINT('Ctrl Pts',(60.3845698058337,246.136849264134,22.4859143381761)) ;
#117068=CARTESIAN_POINT('Ctrl Pts',(60.3054453598482,246.553871268792,24.3252946374551)) ;
#117069=CARTESIAN_POINT('Ctrl Pts',(60.2263209138627,248.32328265922,24.9782483527963)) ;
#117070=CARTESIAN_POINT('Ctrl Pts',(60.1471964678772,249.835186080924,23.8507394713336)) ;
#117071=CARTESIAN_POINT('Ctrl Pts',(60.0680720218916,249.714017108399,21.9685921672034)) ;
#117072=CARTESIAN_POINT('Ctrl Pts',(59.9889475759061,248.070012699505,21.0442537021036)) ;
#117073=CARTESIAN_POINT('Ctrl Pts',(59.9098231299206,246.398943928648,21.9187126883123)) ;
#117074=CARTESIAN_POINT('Ctrl Pts',(59.8306986839351,246.221201495357,23.7963601955819)) ;
#117075=CARTESIAN_POINT('Ctrl Pts',(59.7515742379496,247.698501829009,24.9688512359172)) ;
#117076=CARTESIAN_POINT('Ctrl Pts',(59.672449791964,249.486749286386,24.3694161883128)) ;
#117077=CARTESIAN_POINT('Ctrl Pts',(59.5933253459785,249.95893897527,22.5434401345883)) ;
#117078=CARTESIAN_POINT('Ctrl Pts',(59.5142008999929,248.685457469433,21.1522548886714)) ;
#117079=CARTESIAN_POINT('Ctrl Pts',(59.4350764540075,246.82495921889,21.4616054747979)) ;
#117080=CARTESIAN_POINT('Ctrl Pts',(59.3559520080219,246.070185334933,23.1900348015801)) ;
#117081=CARTESIAN_POINT('Ctrl Pts',(59.2768275620364,247.107853374917,24.7649622895547)) ;
#117082=CARTESIAN_POINT('Ctrl Pts',(59.1977031160509,248.993859581938,24.7534682694172)) ;
#117083=CARTESIAN_POINT('Ctrl Pts',(59.1185786700654,250.012254888613,23.166010385407)) ;
#117084=CARTESIAN_POINT('Ctrl Pts',(59.0394542240798,249.236470463788,21.4469088243396)) ;
#117085=CARTESIAN_POINT('Ctrl Pts',(58.9603297780943,247.372340000228,21.1602575380368)) ;
#117086=CARTESIAN_POINT('Ctrl Pts',(58.8812053321088,246.115909157423,22.5668609123824)) ;
#117087=CARTESIAN_POINT('Ctrl Pts',(58.8020808861232,246.610319482365,24.3869463402507)) ;
#117088=CARTESIAN_POINT('Ctrl Pts',(58.7229564401378,248.40573977009,24.9645407878698)) ;
#117089=CARTESIAN_POINT('Ctrl Pts',(58.6438319941522,249.86864062767,23.7741319608601)) ;
#117090=CARTESIAN_POINT('Ctrl Pts',(58.5647075481667,249.668024136914,21.8987884142042)) ;
#117091=CARTESIAN_POINT('Ctrl Pts',(58.4855831021812,247.986425558609,21.0447658994073)) ;
#117092=CARTESIAN_POINT('Ctrl Pts',(58.4064586561957,246.353800288012,21.9890645538417)) ;
#117093=CARTESIAN_POINT('Ctrl Pts',(58.3273342102101,246.255600020638,23.8725676584932)) ;
#117094=CARTESIAN_POINT('Ctrl Pts',(58.2482097642246,247.781091543872,24.9815246477607)) ;
#117095=CARTESIAN_POINT('Ctrl Pts',(58.1690853182391,249.542503999089,24.3071396394564)) ;
#117096=CARTESIAN_POINT('Ctrl Pts',(58.0899608722536,249.93688289504,22.4626219814414)) ;
#117097=CARTESIAN_POINT('Ctrl Pts',(58.010836426268,248.6062037506,21.1269440478337)) ;
#117098=CARTESIAN_POINT('Ctrl Pts',(57.9317119802825,246.759493802438,21.5135903822277)) ;
#117099=CARTESIAN_POINT('Ctrl Pts',(57.8525875342969,246.080742984571,23.2741238760057)) ;
#117100=CARTESIAN_POINT('Ctrl Pts',(57.79983790364,246.813656637022,24.2892836370601)) ;
#117101=CARTESIAN_POINT('Ctrl Pts',(57.7734630883115,247.313716082947,24.5300879248187)) ;
#117102=CARTESIAN_POINT('Origin',(67.9402651077866,248.040265107786,23.0213203435596)) ;
#117103=CARTESIAN_POINT('Origin',(55.9402651077866,248.040265107786,23.0213203435596)) ;
#117146=UNCERTAINTY_MEASURE_WITH_UNIT(LENGTH_MEASURE(0.01),#117171,
'DISTANCE_ACCURACY_VALUE',
'Maximum model space distance between geometric entities at asserted c
onnectivities') ;
#117147=UNCERTAINTY_MEASURE_WITH_UNIT(LENGTH_MEASURE(0.01),#117171,
'DISTANCE_ACCURACY_VALUE',
'Maximum model space distance between geometric entities at asserted c
onnectivities') ;
#117169=(
GEOMETRIC_REPRESENTATION_CONTEXT(3)
GLOBAL_UNCERTAINTY_ASSIGNED_CONTEXT((#117146))
GLOBAL_UNIT_ASSIGNED_CONTEXT((#117171,#117173,#117174))
REPRESENTATION_CONTEXT('','3D')
) ;
#117170=(
GEOMETRIC_REPRESENTATION_CONTEXT(3)
GLOBAL_UNCERTAINTY_ASSIGNED_CONTEXT((#117147))
GLOBAL_UNIT_ASSIGNED_CONTEXT((#117171,#117173,#117174))
REPRESENTATION_CONTEXT('','3D')
) ;
#117171=(
LENGTH_UNIT()
NAMED_UNIT(*)
SI_UNIT(.MILLI.,.METRE.)
) ;
#117173=(
NAMED_UNIT(*)
PLANE_ANGLE_UNIT()
SI_UNIT($,.RADIAN.)
) ;
#117174=(
NAMED_UNIT(*)
SI_UNIT($,.STERADIAN.)
SOLID_ANGLE_UNIT()
) ;
#117196=SHAPE_DEFINITION_REPRESENTATION(#117218,#117261) ;
#117218=PRODUCT_DEFINITION_SHAPE('',$,#117284) ;
#117261=SHAPE_REPRESENTATION('',(#55046),#117169) ;
#117262=PRODUCT_DEFINITION_CONTEXT('part definition',#117330,'design') ;
#117284=PRODUCT_DEFINITION('Knob_Pin','Knob_Pin',#117306,#117262) ;
#117306=PRODUCT_DEFINITION_FORMATION('',$,#117353) ;
#117330=APPLICATION_CONTEXT(
'Core Data for Automotive Mechanical Design Process') ;
#117331=PRODUCT_CONTEXT('part definition',#117330,'mechanical') ;
#117353=PRODUCT('Knob_Pin','Knob_Pin',$,(#117331)) ;
#117355=PRESENTATION_STYLE_ASSIGNMENT((#117357)) ;
#117357=SURFACE_STYLE_USAGE(.BOTH.,#117359) ;
#117359=SURFACE_SIDE_STYLE('',(#117361)) ;
#117361=SURFACE_STYLE_FILL_AREA(#117363) ;
#117363=FILL_AREA_STYLE('Opaque(160,160,160)',(#117365)) ;
#117365=FILL_AREA_STYLE_COLOUR('Opaque(160,160,160)',#117367) ;
#117367=COLOUR_RGB('Opaque(160,160,160)', 0.09019608, 0.27058824, 0.51372549) ;
ENDSEC;
END-ISO-10303-21;
